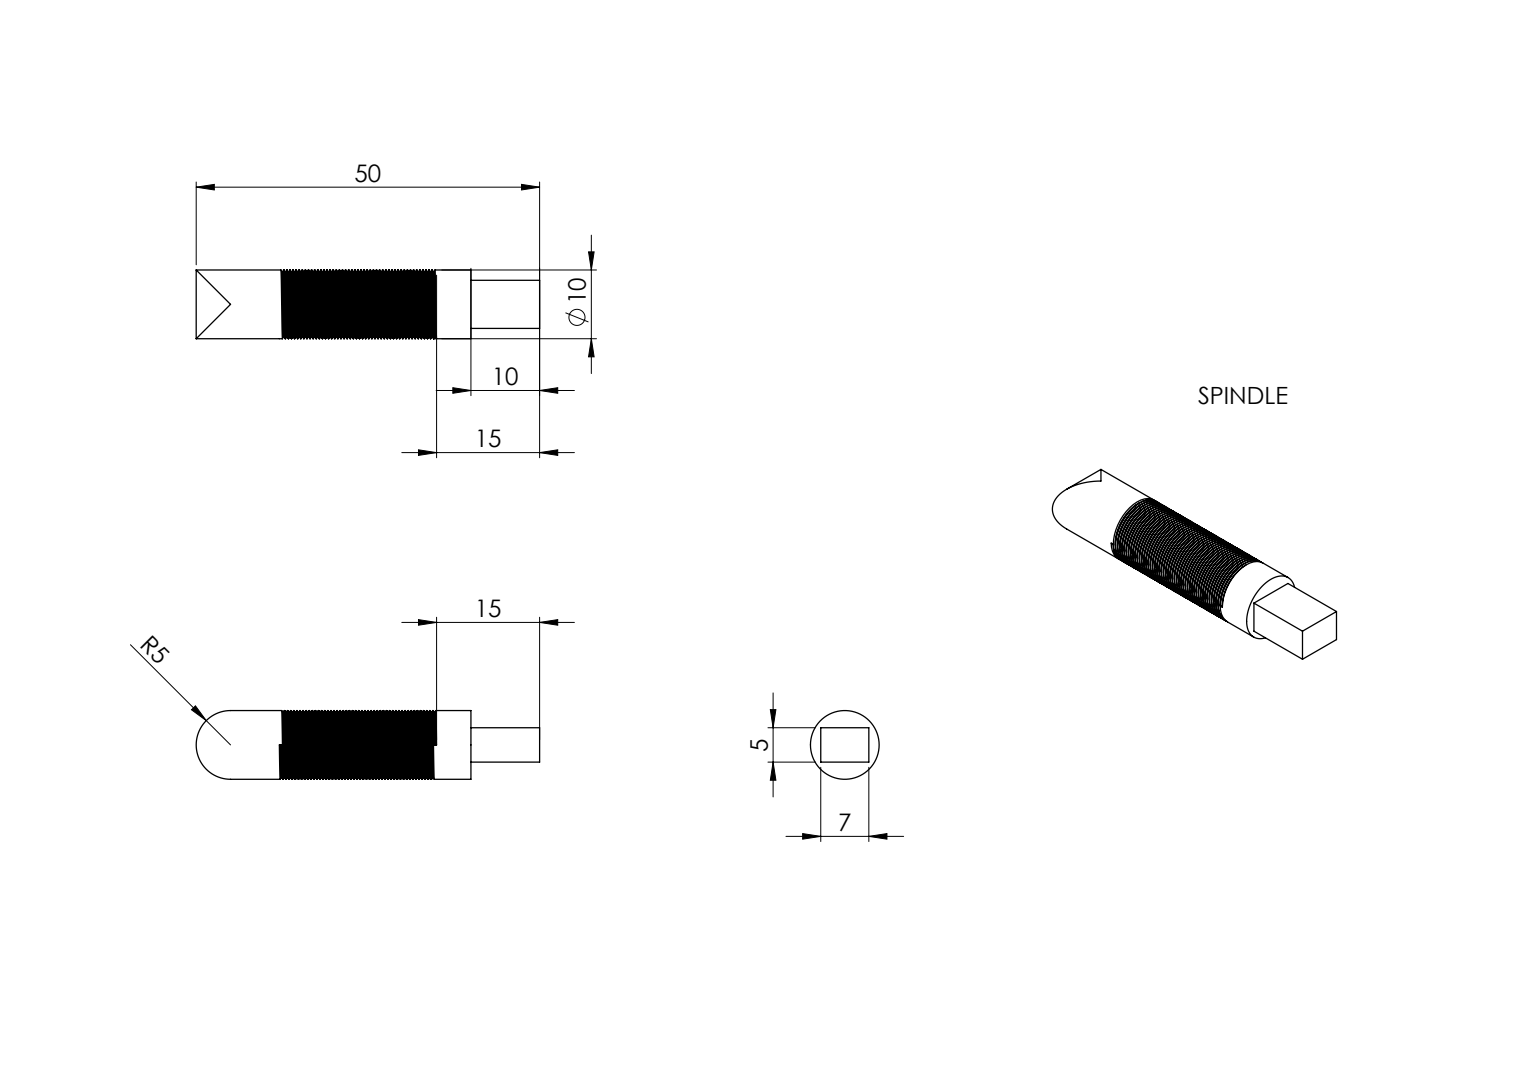
ISO-10303-21;
HEADER;
FILE_DESCRIPTION (('STEP AP214'),
    '1' );
FILE_NAME ('spindle.step',
    '2026-10-26T05:42:23',
    ( '' ),
    ( '' ),
    'SwSTEP 2.0',
    'SolidWorks 2026',
    '' );
FILE_SCHEMA (( 'AUTOMOTIVE_DESIGN' ));
ENDSEC;

DATA;
#7=CARTESIAN_POINT ( 'NONE',  ( 45.00000000000000000, 0.000000000000000000, 0.000000000000000000 ) ) ;
#9=CARTESIAN_POINT ( 'NONE',  ( 19.58437500061451786, -2.746126346562642428, -4.756430356249999214 ) ) ;
#12=CARTESIAN_POINT ( 'NONE',  ( 15.13125000122903252, 4.330127018922191873, 2.499999999999999556 ) ) ;
#27=CARTESIAN_POINT ( 'NONE',  ( 7.396875000614516082, -4.119189519843965641, -2.378215178125001383 ) ) ;
#49=CARTESIAN_POINT ( 'NONE',  ( 13.88437500061451679, 5.824947211148865298E-16, -4.756430356249998326 ) ) ;
#74=EDGE_CURVE ( 'NONE', #45106, #54880, #1431, .T. ) ;
#80=CARTESIAN_POINT ( 'NONE',  ( 19.88437500061451857, 4.119189519843966529, 2.378215178124999607 ) ) ;
#85=CARTESIAN_POINT ( 'NONE',  ( 19.46249999999999858, 2.886751345948129099, -4.999999999999998224 ) ) ;
#89=CARTESIAN_POINT ( 'NONE',  ( 24.45937500061451786, -5.492252693125287522, -1.008910452111647106E-15 ) ) ;
#95=CARTESIAN_POINT ( 'NONE',  ( 27.64687500061451431, -4.119189519843965641, -2.378215178125001383 ) ) ;
#97=CARTESIAN_POINT ( 'NONE',  ( 11.07187500061451679, 5.824947211148865298E-16, -4.756430356249998326 ) ) ;
#104=( BOUNDED_CURVE ( )  B_SPLINE_CURVE ( 2, ( #27084, #21157, #20050, #59212, #14521, #42242, #3825 ),
 .UNSPECIFIED., .F., .F. ) 
 B_SPLINE_CURVE_WITH_KNOTS ( ( 3, 2, 2, 3 ),
 ( 0.5700000000000000622, 0.5733333333333334725, 0.5766666666666667718, 0.5800000000000000711 ),
 .UNSPECIFIED. ) 
 CURVE ( )  GEOMETRIC_REPRESENTATION_ITEM ( )  RATIONAL_B_SPLINE_CURVE ( ( 0.9999999999999955591, 0.8660254037844431485, 1.000000000000000000, 0.8660254037844387076, 1.000000000000000000, 0.8660254037844342667, 1.000000000000004441 ) ) 
 REPRESENTATION_ITEM ( '' )  );
#108=CARTESIAN_POINT ( 'NONE',  ( 18.67500000000000071, 4.330127018922191873, 2.499999999999999556 ) ) ;
#123=ORIENTED_EDGE ( 'NONE', *, *, #29254, .F. ) ;
#133=CARTESIAN_POINT ( 'NONE',  ( 22.35937500061451644, -4.119189519843965641, -2.378215178125001383 ) ) ;
#139=ORIENTED_EDGE ( 'NONE', *, *, #5292, .F. ) ;
#151=CARTESIAN_POINT ( 'NONE',  ( 17.30625000122903145, 4.330127018922192761, -2.499999999999997780 ) ) ;
#163=EDGE_CURVE ( 'NONE', #39643, #7983, #64627, .T. ) ;
#168=CARTESIAN_POINT ( 'NONE',  ( 26.67187500061451644, 2.746126346562643317, 4.756430356249998326 ) ) ;
#173=CARTESIAN_POINT ( 'NONE',  ( 26.25000000000000000, 4.330127018922192761, -2.499999999999997780 ) ) ;
#181=CARTESIAN_POINT ( 'NONE',  ( 11.11875000122903323, 2.886751345948126879, 4.999999999999999112 ) ) ;
#182=CARTESIAN_POINT ( 'NONE',  ( 13.19999999999999929, 4.330127018922192761, -2.499999999999997780 ) ) ;
#185=CARTESIAN_POINT ( 'NONE',  ( 21.27187500061451431, -4.119189519843968306, 2.378215178124996054 ) ) ;
#192=CARTESIAN_POINT ( 'NONE',  ( 10.74375000122903323, -2.886751345948130876, 4.999999999999996447 ) ) ;
#196=CARTESIAN_POINT ( 'NONE',  ( 13.05937500061451573, 2.746126346562643317, 4.756430356249998326 ) ) ;
#203=LINE ( 'NONE', #67793, #8872 ) ;
#217=CARTESIAN_POINT ( 'NONE',  ( 13.57500000000000107, 6.123233995736764310E-16, -4.999999999999998224 ) ) ;
#219=CARTESIAN_POINT ( 'NONE',  ( 29.29687500061451644, 0.000000000000000000, 4.756430356249998326 ) ) ;
#220=CARTESIAN_POINT ( 'NONE',  ( 12.38437500061451857, -4.119189519843968306, 2.378215178124996054 ) ) ;
#237=CARTESIAN_POINT ( 'NONE',  ( 23.26875000122903003, 2.886751345948126879, 4.999999999999999112 ) ) ;
#282=CARTESIAN_POINT ( 'NONE',  ( 17.89687500061451431, 4.119189519843966529, -2.378215178124998275 ) ) ;
#297=CARTESIAN_POINT ( 'NONE',  ( 18.22499999999999787, 4.330127018922191873, 2.499999999999999556 ) ) ;
#298=CARTESIAN_POINT ( 'NONE',  ( 19.05937500061451928, 0.000000000000000000, 4.756430356249998326 ) ) ;
#308=EDGE_LOOP ( 'NONE', ( #45837, #56679, #50706, #57678 ) ) ;
#339=AXIS2_PLACEMENT_3D ( 'NONE', #22340, #45247, #39713 ) ;
#342=CARTESIAN_POINT ( 'NONE',  ( 9.946875000614516793, 5.492252693125287522, 3.363034840372157021E-16 ) ) ;
#360=CARTESIAN_POINT ( 'NONE',  ( 18.38437500061451502, 5.492252693125287522, 3.363034840372157021E-16 ) ) ;
#363=CARTESIAN_POINT ( 'NONE',  ( 26.67187500061451289, -4.119189519843968306, 2.378215178124996054 ) ) ;
#371=FACE_OUTER_BOUND ( 'NONE', #14066, .T. ) ;
#377=CARTESIAN_POINT ( 'NONE',  ( 7.696875000614517681, 0.000000000000000000, 4.756430356249998326 ) ) ;
#384=CARTESIAN_POINT ( 'NONE',  ( 24.84375000122903288, -2.886751345948153968, -4.999999999999952038 ) ) ;
#386=CARTESIAN_POINT ( 'NONE',  ( 11.38125000122903252, 6.123233995736764310E-16, -4.999999999999998224 ) ) ;
#399=CARTESIAN_POINT ( 'NONE',  ( 15.08437500061451786, -4.119189519843968306, 2.378215178124996054 ) ) ;
#430=CARTESIAN_POINT ( 'NONE',  ( 17.37187500061451573, -5.492252693125287522, -1.008910452111647106E-15 ) ) ;
#432=CARTESIAN_POINT ( 'NONE',  ( 14.53125000122903288, 6.123233995736764310E-16, -4.999999999999998224 ) ) ;
#437=CARTESIAN_POINT ( 'NONE',  ( 18.67500000000000071, 4.330127018922191873, 2.499999999999999556 ) ) ;
#441=CARTESIAN_POINT ( 'NONE',  ( 26.14687500061451431, 0.000000000000000000, 4.756430356249998326 ) ) ;
#442=CARTESIAN_POINT ( 'NONE',  ( 18.39375000122902648, -2.886751345948074920, 5.000000000000092371 ) ) ;
#449=CARTESIAN_POINT ( 'NONE',  ( 25.02187500061451431, 5.824947211148865298E-16, -4.756430356249998326 ) ) ;
#451=CARTESIAN_POINT ( 'NONE',  ( 11.10937500061451644, 2.746126346562645981, -4.756430356249997438 ) ) ;
#454=ORIENTED_EDGE ( 'NONE', *, *, #66600, .F. ) ;
#456=CARTESIAN_POINT ( 'NONE',  ( 45.00000000000000000, 6.123233995736764310E-16, -4.999999999999998224 ) ) ;
#457=CARTESIAN_POINT ( 'NONE',  ( 17.00625000122903074, 0.000000000000000000, 4.999999999999998224 ) ) ;
#461=CYLINDRICAL_SURFACE ( 'NONE', #51393, 4.999999999999998224 ) ;
#465=CARTESIAN_POINT ( 'NONE',  ( 13.69687500061451679, -4.119189519843965641, -2.378215178125001383 ) ) ;
#475=CARTESIAN_POINT ( 'NONE',  ( 18.86249999999999716, -5.773502691896255534, -1.060575238724906372E-15 ) ) ;
#485=CARTESIAN_POINT ( 'NONE',  ( 21.53437500061451715, 5.824947211148865298E-16, -4.756430356249998326 ) ) ;
#489=( BOUNDED_CURVE ( )  B_SPLINE_CURVE ( 2, ( #20921, #14646, #9118, #48647, #21286, #33107, #71172 ),
 .UNSPECIFIED., .F., .F. ) 
 B_SPLINE_CURVE_WITH_KNOTS ( ( 3, 2, 2, 3 ),
 ( 0.3500000000000000888, 0.3533333333333333881, 0.3566666666666667429, 0.3599999999999999867 ),
 .UNSPECIFIED. ) 
 CURVE ( )  GEOMETRIC_REPRESENTATION_ITEM ( )  RATIONAL_B_SPLINE_CURVE ( ( 0.9999999999999955591, 0.8660254037844431485, 1.000000000000000000, 0.8660254037844387076, 1.000000000000000000, 0.8660254037844387076, 1.000000000000000000 ) ) 
 REPRESENTATION_ITEM ( '' )  );
#507=CARTESIAN_POINT ( 'NONE',  ( 16.66875000122903216, -5.773502691896255534, -1.060575238724906372E-15 ) ) ;
#509=CARTESIAN_POINT ( 'NONE',  ( 29.67656250092177217, 0.000000000000000000, 4.878215178124998275 ) ) ;
#523=CARTESIAN_POINT ( 'NONE',  ( 25.32187500061451857, 2.746126346562643317, 4.756430356249998326 ) ) ;
#528=CARTESIAN_POINT ( 'NONE',  ( 26.17500000000000071, 6.123233995736764310E-16, -4.999999999999998224 ) ) ;
#538=CARTESIAN_POINT ( 'NONE',  ( 9.431250001229033231, -4.330127018922194537, 2.499999999999995559 ) ) ;
#542=CARTESIAN_POINT ( 'NONE',  ( 18.87187500061451573, 4.119189519843966529, 2.378215178124999607 ) ) ;
#555=CARTESIAN_POINT ( 'NONE',  ( 13.13437500061451679, -2.746126346562646425, 4.756430356249996549 ) ) ;
#579=CARTESIAN_POINT ( 'NONE',  ( 28.88437500061451502, 4.119189519843966529, 2.378215178124999607 ) ) ;
#583=CARTESIAN_POINT ( 'NONE',  ( 11.67187500061451821, 2.746126346562645981, -4.756430356249997438 ) ) ;
#593=( BOUNDED_CURVE ( )  B_SPLINE_CURVE ( 2, ( #12661, #29655, #35196, #35914, #62904, #56997, #24104 ),
 .UNSPECIFIED., .F., .F. ) 
 B_SPLINE_CURVE_WITH_KNOTS ( ( 3, 2, 2, 3 ),
 ( 0.8600000000000002087, 0.8633333333333333970, 0.8666666666666668073, 0.8699999999999999956 ),
 .UNSPECIFIED. ) 
 CURVE ( )  GEOMETRIC_REPRESENTATION_ITEM ( )  RATIONAL_B_SPLINE_CURVE ( ( 0.9999999999999911182, 0.8660254037844475894, 1.000000000000000000, 0.8660254037844387076, 1.000000000000000000, 0.8660254037844387076, 1.000000000000000000 ) ) 
 REPRESENTATION_ITEM ( '' )  );
#600=CARTESIAN_POINT ( 'NONE',  ( 22.36875000122903145, 2.886751345948126879, 4.999999999999999112 ) ) ;
#607=CARTESIAN_POINT ( 'NONE',  ( 25.55625000122903501, 0.000000000000000000, 4.999999999999998224 ) ) ;
#647=CARTESIAN_POINT ( 'NONE',  ( 18.12187500061451928, -4.119189519843968306, 2.378215178124996054 ) ) ;
#662=CARTESIAN_POINT ( 'NONE',  ( 22.12500000000000000, 6.123233995736764310E-16, -4.999999999999998224 ) ) ;
#663=CARTESIAN_POINT ( 'NONE',  ( 20.85937500061451644, 0.000000000000000000, 4.756430356249998326 ) ) ;
#675=VERTEX_POINT ( 'NONE', #2077 ) ;
#706=AXIS2_PLACEMENT_3D ( 'NONE', #6791, #31874, #14139 ) ;
#707=CARTESIAN_POINT ( 'NONE',  ( 9.834375000614517859, 5.824947211148865298E-16, -4.756430356249998326 ) ) ;
#729=CARTESIAN_POINT ( 'NONE',  ( 18.23437500061451644, -2.746126346562642428, -4.756430356249999214 ) ) ;
#732=CARTESIAN_POINT ( 'NONE',  ( 24.98437500061451289, -2.746126346562642428, -4.756430356249999214 ) ) ;
#736=CARTESIAN_POINT ( 'NONE',  ( 28.72500000000000142, -4.330127018922194537, 2.499999999999995559 ) ) ;
#746=CARTESIAN_POINT ( 'NONE',  ( 26.14687500061451431, 5.492252693125287522, 3.363034840372157021E-16 ) ) ;
#765=CARTESIAN_POINT ( 'NONE',  ( 15.19687500061451679, -2.746126346562641984, -4.756430356249999214 ) ) ;
#780=ORIENTED_EDGE ( 'NONE', *, *, #27131, .T. ) ;
#797=CARTESIAN_POINT ( 'NONE',  ( 17.29687500061451999, -2.746126346562646425, 4.756430356249996549 ) ) ;
#805=CARTESIAN_POINT ( 'NONE',  ( 16.35000000000000142, 4.330127018922192761, -2.499999999999997780 ) ) ;
#809=CARTESIAN_POINT ( 'NONE',  ( 26.52187500061451431, 4.119189519843966529, 2.378215178124999607 ) ) ;
#816=CARTESIAN_POINT ( 'NONE',  ( 23.85937500061451644, 2.746126346562643317, 4.756430356249998326 ) ) ;
#818=CARTESIAN_POINT ( 'NONE',  ( 10.32187500061451679, 4.119189519843966529, 2.378215178124999607 ) ) ;
#821=ORIENTED_EDGE ( 'NONE', *, *, #39594, .T. ) ;
#823=CARTESIAN_POINT ( 'NONE',  ( 16.72500000000000142, 6.123233995736764310E-16, -4.999999999999998224 ) ) ;
#827=CARTESIAN_POINT ( 'NONE',  ( 29.55000000000000071, 0.000000000000000000, 4.999999999999998224 ) ) ;
#829=VERTEX_POINT ( 'NONE', #12152 ) ;
#831=CARTESIAN_POINT ( 'NONE',  ( 11.82187500061451502, -4.119189519843968306, 2.378215178124996054 ) ) ;
#851=VECTOR ( 'NONE', #69149, 1000.000000000000000 ) ;
#853=CARTESIAN_POINT ( 'NONE',  ( 21.38437500061451502, -4.119189519843968306, 2.378215178124996054 ) ) ;
#865=CARTESIAN_POINT ( 'NONE',  ( 15.05625000122903323, 4.330127018922192761, -2.499999999999997780 ) ) ;
#873=CARTESIAN_POINT ( 'NONE',  ( 16.59375000122903288, -2.886751345948129988, 4.999999999999997335 ) ) ;
#889=CARTESIAN_POINT ( 'NONE',  ( 24.60937500061451644, -4.119189519843965641, -2.378215178125001383 ) ) ;
#893=EDGE_CURVE ( 'NONE', #53197, #52280, #67237, .T. ) ;
#895=CARTESIAN_POINT ( 'NONE',  ( 23.96249999999999858, 2.886751345948129099, -4.999999999999998224 ) ) ;
#902=CARTESIAN_POINT ( 'NONE',  ( 22.96875000122903288, -5.773502691896255534, -1.060575238724906372E-15 ) ) ;
#904=CARTESIAN_POINT ( 'NONE',  ( 9.993750001229033231, -2.886751345948125991, -5.000000000000000000 ) ) ;
#905=CARTESIAN_POINT ( 'NONE',  ( 9.037499999999997868, -2.886751345948181946, -4.999999999999904077 ) ) ;
#908=CARTESIAN_POINT ( 'NONE',  ( 19.39687500061451786, 0.000000000000000000, 4.756430356249998326 ) ) ;
#911=ORIENTED_EDGE ( 'NONE', *, *, #71191, .F. ) ;
#912=CARTESIAN_POINT ( 'NONE',  ( 27.52500000000000213, 6.123233995736764310E-16, -4.999999999999998224 ) ) ;
#919=CARTESIAN_POINT ( 'NONE',  ( 10.20937500061451608, 2.746126346562645981, -4.756430356249997438 ) ) ;
#922=( BOUNDED_CURVE ( )  B_SPLINE_CURVE ( 2, ( #607, #7219, #22752, #18276, #6498, #23113, #45303 ),
 .UNSPECIFIED., .F., .F. ) 
 B_SPLINE_CURVE_WITH_KNOTS ( ( 3, 2, 2, 3 ),
 ( 0.1799999999999999378, 0.1833333333333333204, 0.1866666666666667029, 0.1900000000000000855 ),
 .UNSPECIFIED. ) 
 CURVE ( )  GEOMETRIC_REPRESENTATION_ITEM ( )  RATIONAL_B_SPLINE_CURVE ( ( 1.000000000000002220, 0.8660254037844364872, 1.000000000000000000, 0.8660254037844387076, 1.000000000000000000, 0.8660254037844353769, 1.000000000000003331 ) ) 
 REPRESENTATION_ITEM ( '' )  );
#938=ADVANCED_FACE ( 'NONE', ( #56138 ), #34679, .T. ) ;
#942=CARTESIAN_POINT ( 'NONE',  ( 28.54687500061451644, -2.746126346562646425, 4.756430356249996549 ) ) ;
#945=CARTESIAN_POINT ( 'NONE',  ( 27.64687500061451431, -4.119189519843965641, -2.378215178125001383 ) ) ;
#946=CARTESIAN_POINT ( 'NONE',  ( 12.45937500061451786, -4.119189519843965641, -2.378215178125001383 ) ) ;
#961=CARTESIAN_POINT ( 'NONE',  ( 22.51875000122903003, -5.773502691896255534, -1.060575238724906372E-15 ) ) ;
#987=FACE_OUTER_BOUND ( 'NONE', #13837, .T. ) ;
#996=CARTESIAN_POINT ( 'NONE',  ( 19.14375000122903003, 5.773502691896255534, 3.535250795749688401E-16 ) ) ;
#1007=ORIENTED_EDGE ( 'NONE', *, *, #23321, .F. ) ;
#1010=CARTESIAN_POINT ( 'NONE',  ( 19.80937500061451217, 2.746126346562643317, 4.756430356249998326 ) ) ;
#1012=( BOUNDED_CURVE ( )  B_SPLINE_CURVE ( 2, ( #8240, #47399, #2701, #60291, #65115, #64749, #48503 ),
 .UNSPECIFIED., .F., .F. ) 
 B_SPLINE_CURVE_WITH_KNOTS ( ( 3, 2, 2, 3 ),
 ( 0.4799999999999999267, 0.4833333333333333370, 0.4866666666666667473, 0.4900000000000001021 ),
 .UNSPECIFIED. ) 
 CURVE ( )  GEOMETRIC_REPRESENTATION_ITEM ( )  RATIONAL_B_SPLINE_CURVE ( ( 1.000000000000002220, 0.8660254037844364872, 1.000000000000000000, 0.8660254037844387076, 1.000000000000000000, 0.8660254037844342667, 1.000000000000004441 ) ) 
 REPRESENTATION_ITEM ( '' )  );
#1027=CARTESIAN_POINT ( 'NONE',  ( 22.19999999999999574, 4.330127018922192761, -2.499999999999997780 ) ) ;
#1028=CARTESIAN_POINT ( 'NONE',  ( 20.40937500061451715, 0.000000000000000000, 4.756430356249998326 ) ) ;
#1045=CARTESIAN_POINT ( 'NONE',  ( 29.60625000122903216, 0.000000000000000000, 4.999999999999998224 ) ) ;
#1049=CARTESIAN_POINT ( 'NONE',  ( 8.521875000614517859, 2.746126346562645981, -4.756430356249997438 ) ) ;
#1055=EDGE_CURVE ( 'NONE', #42390, #54979, #24487, .T. ) ;
#1067=EDGE_CURVE ( 'NONE', #56470, #45665, #34410, .T. ) ;
#1074=CARTESIAN_POINT ( 'NONE',  ( 8.709375000614517859, 0.000000000000000000, 4.756430356249998326 ) ) ;
#1083=CARTESIAN_POINT ( 'NONE',  ( 23.98125000122903216, 6.123233995736764310E-16, -4.999999999999998224 ) ) ;
#1094=CARTESIAN_POINT ( 'NONE',  ( 16.77187500061451431, -4.119189519843968306, 2.378215178124996054 ) ) ;
#1097=CARTESIAN_POINT ( 'NONE',  ( 27.27187500061451786, 5.824947211148865298E-16, -4.756430356249998326 ) ) ;
#1101=DIRECTION ( 'NONE',  ( -1.000000000000000000, -0.000000000000000000, -0.000000000000000000 ) ) ;
#1104=CARTESIAN_POINT ( 'NONE',  ( 28.25625000122903074, 0.000000000000000000, 4.999999999999998224 ) ) ;
#1105=CARTESIAN_POINT ( 'NONE',  ( 45.00000000000000000, 0.000000000000000000, 0.000000000000000000 ) ) ;
#1111=CARTESIAN_POINT ( 'NONE',  ( 27.60937500061451644, 0.000000000000000000, 4.756430356249998326 ) ) ;
#1128=CARTESIAN_POINT ( 'NONE',  ( 15.42187500061451821, 2.746126346562643317, 4.756430356249998326 ) ) ;
#1145=EDGE_CURVE ( 'NONE', #65176, #58120, #30504, .T. ) ;
#1155=EDGE_LOOP ( 'NONE', ( #2010, #4569, #25849, #38019 ) ) ;
#1159=CARTESIAN_POINT ( 'NONE',  ( 17.48437500061451999, 5.824947211148865298E-16, -4.756430356249998326 ) ) ;
#1165=CARTESIAN_POINT ( 'NONE',  ( 17.02499999999999858, -4.330127018922194537, 2.499999999999995559 ) ) ;
#1168=DIRECTION ( 'NONE',  ( -1.000000000000000000, -0.000000000000000000, -0.000000000000000000 ) ) ;
#1169=CARTESIAN_POINT ( 'NONE',  ( 24.08437500061451786, -2.746126346562641984, -4.756430356249999214 ) ) ;
#1172=DIRECTION ( 'NONE',  ( 0.000000000000000000, -0.000000000000000000, -1.000000000000000000 ) ) ;
#1176=CARTESIAN_POINT ( 'NONE',  ( 25.77187500061451431, -4.119189519843968306, 2.378215178124996054 ) ) ;
#1178=CARTESIAN_POINT ( 'NONE',  ( 11.40937500061451537, -5.492252693125287522, -1.008910452111647106E-15 ) ) ;
#1186=CARTESIAN_POINT ( 'NONE',  ( 19.31250000000000000, -5.773502691896255534, -1.060575238724906372E-15 ) ) ;
#1187=FACE_OUTER_BOUND ( 'NONE', #70804, .T. ) ;
#1188=ORIENTED_EDGE ( 'NONE', *, *, #50906, .T. ) ;
#1190=CARTESIAN_POINT ( 'NONE',  ( 10.88437500061451679, -2.746126346562646425, 4.756430356249996549 ) ) ;
#1203=ORIENTED_EDGE ( 'NONE', *, *, #11547, .T. ) ;
#1211=CARTESIAN_POINT ( 'NONE',  ( 22.62187500061451573, 2.746126346562643317, 4.756430356249998326 ) ) ;
#1228=CARTESIAN_POINT ( 'NONE',  ( 28.61250000000000071, 2.886751345948148195, 4.999999999999962697 ) ) ;
#1231=CARTESIAN_POINT ( 'NONE',  ( 17.41875000122903216, 2.886751345948126879, 4.999999999999999112 ) ) ;
#1248=CARTESIAN_POINT ( 'NONE',  ( 23.48437500061451644, 4.119189519843966529, 2.378215178124999607 ) ) ;
#1254=CARTESIAN_POINT ( 'NONE',  ( 25.08749999999999858, -2.886751345948129988, 4.999999999999997335 ) ) ;
#1258=CARTESIAN_POINT ( 'NONE',  ( 24.41250000000000142, 2.886751345948142866, -4.999999999999973355 ) ) ;
#1262=CARTESIAN_POINT ( 'NONE',  ( 8.493750001229033231, -2.886751345948129988, 4.999999999999997335 ) ) ;
#1265=CARTESIAN_POINT ( 'NONE',  ( 17.74687500061451928, -4.119189519843965641, -2.378215178125001383 ) ) ;
#1274=CARTESIAN_POINT ( 'NONE',  ( 16.55625000122903145, 0.000000000000000000, 4.999999999999998224 ) ) ;
#1275=CARTESIAN_POINT ( 'NONE',  ( 11.03437500061451360, -2.746126346562642428, -4.756430356249999214 ) ) ;
#1288=CARTESIAN_POINT ( 'NONE',  ( 9.637499999999999289, 5.773502691896255534, 3.535250795749688894E-16 ) ) ;
#1297=CARTESIAN_POINT ( 'NONE',  ( 29.55937500061451573, -4.119189519843965641, -2.378215178125001383 ) ) ;
#1299=CARTESIAN_POINT ( 'NONE',  ( 28.65937500061451715, 2.746126346562645981, -4.756430356249997438 ) ) ;
#1300=CARTESIAN_POINT ( 'NONE',  ( 13.69687500061451679, -2.746126346562646425, 4.756430356249996549 ) ) ;
#1308=DIRECTION ( 'NONE',  ( -1.000000000000000000, -0.000000000000000000, -0.000000000000000000 ) ) ;
#1317=CARTESIAN_POINT ( 'NONE',  ( 22.93125000122903145, -4.330127018922194537, 2.499999999999995559 ) ) ;
#1342=DIRECTION ( 'NONE',  ( 0.000000000000000000, 0.000000000000000000, -1.000000000000000000 ) ) ;
#1343=ADVANCED_FACE ( 'NONE', ( #50096 ), #44567, .T. ) ;
#1345=ADVANCED_FACE ( 'NONE', ( #26702 ), #38510, .T. ) ;
#1353=CARTESIAN_POINT ( 'NONE',  ( 19.10625000122903216, 4.330127018922192761, -2.499999999999997780 ) ) ;
#1361=CARTESIAN_POINT ( 'NONE',  ( 11.10000000000000142, 0.000000000000000000, 4.999999999999998224 ) ) ;
#1370=CARTESIAN_POINT ( 'NONE',  ( 18.27187500061451431, 5.824947211148865298E-16, -4.756430356249998326 ) ) ;
#1379=ORIENTED_EDGE ( 'NONE', *, *, #49066, .T. ) ;
#1386=( GEOMETRIC_REPRESENTATION_CONTEXT ( 3 ) GLOBAL_UNCERTAINTY_ASSIGNED_CONTEXT ( ( #63913 ) ) GLOBAL_UNIT_ASSIGNED_CONTEXT ( ( #46737, #57797, #30097 ) ) REPRESENTATION_CONTEXT ( 'NONE', 'WORKASPACE' ) );
#1387=CARTESIAN_POINT ( 'NONE',  ( 22.31250000000000000, 2.886751345948154857, 4.999999999999951150 ) ) ;
#1388=CARTESIAN_POINT ( 'NONE',  ( 20.67187500061451289, 2.746126346562645981, -4.756430356249997438 ) ) ;
#1411=DIRECTION ( 'NONE',  ( -1.000000000000000000, -0.000000000000000000, -0.000000000000000000 ) ) ;
#1431=( BOUNDED_CURVE ( )  B_SPLINE_CURVE ( 2, ( #52853, #2977, #53211, #8514, #2607, #25129, #47670 ),
 .UNSPECIFIED., .F., .T. ) 
 B_SPLINE_CURVE_WITH_KNOTS ( ( 3, 2, 2, 3 ),
 ( 0.6300000000000001155, 0.6333333333333334147, 0.6366666666666668251, 0.6400000000000001243 ),
 .UNSPECIFIED. ) 
 CURVE ( )  GEOMETRIC_REPRESENTATION_ITEM ( )  RATIONAL_B_SPLINE_CURVE ( ( 0.9999999999999955591, 0.8660254037844431485, 1.000000000000000000, 0.8660254037844387076, 1.000000000000000000, 0.8660254037844342667, 1.000000000000004441 ) ) 
 REPRESENTATION_ITEM ( '' )  );
#1434=CARTESIAN_POINT ( 'NONE',  ( 8.934375000614517504, 5.824947211148865298E-16, -4.756430356249998326 ) ) ;
#1440=EDGE_CURVE ( 'NONE', #59687, #30573, #41969, .T. ) ;
#1455=CARTESIAN_POINT ( 'NONE',  ( 17.85937500061451644, 2.746126346562645981, -4.756430356249997438 ) ) ;
#1458=CARTESIAN_POINT ( 'NONE',  ( 26.29687500061451644, -4.119189519843965641, -2.378215178125001383 ) ) ;
#1473=CARTESIAN_POINT ( 'NONE',  ( 27.83437500061451786, 5.824947211148865298E-16, -4.756430356249998326 ) ) ;
#1482=VERTEX_POINT ( 'NONE', #21504 ) ;
#1492=CARTESIAN_POINT ( 'NONE',  ( 14.59687500061452070, -2.746126346562646425, 4.756430356249996549 ) ) ;
#1518=VERTEX_POINT ( 'NONE', #4538 ) ;
#1522=CARTESIAN_POINT ( 'NONE',  ( 15.64687500061451608, -2.746126346562642428, -4.756430356249999214 ) ) ;
#1528=CARTESIAN_POINT ( 'NONE',  ( 18.26249999999999929, 2.886751345948126879, 4.999999999999999112 ) ) ;
#1531=CARTESIAN_POINT ( 'NONE',  ( 45.00000000000000000, 6.123233995736764310E-16, -4.999999999999998224 ) ) ;
#1532=CARTESIAN_POINT ( 'NONE',  ( 24.38437500061451502, -2.746126346562646425, 4.756430356249996549 ) ) ;
#1535=CARTESIAN_POINT ( 'NONE',  ( 45.00000000000000000, 0.000000000000000000, 4.999999999999998224 ) ) ;
#1539=CARTESIAN_POINT ( 'NONE',  ( 25.47187500061451360, 5.824947211148865298E-16, -4.756430356249998326 ) ) ;
#1541=CARTESIAN_POINT ( 'NONE',  ( 10.50937500061451502, -5.492252693125287522, -1.008910452111647106E-15 ) ) ;
#1546=DIRECTION ( 'NONE',  ( 0.000000000000000000, 0.000000000000000000, 1.000000000000000000 ) ) ;
#1550=CARTESIAN_POINT ( 'NONE',  ( 12.28125000122903110, 6.123233995736764310E-16, -4.999999999999998224 ) ) ;
#1553=CARTESIAN_POINT ( 'NONE',  ( 12.19687500061451502, 0.000000000000000000, 4.756430356249998326 ) ) ;
#1565=VERTEX_POINT ( 'NONE', #65849 ) ;
#1573=CARTESIAN_POINT ( 'NONE',  ( 21.83437500061451786, -4.119189519843968306, 2.378215178124996054 ) ) ;
#1580=VERTEX_POINT ( 'NONE', #26328 ) ;
#1590=CARTESIAN_POINT ( 'NONE',  ( 21.41250000000000142, 2.886751345948126879, 4.999999999999998224 ) ) ;
#1607=CARTESIAN_POINT ( 'NONE',  ( 24.30937500061451573, 4.119189519843966529, -2.378215178124998275 ) ) ;
#1611=EDGE_CURVE ( 'NONE', #33907, #61284, #66577, .T. ) ;
#1614=CARTESIAN_POINT ( 'NONE',  ( 25.05000000000000071, 0.000000000000000000, 4.999999999999998224 ) ) ;
#1618=DIRECTION ( 'NONE',  ( 0.000000000000000000, 1.000000000000000000, -8.673617379884037937E-17 ) ) ;
#1624=CARTESIAN_POINT ( 'NONE',  ( 15.29999999999999893, -4.330127018922190985, -2.500000000000001332 ) ) ;
#1626=CARTESIAN_POINT ( 'NONE',  ( 8.381250001229034297, 4.330127018922191873, 2.499999999999999556 ) ) ;
#1629=CARTESIAN_POINT ( 'NONE',  ( 17.48437500061451644, 5.492252693125287522, 3.363034840372157021E-16 ) ) ;
#1636=EDGE_CURVE ( 'NONE', #53798, #61419, #18855, .T. ) ;
#1641=CARTESIAN_POINT ( 'NONE',  ( 9.984375000614516438, -2.746126346562646425, 4.756430356249996549 ) ) ;
#1642=ORIENTED_EDGE ( 'NONE', *, *, #4558, .T. ) ;
#1649=CARTESIAN_POINT ( 'NONE',  ( 28.48125000122902861, 6.123233995736764310E-16, -4.999999999999998224 ) ) ;
#1653=CARTESIAN_POINT ( 'NONE',  ( 10.01250000000000107, 2.886751345948129099, -4.999999999999998224 ) ) ;
#1656=VERTEX_POINT ( 'NONE', #44433 ) ;
#1663=CARTESIAN_POINT ( 'NONE',  ( 26.97187500061451360, 4.119189519843966529, 2.378215178124999607 ) ) ;
#1664=CARTESIAN_POINT ( 'NONE',  ( 13.84687500061451537, -2.746126346562642428, -4.756430356249999214 ) ) ;
#1679=CARTESIAN_POINT ( 'NONE',  ( 23.75625000122903074, 0.000000000000000000, 4.999999999999998224 ) ) ;
#1702=CARTESIAN_POINT ( 'NONE',  ( 25.42500000000000071, 4.330127018922191873, 2.499999999999999556 ) ) ;
#1717=CARTESIAN_POINT ( 'NONE',  ( 45.00000000000000000, 0.000000000000000000, 0.000000000000000000 ) ) ;
#1724=VERTEX_POINT ( 'NONE', #60289 ) ;
#1730=CARTESIAN_POINT ( 'NONE',  ( 19.43437500061451573, -2.746126346562646425, 4.756430356249996549 ) ) ;
#1743=EDGE_CURVE ( 'NONE', #59457, #65810, #46732, .T. ) ;
#1749=CARTESIAN_POINT ( 'NONE',  ( 19.39687500061451786, 5.492252693125287522, 3.363034840372157021E-16 ) ) ;
#1773=CARTESIAN_POINT ( 'NONE',  ( 7.500000000000000000, 0.000000000000000000, 4.999999999999998224 ) ) ;
#1784=VERTEX_POINT ( 'NONE', #29238 ) ;
#1785=VECTOR ( 'NONE', #34589, 1000.000000000000000 ) ;
#1797=CARTESIAN_POINT ( 'NONE',  ( 27.88125000122903074, -4.330127018922194537, 2.499999999999995559 ) ) ;
#1798=CARTESIAN_POINT ( 'NONE',  ( 9.534375000614517148, 4.119189519843966529, 2.378215178124999607 ) ) ;
#1808=DIRECTION ( 'NONE',  ( -1.000000000000000000, -0.000000000000000000, -0.000000000000000000 ) ) ;
#1809=VECTOR ( 'NONE', #70709, 1000.000000000000000 ) ;
#1818=CARTESIAN_POINT ( 'NONE',  ( 14.48437500061451644, -2.746126346562646425, 4.756430356249996549 ) ) ;
#1821=CARTESIAN_POINT ( 'NONE',  ( 25.20937500061451431, 2.746126346562643317, 4.756430356249998326 ) ) ;
#1836=CARTESIAN_POINT ( 'NONE',  ( 27.30937500061451573, -4.119189519843965641, -2.378215178125001383 ) ) ;
#1846=VERTEX_POINT ( 'NONE', #34042 ) ;
#1856=CARTESIAN_POINT ( 'NONE',  ( 11.63437500061451857, 5.824947211148865298E-16, -4.756430356249998326 ) ) ;
#1887=VECTOR ( 'NONE', #21892, 1000.000000000000000 ) ;
#1889=CARTESIAN_POINT ( 'NONE',  ( 17.55937500061451573, 4.119189519843966529, -2.378215178124998275 ) ) ;
#1896=CARTESIAN_POINT ( 'NONE',  ( 16.42500000000000071, 4.330127018922191873, 2.499999999999999556 ) ) ;
#1900=CARTESIAN_POINT ( 'NONE',  ( 22.80937500061451573, 2.746126346562645981, -4.756430356249997438 ) ) ;
#1907=CARTESIAN_POINT ( 'NONE',  ( 24.34687500061451715, 0.000000000000000000, 4.756430356249998326 ) ) ;
#1909=CARTESIAN_POINT ( 'NONE',  ( 8.521875000614517859, 4.119189519843966529, 2.378215178124999607 ) ) ;
#1921=CARTESIAN_POINT ( 'NONE',  ( 12.94687500061451502, 4.119189519843966529, -2.378215178124998275 ) ) ;
#1939=CARTESIAN_POINT ( 'NONE',  ( 19.77187500061451786, 2.746126346562645981, -4.756430356249997438 ) ) ;
#1975=CARTESIAN_POINT ( 'NONE',  ( 23.14687500061451786, -2.746126346562646425, 4.756430356249996549 ) ) ;
#1981=CARTESIAN_POINT ( 'NONE',  ( 25.83749999999999858, 5.773502691896255534, 3.535250795749688894E-16 ) ) ;
#1989=CARTESIAN_POINT ( 'NONE',  ( 9.206250001229033586, 4.330127018922192761, -2.499999999999997780 ) ) ;
#1992=CARTESIAN_POINT ( 'NONE',  ( 17.97187500061451360, 4.119189519843966529, 2.378215178124999607 ) ) ;
#2004=CARTESIAN_POINT ( 'NONE',  ( 9.909375000614517148, 2.746126346562643317, 4.756430356249998326 ) ) ;
#2010=ORIENTED_EDGE ( 'NONE', *, *, #40326, .T. ) ;
#2015=CARTESIAN_POINT ( 'NONE',  ( 27.49687500061451573, 0.000000000000000000, 4.756430356249998326 ) ) ;
#2018=CARTESIAN_POINT ( 'NONE',  ( 8.437500000000000000, -2.886751345948129988, 4.999999999999997335 ) ) ;
#2021=ORIENTED_EDGE ( 'NONE', *, *, #59244, .T. ) ;
#2026=CARTESIAN_POINT ( 'NONE',  ( 28.80937500061451573, 4.119189519843966529, -2.378215178124998275 ) ) ;
#2028=CARTESIAN_POINT ( 'NONE',  ( 28.73437500061451644, 5.492252693125287522, 3.363034840372157021E-16 ) ) ;
#2029=CARTESIAN_POINT ( 'NONE',  ( 9.571875000614518569, 2.746126346562643317, 4.756430356249998326 ) ) ;
#2043=CARTESIAN_POINT ( 'NONE',  ( 22.06875000122903074, -5.773502691896255534, -1.060575238724906372E-15 ) ) ;
#2058=CARTESIAN_POINT ( 'NONE',  ( 29.74687500061451217, 5.492252693125287522, 3.363034840372157021E-16 ) ) ;
#2068=FACE_OUTER_BOUND ( 'NONE', #6092, .T. ) ;
#2077=CARTESIAN_POINT ( 'NONE',  ( 28.25625000122903074, 0.000000000000000000, 4.999999999999998224 ) ) ;
#2080=VERTEX_POINT ( 'NONE', #36056 ) ;
#2084=LINE ( 'NONE', #13876, #33673 ) ;
#2094=CARTESIAN_POINT ( 'NONE',  ( 15.42187500061451466, -4.119189519843968306, 2.378215178124996054 ) ) ;
#2102=CARTESIAN_POINT ( 'NONE',  ( 11.49375000122903145, 5.773502691896255534, 3.535250795749688401E-16 ) ) ;
#2113=CARTESIAN_POINT ( 'NONE',  ( 18.49687500061452283, 5.492252693125287522, 3.363034840372157021E-16 ) ) ;
#2122=EDGE_CURVE ( 'NONE', #31702, #69475, #39613, .T. ) ;
#2144=EDGE_LOOP ( 'NONE', ( #2437, #31615, #54378, #3537 ) ) ;
#2156=CARTESIAN_POINT ( 'NONE',  ( 28.46249999999999858, 2.886751345948129099, -4.999999999999998224 ) ) ;
#2165=CYLINDRICAL_SURFACE ( 'NONE', #11436, 4.999999999999998224 ) ;
#2174=CARTESIAN_POINT ( 'NONE',  ( 16.47187500061451715, 5.824947211148865298E-16, -4.756430356249998326 ) ) ;
#2177=CARTESIAN_POINT ( 'NONE',  ( 23.48437500061451644, -2.746126346562646425, 4.756430356249996549 ) ) ;
#2185=CARTESIAN_POINT ( 'NONE',  ( 18.52499999999999858, 6.123233995736764310E-16, -4.999999999999998224 ) ) ;
#2192=CARTESIAN_POINT ( 'NONE',  ( 27.27187500061451431, -5.492252693125287522, -1.008910452111647106E-15 ) ) ;
#2211=CARTESIAN_POINT ( 'NONE',  ( 13.17187500061451821, 2.746126346562643317, 4.756430356249998326 ) ) ;
#2216=ADVANCED_FACE ( 'NONE', ( #14247 ), #53785, .T. ) ;
#2225=CARTESIAN_POINT ( 'NONE',  ( 21.93750000000000000, -2.886751345948130876, 4.999999999999996447 ) ) ;
#2240=CARTESIAN_POINT ( 'NONE',  ( 13.88437500061451679, 5.824947211148865298E-16, -4.756430356249998326 ) ) ;
#2246=CARTESIAN_POINT ( 'NONE',  ( 18.00000000000000355, -4.330127018922190985, -2.500000000000001332 ) ) ;
#2250=CARTESIAN_POINT ( 'NONE',  ( 23.93437500061451573, -2.746126346562646425, 4.756430356249996549 ) ) ;
#2254=CARTESIAN_POINT ( 'NONE',  ( 26.43750000000000355, -2.886751345948143310, 4.999999999999972466 ) ) ;
#2257=( BOUNDED_CURVE ( )  B_SPLINE_CURVE ( 2, ( #19511, #64956, #8081, #42435, #36883, #59401, #8810 ),
 .UNSPECIFIED., .F., .F. ) 
 B_SPLINE_CURVE_WITH_KNOTS ( ( 3, 2, 2, 3 ),
 ( 0.2600000000000000644, 0.2633333333333333637, 0.2666666666666667185, 0.2700000000000000733 ),
 .UNSPECIFIED. ) 
 CURVE ( )  GEOMETRIC_REPRESENTATION_ITEM ( )  RATIONAL_B_SPLINE_CURVE ( ( 0.9999999999999977796, 0.8660254037844409281, 1.000000000000000000, 0.8660254037844387076, 1.000000000000000000, 0.8660254037844364872, 1.000000000000002220 ) ) 
 REPRESENTATION_ITEM ( '' )  );
#2260=CARTESIAN_POINT ( 'NONE',  ( 23.52187500061451431, -4.119189519843968306, 2.378215178124996054 ) ) ;
#2262=CARTESIAN_POINT ( 'NONE',  ( 8.034375000614515372, 5.492252693125287522, 3.363034840372157021E-16 ) ) ;
#2269=EDGE_LOOP ( 'NONE', ( #54628, #66842, #1379, #38711 ) ) ;
#2271=CARTESIAN_POINT ( 'NONE',  ( 11.37187500061451573, -4.119189519843968306, 2.378215178124996054 ) ) ;
#2291=CARTESIAN_POINT ( 'NONE',  ( 19.50937500061451857, 0.000000000000000000, 4.756430356249998326 ) ) ;
#2325=CARTESIAN_POINT ( 'NONE',  ( 22.50937500061451857, 4.119189519843966529, -2.378215178124998275 ) ) ;
#2330=CARTESIAN_POINT ( 'NONE',  ( 24.07499999999999929, 4.330127018922191873, 2.499999999999999556 ) ) ;
#2335=CARTESIAN_POINT ( 'NONE',  ( 45.00000000000000000, 0.000000000000000000, 4.999999999999998224 ) ) ;
#2341=CARTESIAN_POINT ( 'NONE',  ( 28.62187500061451217, 5.824947211148865298E-16, -4.756430356249998326 ) ) ;
#2343=CARTESIAN_POINT ( 'NONE',  ( 16.17187500061451644, 4.119189519843966529, 2.378215178124999607 ) ) ;
#2355=CARTESIAN_POINT ( 'NONE',  ( 11.40937500061451360, -5.492252693125287522, -1.008910452111647106E-15 ) ) ;
#2366=CARTESIAN_POINT ( 'NONE',  ( 28.28437500061451360, 5.492252693125287522, 3.363034840372157021E-16 ) ) ;
#2369=CARTESIAN_POINT ( 'NONE',  ( 8.062500000000000000, -5.773502691896255534, -1.060575238724906372E-15 ) ) ;
#2377=CARTESIAN_POINT ( 'NONE',  ( 27.90937500061451715, 4.119189519843966529, -2.378215178124998275 ) ) ;
#2379=CARTESIAN_POINT ( 'NONE',  ( 10.54687500061451644, -2.746126346562646425, 4.756430356249996549 ) ) ;
#2394=CARTESIAN_POINT ( 'NONE',  ( 20.38125000122903430, 6.123233995736764310E-16, -4.999999999999998224 ) ) ;
#2417=CARTESIAN_POINT ( 'NONE',  ( 45.00000000000000000, 0.000000000000000000, 0.000000000000000000 ) ) ;
#2421=CARTESIAN_POINT ( 'NONE',  ( 45.00000000000000000, 6.123233995736764310E-16, -4.999999999999998224 ) ) ;
#2426=DIRECTION ( 'NONE',  ( -1.000000000000000000, -0.000000000000000000, -0.000000000000000000 ) ) ;
#2433=CARTESIAN_POINT ( 'NONE',  ( 27.58125000122903359, 6.123233995736764310E-16, -4.999999999999998224 ) ) ;
#2437=ORIENTED_EDGE ( 'NONE', *, *, #32834, .F. ) ;
#2441=CARTESIAN_POINT ( 'NONE',  ( 25.94999999999999929, 0.000000000000000000, 4.999999999999998224 ) ) ;
#2444=CARTESIAN_POINT ( 'NONE',  ( 16.09687500061451715, 4.119189519843966529, -2.378215178124998275 ) ) ;
#2452=CYLINDRICAL_SURFACE ( 'NONE', #69010, 4.999999999999998224 ) ;
#2459=CARTESIAN_POINT ( 'NONE',  ( 9.356250001229033941, 0.000000000000000000, 4.999999999999998224 ) ) ;
#2460=CARTESIAN_POINT ( 'NONE',  ( 14.13750000000000107, 5.773502691896255534, 3.535250795749688401E-16 ) ) ;
#2461=CARTESIAN_POINT ( 'NONE',  ( 45.00000000000000000, 6.123233995736764310E-16, -4.999999999999998224 ) ) ;
#2463=CARTESIAN_POINT ( 'NONE',  ( 27.35625000122903216, 0.000000000000000000, 4.999999999999998224 ) ) ;
#2464=CARTESIAN_POINT ( 'NONE',  ( 17.78437500061451715, -4.119189519843968306, 2.378215178124996054 ) ) ;
#2477=CARTESIAN_POINT ( 'NONE',  ( 13.95000000000000107, -4.330127018922190985, -2.500000000000001332 ) ) ;
#2481=CARTESIAN_POINT ( 'NONE',  ( 27.61875000122903145, 2.886751345948129099, -4.999999999999998224 ) ) ;
#2500=PRODUCT_DEFINITION ( 'UNKNOWN', '', #41496, #8500 ) ;
#2508=CARTESIAN_POINT ( 'NONE',  ( 7.959375000614516971, -4.119189519843965641, -2.378215178125001383 ) ) ;
#2511=AXIS2_PLACEMENT_3D ( 'NONE', #7, #11071, #28074 ) ;
#2515=EDGE_CURVE ( 'NONE', #24010, #53411, #49114, .T. ) ;
#2519=CYLINDRICAL_SURFACE ( 'NONE', #71610, 4.999999999999998224 ) ;
#2530=CARTESIAN_POINT ( 'NONE',  ( 14.10937500061451644, -5.492252693125287522, -1.008910452111647106E-15 ) ) ;
#2533=CARTESIAN_POINT ( 'NONE',  ( 23.93437500061451573, -2.746126346562646425, 4.756430356249996549 ) ) ;
#2541=CARTESIAN_POINT ( 'NONE',  ( 23.43750000000000000, -2.886751345948153968, -4.999999999999952038 ) ) ;
#2542=CARTESIAN_POINT ( 'NONE',  ( 45.00000000000000000, 0.000000000000000000, 0.000000000000000000 ) ) ;
#2549=CARTESIAN_POINT ( 'NONE',  ( 23.74687500061451573, -2.746126346562642428, -4.756430356249999214 ) ) ;
#2567=CARTESIAN_POINT ( 'NONE',  ( 13.09687500061451537, 5.492252693125287522, 3.363034840372157021E-16 ) ) ;
#2596=CARTESIAN_POINT ( 'NONE',  ( 13.80937500061451750, -4.119189519843965641, -2.378215178125001383 ) ) ;
#2602=CARTESIAN_POINT ( 'NONE',  ( 15.56250000000000000, 2.886751345948126879, 4.999999999999999112 ) ) ;
#2606=CARTESIAN_POINT ( 'NONE',  ( 24.30937500061451573, 2.746126346562643317, 4.756430356249998326 ) ) ;
#2607=CARTESIAN_POINT ( 'NONE',  ( 15.67500000000000071, -4.330127018922194537, 2.499999999999995559 ) ) ;
#2615=CARTESIAN_POINT ( 'NONE',  ( 21.42187500061451644, 5.824947211148865298E-16, -4.756430356249998326 ) ) ;
#2617=CARTESIAN_POINT ( 'NONE',  ( 7.734375000614519102, -2.746126346562646425, 4.756430356249996549 ) ) ;
#2625=CARTESIAN_POINT ( 'NONE',  ( 8.756250001229034297, 4.330127018922192761, -2.499999999999997780 ) ) ;
#2628=CARTESIAN_POINT ( 'NONE',  ( 9.834375000614514306, 5.492252693125287522, 3.363034840372157021E-16 ) ) ;
#2631=( BOUNDED_CURVE ( )  B_SPLINE_CURVE ( 3, ( #61263, #54627, #16909, #26558 ),
 .UNSPECIFIED., .F., .F. ) 
 B_SPLINE_CURVE_WITH_KNOTS ( ( 4, 4 ),
 ( 3.141592653589793116, 4.712388980384689674 ),
 .UNSPECIFIED. ) 
 CURVE ( )  GEOMETRIC_REPRESENTATION_ITEM ( )  RATIONAL_B_SPLINE_CURVE ( ( 1.000000000000000000, 0.8047378541243649375, 0.8047378541243649375, 1.000000000000000000 ) ) 
 REPRESENTATION_ITEM ( '' )  );
#2651=EDGE_CURVE ( 'NONE', #53197, #48464, #51910, .T. ) ;
#2653=CARTESIAN_POINT ( 'NONE',  ( 20.18437500061451573, 5.824947211148865298E-16, -4.756430356249998326 ) ) ;
#2687=CARTESIAN_POINT ( 'NONE',  ( 21.94687500061451857, -2.746126346562642428, -4.756430356249999214 ) ) ;
#2690=EDGE_CURVE ( 'NONE', #33907, #58199, #16803, .T. ) ;
#2695=CARTESIAN_POINT ( 'NONE',  ( 23.43750000000000000, -2.886751345948125991, -5.000000000000000000 ) ) ;
#2701=CARTESIAN_POINT ( 'NONE',  ( 18.73125000122903216, 4.330127018922191873, 2.499999999999999556 ) ) ;
#2705=CARTESIAN_POINT ( 'NONE',  ( 28.65937500061451715, 2.746126346562645981, -4.756430356249997438 ) ) ;
#2707=CARTESIAN_POINT ( 'NONE',  ( 15.04687500061451466, -4.119189519843965641, -2.378215178125001383 ) ) ;
#2719=CARTESIAN_POINT ( 'NONE',  ( 7.546875000614516438, 4.119189519843966529, -2.378215178124998275 ) ) ;
#2731=CARTESIAN_POINT ( 'NONE',  ( 29.48437500061451644, -2.746126346562642428, -4.756430356249999214 ) ) ;
#2734=CARTESIAN_POINT ( 'NONE',  ( 9.112500000000000711, 2.886751345948129099, -4.999999999999998224 ) ) ;
#2741=CARTESIAN_POINT ( 'NONE',  ( 26.93437500061451573, 5.824947211148865298E-16, -4.756430356249998326 ) ) ;
#2743=CARTESIAN_POINT ( 'NONE',  ( 9.309375000614517504, -4.119189519843965641, -2.378215178125001383 ) ) ;
#2759=CARTESIAN_POINT ( 'NONE',  ( 20.49375000122903501, 5.773502691896255534, 3.535250795749688894E-16 ) ) ;
#2767=CARTESIAN_POINT ( 'NONE',  ( 7.856250001229033053, 4.330127018922192761, -2.499999999999997780 ) ) ;
#2774=CARTESIAN_POINT ( 'NONE',  ( 27.75937500061451502, -4.119189519843965641, -2.378215178125001383 ) ) ;
#2782=CARTESIAN_POINT ( 'NONE',  ( 24.82499999999999929, 6.123233995736764310E-16, -4.999999999999998224 ) ) ;
#2783=EDGE_CURVE ( 'NONE', #4916, #19922, #26439, .T. ) ;
#2795=CYLINDRICAL_SURFACE ( 'NONE', #7670, 4.999999999999998224 ) ;
#2803=ORIENTED_EDGE ( 'NONE', *, *, #45125, .F. ) ;
#2810=CARTESIAN_POINT ( 'NONE',  ( 16.84687500061451715, -4.119189519843965641, -2.378215178125001383 ) ) ;
#2830=CARTESIAN_POINT ( 'NONE',  ( 18.68437500061451928, -4.119189519843968306, 2.378215178124996054 ) ) ;
#2843=CARTESIAN_POINT ( 'NONE',  ( 45.00000000000000000, 6.123233995736764310E-16, -4.999999999999998224 ) ) ;
#2847=CARTESIAN_POINT ( 'NONE',  ( 27.09375000122903288, -2.886751345948125991, -5.000000000000000000 ) ) ;
#2872=CARTESIAN_POINT ( 'NONE',  ( 45.00000000000000000, 2.500000000000000000, -3.500000000000000000 ) ) ;
#2873=CARTESIAN_POINT ( 'NONE',  ( 28.94999999999999929, 4.330127018922192761, -2.499999999999997780 ) ) ;
#2888=( BOUNDED_CURVE ( )  B_SPLINE_CURVE ( 2, ( #41429, #24059, #40705, #58757, #57676, #7081, #827 ),
 .UNSPECIFIED., .F., .F. ) 
 B_SPLINE_CURVE_WITH_KNOTS ( ( 3, 2, 2, 3 ),
 ( 0.009999999999999979391, 0.01333333333333330643, 0.01666666666666663174, 0.01999999999999995878 ),
 .UNSPECIFIED. ) 
 CURVE ( )  GEOMETRIC_REPRESENTATION_ITEM ( )  RATIONAL_B_SPLINE_CURVE ( ( 1.000000000000000888, 0.8660254037844378194, 1.000000000000000000, 0.8660254037844387076, 1.000000000000000000, 0.8660254037844403729, 0.9999999999999983347 ) ) 
 REPRESENTATION_ITEM ( '' )  );
#2891=CARTESIAN_POINT ( 'NONE',  ( 16.39687500061451431, -4.119189519843965641, -2.378215178125001383 ) ) ;
#2894=CARTESIAN_POINT ( 'NONE',  ( 24.27187500061451431, 4.119189519843966529, 2.378215178124999607 ) ) ;
#2905=CARTESIAN_POINT ( 'NONE',  ( 12.00000000000000000, 0.000000000000000000, 4.999999999999998224 ) ) ;
#2912=CARTESIAN_POINT ( 'NONE',  ( 25.47187500061451715, -5.492252693125287522, -1.008910452111647106E-15 ) ) ;
#2926=AXIS2_PLACEMENT_3D ( 'NONE', #23677, #1168, #63567 ) ;
#2934=CARTESIAN_POINT ( 'NONE',  ( 13.24687500061451750, -2.746126346562646425, 4.756430356249996549 ) ) ;
#2947=ORIENTED_EDGE ( 'NONE', *, *, #20762, .F. ) ;
#2959=ORIENTED_EDGE ( 'NONE', *, *, #70747, .F. ) ;
#2962=CARTESIAN_POINT ( 'NONE',  ( 14.07187500061451679, 2.746126346562643317, 4.756430356249998326 ) ) ;
#2966=VECTOR ( 'NONE', #39359, 1000.000000000000000 ) ;
#2968=AXIS2_PLACEMENT_3D ( 'NONE', #71232, #47603, #37613 ) ;
#2972=CARTESIAN_POINT ( 'NONE',  ( 14.96250000000000036, 2.886751345948129099, -4.999999999999998224 ) ) ;
#2975=CARTESIAN_POINT ( 'NONE',  ( 24.71250000000000213, -5.773502691896255534, -1.060575238724906372E-15 ) ) ;
#2977=CARTESIAN_POINT ( 'NONE',  ( 15.78749999999999432, -2.886751345948181946, -4.999999999999904077 ) ) ;
#2983=CARTESIAN_POINT ( 'NONE',  ( 23.10937500061451644, -5.492252693125287522, -1.008910452111647106E-15 ) ) ;
#2985=CARTESIAN_POINT ( 'NONE',  ( 8.821875000614515017, 5.824947211148865298E-16, -4.756430356249998326 ) ) ;
#2996=CARTESIAN_POINT ( 'NONE',  ( 10.32187500061451679, 4.119189519843966529, 2.378215178124999607 ) ) ;
#3015=CARTESIAN_POINT ( 'NONE',  ( 22.80000000000000071, 0.000000000000000000, 4.999999999999998224 ) ) ;
#3018=CARTESIAN_POINT ( 'NONE',  ( 20.70937500061451786, 4.119189519843966529, -2.378215178124998275 ) ) ;
#3026=CIRCLE ( 'NONE', #4197, 4.999999999999998224 ) ;
#3037=EDGE_CURVE ( 'NONE', #72150, #24785, #8967, .T. ) ;
#3045=DIRECTION ( 'NONE',  ( -1.000000000000000000, -0.000000000000000000, -0.000000000000000000 ) ) ;
#3053=CARTESIAN_POINT ( 'NONE',  ( 21.45937500061451786, -4.119189519843965641, -2.378215178125001383 ) ) ;
#3059=CARTESIAN_POINT ( 'NONE',  ( 22.83749999999999858, -2.886751345948129988, 4.999999999999997335 ) ) ;
#3062=CARTESIAN_POINT ( 'NONE',  ( 25.27499999999999858, 6.123233995736764310E-16, -4.999999999999998224 ) ) ;
#3065=EDGE_CURVE ( 'NONE', #50451, #66756, #62271, .T. ) ;
#3067=CARTESIAN_POINT ( 'NONE',  ( 13.79999999999999893, 0.000000000000000000, 4.999999999999998224 ) ) ;
#3069=( BOUNDED_CURVE ( )  B_SPLINE_CURVE ( 2, ( #24738, #69461, #63541, #68736, #28838, #2225, #62815 ),
 .UNSPECIFIED., .F., .F. ) 
 B_SPLINE_CURVE_WITH_KNOTS ( ( 3, 2, 2, 3 ),
 ( 0.3500000000000000888, 0.3533333333333333881, 0.3566666666666667429, 0.3599999999999999867 ),
 .UNSPECIFIED. ) 
 CURVE ( )  GEOMETRIC_REPRESENTATION_ITEM ( )  RATIONAL_B_SPLINE_CURVE ( ( 0.9999999999999955591, 0.8660254037844431485, 1.000000000000000000, 0.8660254037844387076, 1.000000000000000000, 0.8660254037844387076, 1.000000000000000000 ) ) 
 REPRESENTATION_ITEM ( '' )  );
#3072=CARTESIAN_POINT ( 'NONE',  ( 7.181250001229034119, -4.330127018922194537, 2.499999999999995559 ) ) ;
#3075=CARTESIAN_POINT ( 'NONE',  ( 16.99687500061451573, 4.119189519843966529, -2.378215178124998275 ) ) ;
#3096=CARTESIAN_POINT ( 'NONE',  ( 28.17187500061451289, 5.824947211148865298E-16, -4.756430356249998326 ) ) ;
#3107=CARTESIAN_POINT ( 'NONE',  ( 27.45937500061451786, 4.119189519843966529, -2.378215178124998275 ) ) ;
#3109=CARTESIAN_POINT ( 'NONE',  ( 10.43437500061451750, 4.119189519843966529, 2.378215178124999607 ) ) ;
#3118=CARTESIAN_POINT ( 'NONE',  ( 45.00000000000000000, 0.000000000000000000, 4.999999999999998224 ) ) ;
#3120=AXIS2_PLACEMENT_3D ( 'NONE', #19948, #42501, #14413 ) ;
#3129=CARTESIAN_POINT ( 'NONE',  ( 20.94375000122902719, 5.773502691896255534, 3.535250795749688894E-16 ) ) ;
#3141=( BOUNDED_CURVE ( )  B_SPLINE_CURVE ( 2, ( #30041, #52579, #8978, #48505, #48136, #41856, #69933 ),
 .UNSPECIFIED., .F., .F. ) 
 B_SPLINE_CURVE_WITH_KNOTS ( ( 3, 2, 2, 3 ),
 ( 0.5000000000000001110, 0.5033333333333334103, 0.5066666666666667096, 0.5100000000000000089 ),
 .UNSPECIFIED. ) 
 CURVE ( )  GEOMETRIC_REPRESENTATION_ITEM ( )  RATIONAL_B_SPLINE_CURVE ( ( 0.9999999999999955591, 0.8660254037844431485, 1.000000000000000000, 0.8660254037844387076, 1.000000000000000000, 0.8660254037844387076, 1.000000000000000000 ) ) 
 REPRESENTATION_ITEM ( '' )  );
#3147=CARTESIAN_POINT ( 'NONE',  ( 29.29687500061451644, 5.492252693125287522, 3.363034840372157021E-16 ) ) ;
#3166=CARTESIAN_POINT ( 'NONE',  ( 11.00625000122903252, 4.330127018922192761, -2.499999999999997780 ) ) ;
#3173=EDGE_CURVE ( 'NONE', #69337, #40700, #203, .T. ) ;
#3184=CARTESIAN_POINT ( 'NONE',  ( 16.80937500061451573, -5.492252693125287522, -1.008910452111647106E-15 ) ) ;
#3189=CARTESIAN_POINT ( 'NONE',  ( 22.57499999999999929, 6.123233995736764310E-16, -4.999999999999998224 ) ) ;
#3203=CARTESIAN_POINT ( 'NONE',  ( 18.19687500061451502, -2.746126346562646425, 4.756430356249996549 ) ) ;
#3214=ORIENTED_EDGE ( 'NONE', *, *, #57780, .F. ) ;
#3221=CARTESIAN_POINT ( 'NONE',  ( 27.05625000122903145, -4.330127018922190985, -2.500000000000001332 ) ) ;
#3224=AXIS2_PLACEMENT_3D ( 'NONE', #12254, #46972, #34423 ) ;
#3225=CARTESIAN_POINT ( 'NONE',  ( 0.000000000000000000, 4.999999999999998224, 0.000000000000000000 ) ) ;
#3246=CARTESIAN_POINT ( 'NONE',  ( 17.53125000122903288, -4.330127018922194537, 2.499999999999995559 ) ) ;
#3247=CARTESIAN_POINT ( 'NONE',  ( 7.809375000614519280, 0.000000000000000000, 4.756430356249998326 ) ) ;
#3253=CARTESIAN_POINT ( 'NONE',  ( 27.33750000000000213, -2.886751345948088243, 5.000000000000068390 ) ) ;
#3266=CARTESIAN_POINT ( 'NONE',  ( 16.13437500061451502, 5.492252693125287522, 3.363034840372157021E-16 ) ) ;
#3270=CARTESIAN_POINT ( 'NONE',  ( 23.74687500061451573, 4.119189519843966529, -2.378215178124998275 ) ) ;
#3275=CARTESIAN_POINT ( 'NONE',  ( 15.88125000122903074, 6.123233995736764310E-16, -4.999999999999998224 ) ) ;
#3280=CARTESIAN_POINT ( 'NONE',  ( 14.02499999999999858, 6.123233995736764310E-16, -4.999999999999998224 ) ) ;
#3287=CARTESIAN_POINT ( 'NONE',  ( 24.98437500061451644, -4.119189519843968306, 2.378215178124996054 ) ) ;
#3290=( BOUNDED_CURVE ( )  B_SPLINE_CURVE ( 2, ( #30362, #18528, #52169, #18885, #63244, #46991, #36266 ),
 .UNSPECIFIED., .F., .F. ) 
 B_SPLINE_CURVE_WITH_KNOTS ( ( 3, 2, 2, 3 ),
 ( 0.000000000000000000, 0.003333333333333326608, 0.006666666666666653217, 0.009999999999999979391 ),
 .UNSPECIFIED. ) 
 CURVE ( )  GEOMETRIC_REPRESENTATION_ITEM ( )  RATIONAL_B_SPLINE_CURVE ( ( 1.000000000000000000, 0.8660254037844387076, 1.000000000000000000, 0.8660254037844387076, 1.000000000000000000, 0.8660254037844395958, 0.9999999999999991118 ) ) 
 REPRESENTATION_ITEM ( '' )  );
#3300=ORIENTED_EDGE ( 'NONE', *, *, #46331, .T. ) ;
#3309=CARTESIAN_POINT ( 'NONE',  ( 11.52187500061451608, -5.492252693125287522, -1.008910452111647106E-15 ) ) ;
#3324=VERTEX_POINT ( 'NONE', #20057 ) ;
#3327=CARTESIAN_POINT ( 'NONE',  ( 16.12500000000000000, -4.330127018922194537, 2.499999999999995559 ) ) ;
#3341=CARTESIAN_POINT ( 'NONE',  ( 14.44687500061451679, 5.492252693125287522, 3.363034840372157021E-16 ) ) ;
#3350=CARTESIAN_POINT ( 'NONE',  ( 14.43750000000000000, -2.886751345948125991, -5.000000000000000000 ) ) ;
#3358=CARTESIAN_POINT ( 'NONE',  ( 19.96875000122903288, 2.886751345948073588, -5.000000000000094147 ) ) ;
#3363=CARTESIAN_POINT ( 'NONE',  ( 21.90937500061451715, 2.746126346562645981, -4.756430356249997438 ) ) ;
#3365=CARTESIAN_POINT ( 'NONE',  ( 9.196875000614515017, -4.119189519843965641, -2.378215178125001383 ) ) ;
#3376=CARTESIAN_POINT ( 'NONE',  ( 8.821875000614515017, 5.824947211148865298E-16, -4.756430356249998326 ) ) ;
#3382=DIRECTION ( 'NONE',  ( -1.000000000000000000, -0.000000000000000000, -0.000000000000000000 ) ) ;
#3385=( BOUNDED_CURVE ( )  B_SPLINE_CURVE ( 2, ( #40780, #51856, #46679, #27975, #57744, #1258, #18578 ),
 .UNSPECIFIED., .F., .F. ) 
 B_SPLINE_CURVE_WITH_KNOTS ( ( 3, 2, 2, 3 ),
 ( 0.2399999999999999634, 0.2433333333333333182, 0.2466666666666666452, 0.2499999999999999722 ),
 .UNSPECIFIED. ) 
 CURVE ( )  GEOMETRIC_REPRESENTATION_ITEM ( )  RATIONAL_B_SPLINE_CURVE ( ( 1.000000000000001110, 0.8660254037844374864, 1.000000000000000000, 0.8660254037844387076, 1.000000000000000000, 0.8660254037844398178, 0.9999999999999988898 ) ) 
 REPRESENTATION_ITEM ( '' )  );
#3387=ORIENTED_EDGE ( 'NONE', *, *, #58181, .F. ) ;
#3399=CARTESIAN_POINT ( 'NONE',  ( 18.57187500061451857, 2.746126346562643317, 4.756430356249998326 ) ) ;
#3406=EDGE_CURVE ( 'NONE', #69693, #30697, #11344, .T. ) ;
#3431=CARTESIAN_POINT ( 'NONE',  ( 20.07187500061451857, -5.492252693125287522, -1.008910452111647106E-15 ) ) ;
#3438=CARTESIAN_POINT ( 'NONE',  ( 22.34999999999999787, 0.000000000000000000, 4.999999999999998224 ) ) ;
#3440=CARTESIAN_POINT ( 'NONE',  ( 9.187500000000001776, 5.773502691896255534, 3.535250795749688401E-16 ) ) ;
#3443=CARTESIAN_POINT ( 'NONE',  ( 12.05625000122903145, 0.000000000000000000, 4.999999999999998224 ) ) ;
#3444=CYLINDRICAL_SURFACE ( 'NONE', #64377, 4.999999999999998224 ) ;
#3449=CARTESIAN_POINT ( 'NONE',  ( 28.69687500061451502, 4.119189519843966529, -2.378215178124998275 ) ) ;
#3451=CARTESIAN_POINT ( 'NONE',  ( 15.30937500061451573, 2.746126346562643317, 4.756430356249998326 ) ) ;
#3454=ORIENTED_EDGE ( 'NONE', *, *, #50099, .T. ) ;
#3461=CARTESIAN_POINT ( 'NONE',  ( 9.121875000614517504, -4.119189519843968306, 2.378215178124996054 ) ) ;
#3466=ORIENTED_EDGE ( 'NONE', *, *, #3037, .T. ) ;
#3472=CARTESIAN_POINT ( 'NONE',  ( 28.24687500061451217, 4.119189519843966529, -2.378215178124998275 ) ) ;
#3476=CARTESIAN_POINT ( 'NONE',  ( 9.225000000000001421, 4.330127018922191873, 2.499999999999999556 ) ) ;
#3480=EDGE_CURVE ( 'NONE', #25370, #59877, #65508, .T. ) ;
#3485=CARTESIAN_POINT ( 'NONE',  ( 26.03437500061451715, 5.824947211148865298E-16, -4.756430356249998326 ) ) ;
#3487=CARTESIAN_POINT ( 'NONE',  ( 10.50937500061451679, 0.000000000000000000, 4.756430356249998326 ) ) ;
#3503=CARTESIAN_POINT ( 'NONE',  ( 20.98125000122903216, 4.330127018922191873, 2.499999999999999556 ) ) ;
#3517=CARTESIAN_POINT ( 'NONE',  ( 27.19687500061451857, -2.746126346562646425, 4.756430356249996549 ) ) ;
#3525=CARTESIAN_POINT ( 'NONE',  ( 22.14375000122903359, -2.886751345948153968, -4.999999999999952038 ) ) ;
#3537=ORIENTED_EDGE ( 'NONE', *, *, #17177, .F. ) ;
#3550=CARTESIAN_POINT ( 'NONE',  ( 11.66249999999999964, -5.773502691896255534, -1.060575238724906372E-15 ) ) ;
#3553=CARTESIAN_POINT ( 'NONE',  ( 16.13437500061451502, 5.492252693125287522, 3.363034840372157021E-16 ) ) ;
#3564=CARTESIAN_POINT ( 'NONE',  ( 16.93125000122903145, 4.330127018922191873, 2.499999999999999556 ) ) ;
#3572=CARTESIAN_POINT ( 'NONE',  ( 17.70937500061451431, 0.000000000000000000, 4.756430356249998326 ) ) ;
#3583=FACE_OUTER_BOUND ( 'NONE', #19784, .T. ) ;
#3590=CARTESIAN_POINT ( 'NONE',  ( 28.36875000122903145, -5.773502691896255534, -1.060575238724906372E-15 ) ) ;
#3592=CARTESIAN_POINT ( 'NONE',  ( 45.00000000000000000, 0.000000000000000000, 4.999999999999998224 ) ) ;
#3601=VERTEX_POINT ( 'NONE', #24880 ) ;
#3614=CARTESIAN_POINT ( 'NONE',  ( 25.05000000000000071, 0.000000000000000000, 4.999999999999998224 ) ) ;
#3615=CARTESIAN_POINT ( 'NONE',  ( 29.62500000000000000, -4.330127018922194537, 2.499999999999995559 ) ) ;
#3620=CARTESIAN_POINT ( 'NONE',  ( 21.67500000000000071, 6.123233995736764310E-16, -4.999999999999998224 ) ) ;
#3633=CARTESIAN_POINT ( 'NONE',  ( 12.00937500061451502, 2.746126346562645981, -4.756430356249997438 ) ) ;
#3637=CARTESIAN_POINT ( 'NONE',  ( 24.68437500061451573, 5.492252693125287522, 3.363034840372157021E-16 ) ) ;
#3647=CARTESIAN_POINT ( 'NONE',  ( 12.86250000000000071, 2.886751345948126879, 4.999999999999999112 ) ) ;
#3654=CARTESIAN_POINT ( 'NONE',  ( 25.62187500061451573, 2.746126346562645981, -4.756430356249997438 ) ) ;
#3675=CARTESIAN_POINT ( 'NONE',  ( 9.046875000614518214, 5.492252693125287522, 3.363034840372157021E-16 ) ) ;
#3702=CARTESIAN_POINT ( 'NONE',  ( 13.17187500061451999, 2.746126346562643317, 4.756430356249998326 ) ) ;
#3706=STYLED_ITEM ( 'NONE', ( #8294 ), #10934 ) ;
#3711=CARTESIAN_POINT ( 'NONE',  ( 15.48749999999999893, 5.773502691896255534, 3.535250795749688894E-16 ) ) ;
#3713=CARTESIAN_POINT ( 'NONE',  ( 21.28125000122903288, 6.123233995736764310E-16, -4.999999999999998224 ) ) ;
#3725=CARTESIAN_POINT ( 'NONE',  ( 23.37187500061451573, 4.119189519843966529, 2.378215178124999607 ) ) ;
#3738=CARTESIAN_POINT ( 'NONE',  ( 10.13437500061451502, -2.746126346562642428, -4.756430356249999214 ) ) ;
#3761=CARTESIAN_POINT ( 'NONE',  ( 16.58437500061451786, 5.824947211148865298E-16, -4.756430356249998326 ) ) ;
#3773=ORIENTED_EDGE ( 'NONE', *, *, #43418, .F. ) ;
#3795=CARTESIAN_POINT ( 'NONE',  ( 22.24687500061451217, -2.746126346562646425, 4.756430356249996549 ) ) ;
#3802=CARTESIAN_POINT ( 'NONE',  ( 22.94999999999999929, -4.330127018922190985, -2.500000000000001332 ) ) ;
#3806=CARTESIAN_POINT ( 'NONE',  ( 18.54375000122903216, -2.886751345948181946, -4.999999999999904077 ) ) ;
#3808=CARTESIAN_POINT ( 'NONE',  ( 28.23749999999999716, -2.886751345948137093, 4.999999999999984901 ) ) ;
#3814=CARTESIAN_POINT ( 'NONE',  ( 29.48437500061451644, -2.746126346562642428, -4.756430356249999214 ) ) ;
#3816=CARTESIAN_POINT ( 'NONE',  ( 16.95937500061451431, 2.746126346562645981, -4.756430356249997438 ) ) ;
#3822=CARTESIAN_POINT ( 'NONE',  ( 26.02499999999999858, -4.330127018922194537, 2.499999999999995559 ) ) ;
#3825=CARTESIAN_POINT ( 'NONE',  ( 16.55625000122903145, 0.000000000000000000, 4.999999999999998224 ) ) ;
#3826=CARTESIAN_POINT ( 'NONE',  ( 8.709375000614516082, -5.492252693125287522, -1.008910452111647106E-15 ) ) ;
#3848=CARTESIAN_POINT ( 'NONE',  ( 26.67187500061451644, 2.746126346562643317, 4.756430356249998326 ) ) ;
#3850=CARTESIAN_POINT ( 'NONE',  ( 7.921875000614517326, -5.492252693125287522, -1.008910452111647106E-15 ) ) ;
#3866=CARTESIAN_POINT ( 'NONE',  ( 17.60625000122903572, -4.330127018922190985, -2.500000000000001332 ) ) ;
#3882=ADVANCED_FACE ( 'NONE', ( #38906 ), #27093, .T. ) ;
#3884=CARTESIAN_POINT ( 'NONE',  ( 28.24687500061451573, -2.746126346562642428, -4.756430356249999214 ) ) ;
#3918=CARTESIAN_POINT ( 'NONE',  ( 11.55000000000000071, 0.000000000000000000, 4.999999999999998224 ) ) ;
#3921=CARTESIAN_POINT ( 'NONE',  ( 13.47187500061451715, 4.119189519843966529, 2.378215178124999607 ) ) ;
#3940=CARTESIAN_POINT ( 'NONE',  ( 15.60937500061451644, -4.119189519843965641, -2.378215178125001383 ) ) ;
#3950=CARTESIAN_POINT ( 'NONE',  ( 13.06875000122903252, -5.773502691896255534, -1.060575238724906372E-15 ) ) ;
#3953=CARTESIAN_POINT ( 'NONE',  ( 24.50625000122903074, 4.330127018922192761, -2.499999999999997780 ) ) ;
#3957=CARTESIAN_POINT ( 'NONE',  ( 29.15625000122903288, 0.000000000000000000, 4.999999999999998224 ) ) ;
#3959=CARTESIAN_POINT ( 'NONE',  ( 26.90625000122902932, 0.000000000000000000, 4.999999999999998224 ) ) ;
#3969=EDGE_LOOP ( 'NONE', ( #38470, #37871, #37135, #21085, #9447, #39565, #454, #49334, #57532, #30105, #69830, #43814, #15641, #22569, #61517, #15338, #6826, #41283, #5734, #50296, #19819, #53002, #52502, #21761, #36258, #29483, #62501, #50659, #31162, #28528, #2803, #23071, #10901, #23829, #14031, #59663, #20232, #21301, #19195, #60039, #44630, #32712, #23652, #32547, #4840, #34362, #911, #52509, #22582, #58085, #33339, #45827, #27225, #48022, #64051, #16436, #17205, #44911, #31975, #29923, #29249, #3387, #7442, #35869, #45244, #40070, #52077, #23066, #67874, #71276, #16373, #61647, #11771, #14855, #44854, #54439, #45179, #33522, #29666, #14102, #18956, #50395, #23163, #18490, #48751, #64611, #55896, #8587, #54471, #58855, #52237, #6386, #37665, #7894, #21537, #71421, #47543, #41892, #71650, #64408, #39084, #40079, #67576 ) ) ;
#3983=CARTESIAN_POINT ( 'NONE',  ( 27.56250000000000000, 2.886751345948129099, -4.999999999999998224 ) ) ;
#4007=CARTESIAN_POINT ( 'NONE',  ( 20.85937500061451644, -5.492252693125287522, -1.008910452111647106E-15 ) ) ;
#4011=CARTESIAN_POINT ( 'NONE',  ( 16.06875000122903074, 2.886751345948126879, 4.999999999999998224 ) ) ;
#4016=CARTESIAN_POINT ( 'NONE',  ( 13.19999999999999929, 4.330127018922192761, -2.499999999999997780 ) ) ;
#4023=CARTESIAN_POINT ( 'NONE',  ( 24.60937500061451644, -4.119189519843965641, -2.378215178125001383 ) ) ;
#4044=CARTESIAN_POINT ( 'NONE',  ( 9.909375000614517148, 4.119189519843966529, -2.378215178124998275 ) ) ;
#4058=CARTESIAN_POINT ( 'NONE',  ( 16.27499999999999858, 6.123233995736764310E-16, -4.999999999999998224 ) ) ;
#4067=ORIENTED_EDGE ( 'NONE', *, *, #24303, .T. ) ;
#4070=CARTESIAN_POINT ( 'NONE',  ( 11.85937500061451644, 0.000000000000000000, 4.756430356249998326 ) ) ;
#4090=CARTESIAN_POINT ( 'NONE',  ( 21.04687500061451644, 4.119189519843966529, -2.378215178124998275 ) ) ;
#4093=CARTESIAN_POINT ( 'NONE',  ( 14.53125000122903288, 6.123233995736764310E-16, -4.999999999999998224 ) ) ;
#4109=CARTESIAN_POINT ( 'NONE',  ( 9.084375000614516082, -2.746126346562646425, 4.756430356249996549 ) ) ;
#4130=CARTESIAN_POINT ( 'NONE',  ( 17.18437500061451573, 4.119189519843966529, 2.378215178124999607 ) ) ;
#4148=LINE ( 'NONE', #53275, #62074 ) ;
#4159=AXIS2_PLACEMENT_3D ( 'NONE', #29800, #57509, #6911 ) ;
#4162=CARTESIAN_POINT ( 'NONE',  ( 20.52187500061451786, -5.492252693125287522, -1.008910452111647106E-15 ) ) ;
#4169=CARTESIAN_POINT ( 'NONE',  ( 23.25000000000000000, 0.000000000000000000, 4.999999999999998224 ) ) ;
#4172=CARTESIAN_POINT ( 'NONE',  ( 18.43125000122903501, -4.330127018922194537, 2.499999999999995559 ) ) ;
#4175=CARTESIAN_POINT ( 'NONE',  ( 24.22500000000000142, -4.330127018922194537, 2.499999999999995559 ) ) ;
#4179=CARTESIAN_POINT ( 'NONE',  ( 26.74687500061451573, -4.119189519843965641, -2.378215178125001383 ) ) ;
#4181=CARTESIAN_POINT ( 'NONE',  ( 13.39687500061451431, 4.119189519843966529, -2.378215178124998275 ) ) ;
#4192=CARTESIAN_POINT ( 'NONE',  ( 8.934375000614515727, 5.492252693125287522, 3.363034840372157021E-16 ) ) ;
#4197=AXIS2_PLACEMENT_3D ( 'NONE', #19143, #47604, #46158 ) ;
#4204=CARTESIAN_POINT ( 'NONE',  ( 16.33125000122903359, 6.123233995736764310E-16, -4.999999999999998224 ) ) ;
#4216=CARTESIAN_POINT ( 'NONE',  ( 23.22187500061451715, -5.492252693125287522, -1.008910452111647106E-15 ) ) ;
#4218=CARTESIAN_POINT ( 'NONE',  ( 8.784375000614518925, -4.119189519843968306, 2.378215178124996054 ) ) ;
#4237=CARTESIAN_POINT ( 'NONE',  ( 18.65625000122902932, 4.330127018922192761, -2.499999999999997780 ) ) ;
#4239=DIRECTION ( 'NONE',  ( 0.000000000000000000, 0.000000000000000000, 1.000000000000000000 ) ) ;
#4240=VERTEX_POINT ( 'NONE', #46616 ) ;
#4254=CARTESIAN_POINT ( 'NONE',  ( 28.99687500061451573, -2.746126346562646425, 4.756430356249996549 ) ) ;
#4259=ADVANCED_FACE ( 'NONE', ( #62155 ), #12265, .T. ) ;
#4263=CARTESIAN_POINT ( 'NONE',  ( 24.97499999999999787, 4.330127018922191873, 2.499999999999999556 ) ) ;
#4273=CARTESIAN_POINT ( 'NONE',  ( 21.23437500061451644, -2.746126346562646425, 4.756430356249996549 ) ) ;
#4282=VERTEX_POINT ( 'NONE', #62869 ) ;
#4290=CARTESIAN_POINT ( 'NONE',  ( 15.23437500061451644, 5.492252693125287522, 3.363034840372157021E-16 ) ) ;
#4292=AXIS2_PLACEMENT_3D ( 'NONE', #32297, #36736, #4239 ) ;
#4309=CARTESIAN_POINT ( 'NONE',  ( 27.13125000122903430, 6.123233995736764310E-16, -4.999999999999998224 ) ) ;
#4310=CARTESIAN_POINT ( 'NONE',  ( 14.82187500061451679, 2.746126346562645981, -4.756430356249997438 ) ) ;
#4329=CARTESIAN_POINT ( 'NONE',  ( 25.44375000122903074, 5.773502691896255534, 3.535250795749688894E-16 ) ) ;
#4339=EDGE_LOOP ( 'NONE', ( #44542, #11640, #13920, #65373 ) ) ;
#4373=ORIENTED_EDGE ( 'NONE', *, *, #58181, .T. ) ;
#4376=CARTESIAN_POINT ( 'NONE',  ( 22.20937500061451786, -5.492252693125287522, -1.008910452111647106E-15 ) ) ;
#4385=CARTESIAN_POINT ( 'NONE',  ( 13.79999999999999893, 0.000000000000000000, 4.999999999999998224 ) ) ;
#4393=CARTESIAN_POINT ( 'NONE',  ( 21.30937500061451573, 0.000000000000000000, 4.756430356249998326 ) ) ;
#4396=CARTESIAN_POINT ( 'NONE',  ( 22.40625000122903288, 0.000000000000000000, 4.999999999999998224 ) ) ;
#4404=ORIENTED_EDGE ( 'NONE', *, *, #51739, .T. ) ;
#4410=LINE ( 'NONE', #50917, #49252 ) ;
#4415=CARTESIAN_POINT ( 'NONE',  ( 9.271875000614519635, -5.492252693125287522, -1.008910452111647106E-15 ) ) ;
#4438=CARTESIAN_POINT ( 'NONE',  ( 11.22187500061451892, 2.746126346562645981, -4.756430356249997438 ) ) ;
#4448=CARTESIAN_POINT ( 'NONE',  ( 16.72500000000000142, 6.123233995736764310E-16, -4.999999999999998224 ) ) ;
#4458=CARTESIAN_POINT ( 'NONE',  ( 19.28437500061451715, 5.492252693125287522, 3.363034840372157021E-16 ) ) ;
#4461=CARTESIAN_POINT ( 'NONE',  ( 13.89375000122903536, -2.886751345948129988, 4.999999999999997335 ) ) ;
#4474=CARTESIAN_POINT ( 'NONE',  ( 29.03437500061451715, -4.119189519843968306, 2.378215178124996054 ) ) ;
#4482=CYLINDRICAL_SURFACE ( 'NONE', #38309, 4.999999999999998224 ) ;
#4497=CARTESIAN_POINT ( 'NONE',  ( 16.88437500061451502, -4.119189519843968306, 2.378215178124996054 ) ) ;
#4528=CARTESIAN_POINT ( 'NONE',  ( 18.90937500061451360, 4.119189519843966529, -2.378215178124998275 ) ) ;
#4530=EDGE_CURVE ( 'NONE', #59687, #19922, #58042, .T. ) ;
#4535=CARTESIAN_POINT ( 'NONE',  ( 20.66250000000000142, -5.773502691896255534, -1.060575238724906372E-15 ) ) ;
#4538=CARTESIAN_POINT ( 'NONE',  ( 17.62500000000000000, 6.123233995736764310E-16, -4.999999999999998224 ) ) ;
#4540=CARTESIAN_POINT ( 'NONE',  ( 17.47499999999999787, -4.330127018922194537, 2.499999999999995559 ) ) ;
#4544=CARTESIAN_POINT ( 'NONE',  ( 27.83437500061451075, 5.492252693125287522, 3.363034840372157021E-16 ) ) ;
#4546=CARTESIAN_POINT ( 'NONE',  ( 12.87187500061451750, 5.824947211148865298E-16, -4.756430356249998326 ) ) ;
#4557=EDGE_LOOP ( 'NONE', ( #30061, #35969, #11210, #14169 ) ) ;
#4558=EDGE_CURVE ( 'NONE', #47688, #38854, #26886, .T. ) ;
#4563=ORIENTED_EDGE ( 'NONE', *, *, #21957, .F. ) ;
#4569=ORIENTED_EDGE ( 'NONE', *, *, #62104, .T. ) ;
#4571=CARTESIAN_POINT ( 'NONE',  ( 29.47499999999999787, 4.330127018922191873, 2.499999999999999556 ) ) ;
#4578=CARTESIAN_POINT ( 'NONE',  ( 24.87187500061451573, 2.746126346562643317, 4.756430356249998326 ) ) ;
#4580=CARTESIAN_POINT ( 'NONE',  ( 8.896875000614517859, -2.746126346562642428, -4.756430356249999214 ) ) ;
#4587=CARTESIAN_POINT ( 'NONE',  ( 27.18750000000000000, 5.773502691896255534, 3.535250795749688401E-16 ) ) ;
#4597=CARTESIAN_POINT ( 'NONE',  ( 19.66875000122903216, 2.886751345948126879, 4.999999999999999112 ) ) ;
#4599=CARTESIAN_POINT ( 'NONE',  ( 13.63125000122903252, 6.123233995736764310E-16, -4.999999999999998224 ) ) ;
#4614=CARTESIAN_POINT ( 'NONE',  ( 25.84687500061451360, -2.746126346562646425, 4.756430356249996549 ) ) ;
#4627=CARTESIAN_POINT ( 'NONE',  ( 27.75000000000000000, 0.000000000000000000, 4.999999999999998224 ) ) ;
#4629=CARTESIAN_POINT ( 'NONE',  ( 11.19375000122903252, -2.886751345948129988, 4.999999999999997335 ) ) ;
#4633=CARTESIAN_POINT ( 'NONE',  ( 20.29687500061451289, 0.000000000000000000, 4.756430356249998326 ) ) ;
#4636=ORIENTED_EDGE ( 'NONE', *, *, #47275, .F. ) ;
#4637=CARTESIAN_POINT ( 'NONE',  ( 45.00000000000000000, 0.000000000000000000, 4.999999999999998224 ) ) ;
#4639=CYLINDRICAL_SURFACE ( 'NONE', #68731, 4.999999999999998224 ) ;
#4652=CARTESIAN_POINT ( 'NONE',  ( 14.22187500061451537, 5.824947211148865298E-16, -4.756430356249998326 ) ) ;
#4663=CARTESIAN_POINT ( 'NONE',  ( 13.18125000122903323, 6.123233995736764310E-16, -4.999999999999998224 ) ) ;
#4667=CARTESIAN_POINT ( 'NONE',  ( 29.22187500061451360, 4.119189519843966529, 2.378215178124999607 ) ) ;
#4668=CARTESIAN_POINT ( 'NONE',  ( 15.30937500061451750, 4.119189519843966529, -2.378215178124998275 ) ) ;
#4685=CARTESIAN_POINT ( 'NONE',  ( 26.34375000122903288, 5.773502691896255534, 3.535250795749688894E-16 ) ) ;
#4697=LINE ( 'NONE', #9864, #23334 ) ;
#4713=CARTESIAN_POINT ( 'NONE',  ( 12.52500000000000213, -4.330127018922194537, 2.499999999999995559 ) ) ;
#4717=CARTESIAN_POINT ( 'NONE',  ( 26.00625000122903074, 0.000000000000000000, 4.999999999999998224 ) ) ;
#4732=CARTESIAN_POINT ( 'NONE',  ( 21.38437500061451502, -2.746126346562642428, -4.756430356249999214 ) ) ;
#4739=CARTESIAN_POINT ( 'NONE',  ( 26.66250000000000142, 2.886751345948129099, -4.999999999999997335 ) ) ;
#4740=ORIENTED_EDGE ( 'NONE', *, *, #71606, .T. ) ;
#4741=CARTESIAN_POINT ( 'NONE',  ( 11.10000000000000142, 0.000000000000000000, 4.999999999999998224 ) ) ;
#4748=CARTESIAN_POINT ( 'NONE',  ( 21.34687500061451715, -2.746126346562646425, 4.756430356249996549 ) ) ;
#4770=CARTESIAN_POINT ( 'NONE',  ( 11.07187500061451679, -5.492252693125287522, -1.008910452111647106E-15 ) ) ;
#4778=VERTEX_POINT ( 'NONE', #31071 ) ;
#4794=CARTESIAN_POINT ( 'NONE',  ( 10.58437500061451964, -4.119189519843968306, 2.378215178124996054 ) ) ;
#4814=CARTESIAN_POINT ( 'NONE',  ( 19.09687500061451360, -4.119189519843965641, -2.378215178125001383 ) ) ;
#4817=CARTESIAN_POINT ( 'NONE',  ( 13.48125000122903394, -4.330127018922194537, 2.499999999999995559 ) ) ;
#4831=CARTESIAN_POINT ( 'NONE',  ( 29.40937500061451715, 0.000000000000000000, 4.756430356249998326 ) ) ;
#4840=ORIENTED_EDGE ( 'NONE', *, *, #1055, .F. ) ;
#4852=CARTESIAN_POINT ( 'NONE',  ( 17.85937500061451999, -4.119189519843965641, -2.378215178125001383 ) ) ;
#4856=ORIENTED_EDGE ( 'NONE', *, *, #35798, .T. ) ;
#4866=ORIENTED_EDGE ( 'NONE', *, *, #14038, .F. ) ;
#4884=CARTESIAN_POINT ( 'NONE',  ( 19.54687500061451644, -2.746126346562646425, 4.756430356249996549 ) ) ;
#4891=CARTESIAN_POINT ( 'NONE',  ( 20.69999999999999929, -4.330127018922190985, -2.500000000000001332 ) ) ;
#4894=CARTESIAN_POINT ( 'NONE',  ( 26.67187500061451289, -4.119189519843968306, 2.378215178124996054 ) ) ;
#4895=CARTESIAN_POINT ( 'NONE',  ( 24.16875000122903216, 2.886751345948112668, 5.000000000000023981 ) ) ;
#4897=CARTESIAN_POINT ( 'NONE',  ( 28.42499999999999716, 6.123233995736764310E-16, -4.999999999999998224 ) ) ;
#4898=CARTESIAN_POINT ( 'NONE',  ( 24.18750000000000355, -2.886751345948102898, 5.000000000000044409 ) ) ;
#4902=CARTESIAN_POINT ( 'NONE',  ( 28.20937500061451075, 2.746126346562645981, -4.756430356249997438 ) ) ;
#4904=CARTESIAN_POINT ( 'NONE',  ( 14.55937500061451573, -5.492252693125287522, -1.008910452111647106E-15 ) ) ;
#4910=CARTESIAN_POINT ( 'NONE',  ( 45.00000000000000000, 0.000000000000000000, 0.000000000000000000 ) ) ;
#4914=DIRECTION ( 'NONE',  ( 0.000000000000000000, 0.000000000000000000, 1.000000000000000000 ) ) ;
#4915=FACE_BOUND ( 'NONE', #44003, .T. ) ;
#4916=VERTEX_POINT ( 'NONE', #43999 ) ;
#4921=ORIENTED_EDGE ( 'NONE', *, *, #55404, .T. ) ;
#4931=CARTESIAN_POINT ( 'NONE',  ( 25.66875000122903216, -5.773502691896255534, -1.060575238724906372E-15 ) ) ;
#4939=CARTESIAN_POINT ( 'NONE',  ( 24.83437500061451431, 4.119189519843966529, 2.378215178124999607 ) ) ;
#4941=CARTESIAN_POINT ( 'NONE',  ( 8.634375000614518569, 4.119189519843966529, 2.378215178124999607 ) ) ;
#4946=ORIENTED_EDGE ( 'NONE', *, *, #24217, .F. ) ;
#4958=CARTESIAN_POINT ( 'NONE',  ( 19.33125000122903359, -4.330127018922194537, 2.499999999999995559 ) ) ;
#4960=CARTESIAN_POINT ( 'NONE',  ( 29.60625000122903216, 0.000000000000000000, 4.999999999999998224 ) ) ;
#4967=DIRECTION ( 'NONE',  ( 0.000000000000000000, 0.000000000000000000, 1.000000000000000000 ) ) ;
#4973=CARTESIAN_POINT ( 'NONE',  ( 25.58437500061451431, 5.824947211148865298E-16, -4.756430356249998326 ) ) ;
#4988=CARTESIAN_POINT ( 'NONE',  ( 12.80625000122903323, 4.330127018922192761, -2.499999999999997780 ) ) ;
#4990=CARTESIAN_POINT ( 'NONE',  ( 34.99999999999999289, 0.000000000000000000, 0.000000000000000000 ) ) ;
#4992=CARTESIAN_POINT ( 'NONE',  ( 21.49687500061451573, 4.119189519843966529, -2.378215178124998275 ) ) ;
#4995=VERTEX_POINT ( 'NONE', #71335 ) ;
#4998=CARTESIAN_POINT ( 'NONE',  ( 45.00000000000000000, 0.000000000000000000, 0.000000000000000000 ) ) ;
#5003=CARTESIAN_POINT ( 'NONE',  ( 13.62187500061451750, -4.119189519843968306, 2.378215178124996054 ) ) ;
#5012=CARTESIAN_POINT ( 'NONE',  ( 14.70937500061451431, 2.746126346562645981, -4.756430356249997438 ) ) ;
#5026=CARTESIAN_POINT ( 'NONE',  ( 14.70937500061451786, -4.119189519843965641, -2.378215178125001383 ) ) ;
#5029=( BOUNDED_CURVE ( )  B_SPLINE_CURVE ( 2, ( #64835, #20119, #59278, #43777, #15317, #71852, #66304 ),
 .UNSPECIFIED., .F., .F. ) 
 B_SPLINE_CURVE_WITH_KNOTS ( ( 3, 2, 2, 3 ),
 ( 0.9799999999999999822, 0.9833333333333333925, 0.9866666666666668029, 0.9900000000000002132 ),
 .UNSPECIFIED. ) 
 CURVE ( )  GEOMETRIC_REPRESENTATION_ITEM ( )  RATIONAL_B_SPLINE_CURVE ( ( 1.000000000000000000, 0.8660254037844387076, 1.000000000000000000, 0.8660254037844387076, 1.000000000000000000, 0.8660254037844298258, 1.000000000000008882 ) ) 
 REPRESENTATION_ITEM ( '' )  );
#5033=CARTESIAN_POINT ( 'NONE',  ( 10.61250000000000071, 2.886751345948238789, 4.999999999999807265 ) ) ;
#5036=AXIS2_PLACEMENT_3D ( 'NONE', #55619, #21994, #32722 ) ;
#5046=CARTESIAN_POINT ( 'NONE',  ( 26.15625000122903288, -4.330127018922190985, -2.500000000000001332 ) ) ;
#5062=ADVANCED_FACE ( 'NONE', ( #15901 ), #72426, .T. ) ;
#5067=EDGE_CURVE ( 'NONE', #33154, #22800, #15171, .T. ) ;
#5085=DIRECTION ( 'NONE',  ( -1.000000000000000000, -0.000000000000000000, -0.000000000000000000 ) ) ;
#5090=ORIENTED_EDGE ( 'NONE', *, *, #66497, .F. ) ;
#5093=CARTESIAN_POINT ( 'NONE',  ( 22.02187500061451431, 4.119189519843966529, 2.378215178124999607 ) ) ;
#5102=CARTESIAN_POINT ( 'NONE',  ( 11.40000000000000036, 4.330127018922192761, -2.499999999999997780 ) ) ;
#5110=CARTESIAN_POINT ( 'NONE',  ( 22.43437500061451573, 5.824947211148865298E-16, -4.756430356249998326 ) ) ;
#5132=CARTESIAN_POINT ( 'NONE',  ( 9.084375000614517859, 4.119189519843966529, 2.378215178124999607 ) ) ;
#5151=EDGE_CURVE ( 'NONE', #21883, #44291, #71709, .T. ) ;
#5154=CARTESIAN_POINT ( 'NONE',  ( 12.38437500061451857, -4.119189519843968306, 2.378215178124996054 ) ) ;
#5164=CARTESIAN_POINT ( 'NONE',  ( 45.00000000000000000, 6.123233995736764310E-16, -4.999999999999998224 ) ) ;
#5165=CARTESIAN_POINT ( 'NONE',  ( 45.00000000000000000, 0.000000000000000000, 0.000000000000000000 ) ) ;
#5169=DIRECTION ( 'NONE',  ( -1.000000000000000000, -0.000000000000000000, -0.000000000000000000 ) ) ;
#5172=LINE ( 'NONE', #34318, #31635 ) ;
#5174=CARTESIAN_POINT ( 'NONE',  ( 20.63437500061451502, 5.492252693125287522, 3.363034840372157021E-16 ) ) ;
#5177=CARTESIAN_POINT ( 'NONE',  ( 13.33125000122903359, 4.330127018922191873, 2.499999999999999556 ) ) ;
#5191=CARTESIAN_POINT ( 'NONE',  ( 29.48437500061451644, -4.119189519843968306, 2.378215178124996054 ) ) ;
#5210=CARTESIAN_POINT ( 'NONE',  ( 16.32187500061451502, 2.746126346562643317, 4.756430356249998326 ) ) ;
#5214=ORIENTED_EDGE ( 'NONE', *, *, #71351, .F. ) ;
#5224=EDGE_LOOP ( 'NONE', ( #29968, #17834, #57777, #70360 ) ) ;
#5244=CARTESIAN_POINT ( 'NONE',  ( 18.75937500061451857, -4.119189519843965641, -2.378215178125001383 ) ) ;
#5245=CARTESIAN_POINT ( 'NONE',  ( 14.60625000122903216, 4.330127018922192761, -2.499999999999997780 ) ) ;
#5249=CARTESIAN_POINT ( 'NONE',  ( 19.53749999999999432, 5.773502691896255534, 3.535250795749688894E-16 ) ) ;
#5252=CARTESIAN_POINT ( 'NONE',  ( 20.60625000122902861, 0.000000000000000000, 4.999999999999998224 ) ) ;
#5253=CARTESIAN_POINT ( 'NONE',  ( 25.54687500061451644, 4.119189519843966529, -2.378215178124998275 ) ) ;
#5254=CARTESIAN_POINT ( 'NONE',  ( 24.05625000122903145, 4.330127018922192761, -2.499999999999997780 ) ) ;
#5259=CARTESIAN_POINT ( 'NONE',  ( 27.87187500061451217, 4.119189519843966529, 2.378215178124999607 ) ) ;
#5261=CARTESIAN_POINT ( 'NONE',  ( 13.09687500061451715, 0.000000000000000000, 4.756430356249998326 ) ) ;
#5271=CARTESIAN_POINT ( 'NONE',  ( 45.00000000000000000, 6.123233995736764310E-16, -4.999999999999998224 ) ) ;
#5278=EDGE_CURVE ( 'NONE', #59530, #39431, #54709, .T. ) ;
#5285=CARTESIAN_POINT ( 'NONE',  ( 16.21875000122903643, -5.773502691896255534, -1.060575238724906372E-15 ) ) ;
#5292=EDGE_CURVE ( 'NONE', #59817, #30697, #28451, .T. ) ;
#5297=CARTESIAN_POINT ( 'NONE',  ( 24.79687500061452354, 5.492252693125287522, 3.363034840372157021E-16 ) ) ;
#5302=EDGE_CURVE ( 'NONE', #61284, #68160, #23261, .T. ) ;
#5319=CARTESIAN_POINT ( 'NONE',  ( 17.64375000122903003, -2.886751345948125991, -5.000000000000000000 ) ) ;
#5336=CARTESIAN_POINT ( 'NONE',  ( 24.98437500061451644, -4.119189519843968306, 2.378215178124996054 ) ) ;
#5342=CARTESIAN_POINT ( 'NONE',  ( 26.36249999999999716, 2.886751345948126879, 4.999999999999999112 ) ) ;
#5350=CARTESIAN_POINT ( 'NONE',  ( 10.89375000122903003, -2.886751345948125991, -5.000000000000000000 ) ) ;
#5354=CARTESIAN_POINT ( 'NONE',  ( 21.79687500061451644, -4.119189519843965641, -2.378215178125001383 ) ) ;
#5365=CARTESIAN_POINT ( 'NONE',  ( 12.45937500061451608, 2.746126346562645981, -4.756430356249997438 ) ) ;
#5386=CARTESIAN_POINT ( 'NONE',  ( 17.06250000000000000, -5.773502691896255534, -1.060575238724906372E-15 ) ) ;
#5389=CARTESIAN_POINT ( 'NONE',  ( 15.34687500061451537, 5.492252693125287522, 3.363034840372157021E-16 ) ) ;
#5393=EDGE_CURVE ( 'NONE', #50344, #27832, #69810, .T. ) ;
#5396=CARTESIAN_POINT ( 'NONE',  ( 10.57500000000000107, 4.330127018922191873, 2.499999999999999556 ) ) ;
#5408=CARTESIAN_POINT ( 'NONE',  ( 27.01875000122903359, -5.773502691896255534, -1.060575238724906372E-15 ) ) ;
#5412=DIRECTION ( 'NONE',  ( 0.000000000000000000, 0.000000000000000000, 1.000000000000000000 ) ) ;
#5421=CARTESIAN_POINT ( 'NONE',  ( 23.94375000122903074, -2.886751345948112224, -5.000000000000023981 ) ) ;
#5450=( BOUNDED_CURVE ( )  B_SPLINE_CURVE ( 2, ( #58196, #41588, #30138, #36039, #57483, #46410, #58559 ),
 .UNSPECIFIED., .F., .F. ) 
 B_SPLINE_CURVE_WITH_KNOTS ( ( 3, 2, 2, 3 ),
 ( 0.4500000000000000111, 0.4533333333333333104, 0.4566666666666666652, 0.4600000000000000200 ),
 .UNSPECIFIED. ) 
 CURVE ( )  GEOMETRIC_REPRESENTATION_ITEM ( )  RATIONAL_B_SPLINE_CURVE ( ( 1.000000000000000000, 0.8660254037844387076, 1.000000000000000000, 0.8660254037844387076, 1.000000000000000000, 0.8660254037844387076, 1.000000000000000000 ) ) 
 REPRESENTATION_ITEM ( '' )  );
#5455=CARTESIAN_POINT ( 'NONE',  ( 21.34687500061451715, -4.119189519843965641, -2.378215178125001383 ) ) ;
#5466=CARTESIAN_POINT ( 'NONE',  ( 10.91250000000000320, 2.886751345948129099, -4.999999999999998224 ) ) ;
#5474=CARTESIAN_POINT ( 'NONE',  ( 22.50937500061451857, 4.119189519843966529, -2.378215178124998275 ) ) ;
#5485=EDGE_LOOP ( 'NONE', ( #32259, #24814, #18681, #14610, #45131, #14448, #50932 ) ) ;
#5496=CARTESIAN_POINT ( 'NONE',  ( 8.259375000614518569, 0.000000000000000000, 4.756430356249998326 ) ) ;
#5505=ORIENTED_EDGE ( 'NONE', *, *, #48083, .F. ) ;
#5516=ORIENTED_EDGE ( 'NONE', *, *, #41396, .T. ) ;
#5519=CARTESIAN_POINT ( 'NONE',  ( 12.64687500061451608, 5.492252693125287522, 3.363034840372157021E-16 ) ) ;
#5528=CARTESIAN_POINT ( 'NONE',  ( 12.18749999999999645, -2.886751345948181946, -4.999999999999904077 ) ) ;
#5529=VECTOR ( 'NONE', #60915, 1000.000000000000000 ) ;
#5530=CARTESIAN_POINT ( 'NONE',  ( 12.58125000122903359, -4.330127018922194537, 2.499999999999995559 ) ) ;
#5532=DIRECTION ( 'NONE',  ( -1.000000000000000000, -0.000000000000000000, -0.000000000000000000 ) ) ;
#5534=CARTESIAN_POINT ( 'NONE',  ( 19.42499999999999716, 6.123233995736764310E-16, -4.999999999999998224 ) ) ;
#5539=CARTESIAN_POINT ( 'NONE',  ( 20.55937500061451217, 2.746126346562645981, -4.756430356249997438 ) ) ;
#5542=CARTESIAN_POINT ( 'NONE',  ( 14.90625000122903110, -4.330127018922190985, -2.500000000000001332 ) ) ;
#5554=EDGE_CURVE ( 'NONE', #8225, #63037, #22891, .T. ) ;
#5557=CARTESIAN_POINT ( 'NONE',  ( 7.546875000614516438, 4.119189519843966529, -2.378215178124998275 ) ) ;
#5579=CARTESIAN_POINT ( 'NONE',  ( 15.53437500061451715, -4.119189519843968306, 2.378215178124996054 ) ) ;
#5594=ORIENTED_EDGE ( 'NONE', *, *, #48575, .T. ) ;
#5602=AXIS2_PLACEMENT_3D ( 'NONE', #51225, #24581, #69659 ) ;
#5612=CARTESIAN_POINT ( 'NONE',  ( 17.78437500061451715, -4.119189519843968306, 2.378215178124996054 ) ) ;
#5613=DIRECTION ( 'NONE',  ( 0.000000000000000000, -1.000000000000000000, 8.673617379884035472E-17 ) ) ;
#5618=CARTESIAN_POINT ( 'NONE',  ( 20.85000000000000142, 4.330127018922192761, -2.499999999999997780 ) ) ;
#5622=CARTESIAN_POINT ( 'NONE',  ( 24.49687500061451573, -4.119189519843965641, -2.378215178125001383 ) ) ;
#5629=CARTESIAN_POINT ( 'NONE',  ( 26.10937500061451644, 2.746126346562643317, 4.756430356249998326 ) ) ;
#5631=CARTESIAN_POINT ( 'NONE',  ( 12.49687500061451573, 4.119189519843966529, -2.378215178124998275 ) ) ;
#5636=CARTESIAN_POINT ( 'NONE',  ( 16.57499999999999929, -4.330127018922194537, 2.499999999999995559 ) ) ;
#5639=VECTOR ( 'NONE', #24621, 1000.000000000000000 ) ;
#5648=ADVANCED_FACE ( 'NONE', ( #22181 ), #34709, .T. ) ;
#5665=CARTESIAN_POINT ( 'NONE',  ( 23.82187500061451502, 2.746126346562645981, -4.756430356249997438 ) ) ;
#5676=CARTESIAN_POINT ( 'NONE',  ( 15.09375000122903110, 5.773502691896255534, 3.535250795749688401E-16 ) ) ;
#5683=CARTESIAN_POINT ( 'NONE',  ( 17.34375000122903288, 5.773502691896255534, 3.535250795749688894E-16 ) ) ;
#5697=CARTESIAN_POINT ( 'NONE',  ( 26.93437500061451573, 5.824947211148865298E-16, -4.756430356249998326 ) ) ;
#5703=CARTESIAN_POINT ( 'NONE',  ( 27.15000000000000213, 4.330127018922192761, -2.499999999999997780 ) ) ;
#5711=CARTESIAN_POINT ( 'NONE',  ( 12.24375000122903323, -2.886751345948125991, -5.000000000000000000 ) ) ;
#5715=CARTESIAN_POINT ( 'NONE',  ( 21.60937500061451644, 2.746126346562643317, 4.756430356249998326 ) ) ;
#5723=CARTESIAN_POINT ( 'NONE',  ( 10.85625000122903216, -4.330127018922190985, -2.500000000000001332 ) ) ;
#5727=CARTESIAN_POINT ( 'NONE',  ( 13.50937500061451679, 2.746126346562643317, 4.756430356249998326 ) ) ;
#5734=ORIENTED_EDGE ( 'NONE', *, *, #39155, .F. ) ;
#5735=CARTESIAN_POINT ( 'NONE',  ( 19.08749999999999858, 5.773502691896255534, 3.535250795749688401E-16 ) ) ;
#5751=CARTESIAN_POINT ( 'NONE',  ( 29.40937500061451360, -5.492252693125287522, -1.008910452111647106E-15 ) ) ;
#5752=CARTESIAN_POINT ( 'NONE',  ( 13.05937500061451750, 4.119189519843966529, -2.378215178124998275 ) ) ;
#5761=CARTESIAN_POINT ( 'NONE',  ( 19.93125000122903145, 6.123233995736764310E-16, -4.999999999999998224 ) ) ;
#5771=CARTESIAN_POINT ( 'NONE',  ( 26.11875000122902790, -5.773502691896255534, -1.060575238724906372E-15 ) ) ;
#5776=CARTESIAN_POINT ( 'NONE',  ( -2.928932188134523606, -4.999999999999997335, 2.928932188134523606 ) ) ;
#5795=EDGE_CURVE ( 'NONE', #24462, #11954, #63319, .T. ) ;
#5814=CARTESIAN_POINT ( 'NONE',  ( 18.08437500061451075, -2.746126346562646425, 4.756430356249996549 ) ) ;
#5822=CARTESIAN_POINT ( 'NONE',  ( 26.81250000000000000, 2.886751345948126879, 4.999999999999998224 ) ) ;
#5830=CARTESIAN_POINT ( 'NONE',  ( 23.59687500061451715, -2.746126346562646425, 4.756430356249996549 ) ) ;
#5847=CARTESIAN_POINT ( 'NONE',  ( 45.00000000000000000, 0.000000000000000000, 4.999999999999998224 ) ) ;
#5848=EDGE_CURVE ( 'NONE', #48096, #14158, #58125, .T. ) ;
#5865=CYLINDRICAL_SURFACE ( 'NONE', #55222, 4.999999999999998224 ) ;
#5869=EDGE_CURVE ( 'NONE', #10555, #8125, #41127, .T. ) ;
#5874=CARTESIAN_POINT ( 'NONE',  ( 10.13437500061451679, -4.119189519843968306, 2.378215178124996054 ) ) ;
#5881=( BOUNDED_CURVE ( )  B_SPLINE_CURVE ( 2, ( #34955, #51596, #63745, #996, #1353, #13134, #7967 ),
 .UNSPECIFIED., .F., .F. ) 
 B_SPLINE_CURVE_WITH_KNOTS ( ( 3, 2, 2, 3 ),
 ( 0.4600000000000000200, 0.4633333333333333748, 0.4666666666666667851, 0.4700000000000001399 ),
 .UNSPECIFIED. ) 
 CURVE ( )  GEOMETRIC_REPRESENTATION_ITEM ( )  RATIONAL_B_SPLINE_CURVE ( ( 1.000000000000000000, 0.8660254037844387076, 1.000000000000000000, 0.8660254037844387076, 1.000000000000000000, 0.8660254037844320463, 1.000000000000006661 ) ) 
 REPRESENTATION_ITEM ( '' )  );
#5890=CARTESIAN_POINT ( 'NONE',  ( 19.65000000000000213, 0.000000000000000000, 4.999999999999998224 ) ) ;
#5894=CARTESIAN_POINT ( 'NONE',  ( 17.93437500061451573, 5.492252693125287522, 3.363034840372157021E-16 ) ) ;
#5897=CARTESIAN_POINT ( 'NONE',  ( 25.88437500061451857, -2.746126346562642428, -4.756430356249999214 ) ) ;
#5905=CYLINDRICAL_SURFACE ( 'NONE', #14771, 4.999999999999998224 ) ;
#5911=CARTESIAN_POINT ( 'NONE',  ( 28.92187500061451644, 2.746126346562643317, 4.756430356249998326 ) ) ;
#5932=CARTESIAN_POINT ( 'NONE',  ( 13.65937500061451715, 0.000000000000000000, 4.756430356249998326 ) ) ;
#5940=( BOUNDED_CURVE ( )  B_SPLINE_CURVE ( 2, ( #71584, #14683, #9156, #9523, #14325, #26145, #48322 ),
 .UNSPECIFIED., .F., .F. ) 
 B_SPLINE_CURVE_WITH_KNOTS ( ( 3, 2, 2, 3 ),
 ( 0.9000000000000000222, 0.9033333333333333215, 0.9066666666666666208, 0.9100000000000000311 ),
 .UNSPECIFIED. ) 
 CURVE ( )  GEOMETRIC_REPRESENTATION_ITEM ( )  RATIONAL_B_SPLINE_CURVE ( ( 1.000000000000000000, 0.8660254037844387076, 1.000000000000000000, 0.8660254037844387076, 1.000000000000000000, 0.8660254037844387076, 1.000000000000000000 ) ) 
 REPRESENTATION_ITEM ( '' )  );
#5952=EDGE_CURVE ( 'NONE', #19210, #33154, #20825, .T. ) ;
#5961=VERTEX_POINT ( 'NONE', #47527 ) ;
#5964=CARTESIAN_POINT ( 'NONE',  ( 19.35937500061451644, 4.119189519843966529, -2.378215178124998275 ) ) ;
#5965=DIRECTION ( 'NONE',  ( 0.000000000000000000, 0.000000000000000000, 1.000000000000000000 ) ) ;
#5972=CARTESIAN_POINT ( 'NONE',  ( 18.75000000000000000, 0.000000000000000000, 4.999999999999998224 ) ) ;
#5977=CARTESIAN_POINT ( 'NONE',  ( 25.95937500061451431, 2.746126346562645981, -4.756430356249997438 ) ) ;
#5984=CARTESIAN_POINT ( 'NONE',  ( 24.04687500061451289, -4.119189519843965641, -2.378215178125001383 ) ) ;
#5986=CARTESIAN_POINT ( 'NONE',  ( 11.48437500061451644, -2.746126346562641984, -4.756430356249999214 ) ) ;
#5989=EDGE_LOOP ( 'NONE', ( #26647, #40947, #41103, #17915 ) ) ;
#5991=CARTESIAN_POINT ( 'NONE',  ( 45.00000000000000000, 0.000000000000000000, 0.000000000000000000 ) ) ;
#5997=EDGE_LOOP ( 'NONE', ( #61702, #13702, #39988, #34006 ) ) ;
#6019=CARTESIAN_POINT ( 'NONE',  ( 22.77187500061451786, -5.492252693125287522, -1.008910452111647106E-15 ) ) ;
#6032=CARTESIAN_POINT ( 'NONE',  ( 45.00000000000000000, 0.000000000000000000, 4.999999999999998224 ) ) ;
#6039=CARTESIAN_POINT ( 'NONE',  ( 17.26875000122903003, 2.886751345948129099, -4.999999999999998224 ) ) ;
#6054=CARTESIAN_POINT ( 'NONE',  ( 26.63437500061451857, 4.119189519843966529, 2.378215178124999607 ) ) ;
#6061=CARTESIAN_POINT ( 'NONE',  ( 27.63749999999999929, 5.773502691896255534, 3.535250795749688894E-16 ) ) ;
#6068=CARTESIAN_POINT ( 'NONE',  ( 15.33750000000000036, -2.886751345948126435, -5.000000000000000000 ) ) ;
#6070=CARTESIAN_POINT ( 'NONE',  ( 12.20625000122903181, -4.330127018922190985, -2.500000000000001332 ) ) ;
#6072=DIRECTION ( 'NONE',  ( -1.000000000000000000, 0.000000000000000000, 0.000000000000000000 ) ) ;
#6074=CARTESIAN_POINT ( 'NONE',  ( 19.47187500061451360, -4.119189519843968306, 2.378215178124996054 ) ) ;
#6077=VERTEX_POINT ( 'NONE', #4663 ) ;
#6085=CARTESIAN_POINT ( 'NONE',  ( 13.54687500061451466, 0.000000000000000000, 4.756430356249998326 ) ) ;
#6086=VERTEX_POINT ( 'NONE', #44917 ) ;
#6092=EDGE_LOOP ( 'NONE', ( #10688, #72175, #13296, #49439 ) ) ;
#6106=CARTESIAN_POINT ( 'NONE',  ( 29.78437500061451715, 4.119189519843966529, 2.378215178124999607 ) ) ;
#6110=CARTESIAN_POINT ( 'NONE',  ( 12.68437500061451573, 4.119189519843966529, 2.378215178124999607 ) ) ;
#6120=CARTESIAN_POINT ( 'NONE',  ( 11.64375000122903003, -2.886751345948130876, 4.999999999999996447 ) ) ;
#6126=FACE_OUTER_BOUND ( 'NONE', #35513, .T. ) ;
#6127=CARTESIAN_POINT ( 'NONE',  ( 23.38125000122903074, -4.330127018922194537, 2.499999999999995559 ) ) ;
#6130=EDGE_LOOP ( 'NONE', ( #29125, #59504, #27177, #71562 ) ) ;
#6133=CARTESIAN_POINT ( 'NONE',  ( 7.429687500307258219, 0.000000000000000000, 4.878215178124998275 ) ) ;
#6147=( BOUNDED_CURVE ( )  B_SPLINE_CURVE ( 2, ( #63118, #62757, #52042, #23951, #11433, #67951, #46501 ),
 .UNSPECIFIED., .F., .F. ) 
 B_SPLINE_CURVE_WITH_KNOTS ( ( 3, 2, 2, 3 ),
 ( 0.9000000000000000222, 0.9033333333333333215, 0.9066666666666666208, 0.9100000000000000311 ),
 .UNSPECIFIED. ) 
 CURVE ( )  GEOMETRIC_REPRESENTATION_ITEM ( )  RATIONAL_B_SPLINE_CURVE ( ( 1.000000000000000000, 0.8660254037844387076, 1.000000000000000000, 0.8660254037844387076, 1.000000000000000000, 0.8660254037844387076, 1.000000000000000000 ) ) 
 REPRESENTATION_ITEM ( '' )  );
#6175=CARTESIAN_POINT ( 'NONE',  ( 18.72187500061451360, 5.824947211148865298E-16, -4.756430356249998326 ) ) ;
#6177=( BOUNDED_CURVE ( )  B_SPLINE_CURVE ( 2, ( #57360, #18552, #63627, #13017, #35555, #69906, #68828 ),
 .UNSPECIFIED., .F., .F. ) 
 B_SPLINE_CURVE_WITH_KNOTS ( ( 3, 2, 2, 3 ),
 ( 0.9100000000000000311, 0.9133333333333333304, 0.9166666666666667407, 0.9200000000000001510 ),
 .UNSPECIFIED. ) 
 CURVE ( )  GEOMETRIC_REPRESENTATION_ITEM ( )  RATIONAL_B_SPLINE_CURVE ( ( 1.000000000000000000, 0.8660254037844387076, 1.000000000000000000, 0.8660254037844387076, 1.000000000000000000, 0.8660254037844342667, 1.000000000000004441 ) ) 
 REPRESENTATION_ITEM ( '' )  );
#6191=DIRECTION ( 'NONE',  ( -1.000000000000000000, -0.000000000000000000, -0.000000000000000000 ) ) ;
#6192=CARTESIAN_POINT ( 'NONE',  ( 19.80937500061451573, 4.119189519843966529, -2.378215178124998275 ) ) ;
#6195=CARTESIAN_POINT ( 'NONE',  ( 12.90000000000000213, 0.000000000000000000, 4.999999999999998224 ) ) ;
#6237=CARTESIAN_POINT ( 'NONE',  ( 8.896875000614517859, -2.746126346562642428, -4.756430356249999214 ) ) ;
#6249=CARTESIAN_POINT ( 'NONE',  ( 12.61875000122903145, -5.773502691896255534, -1.060575238724906372E-15 ) ) ;
#6258=CARTESIAN_POINT ( 'NONE',  ( 17.40937500061451360, 2.746126346562645981, -4.756430356249997438 ) ) ;
#6261=CARTESIAN_POINT ( 'NONE',  ( 25.62187500061451573, 4.119189519843966529, 2.378215178124999607 ) ) ;
#6275=CARTESIAN_POINT ( 'NONE',  ( 26.63437500061451857, 4.119189519843966529, 2.378215178124999607 ) ) ;
#6295=CARTESIAN_POINT ( 'NONE',  ( 15.12187500061451928, -5.492252693125287522, -1.008910452111647106E-15 ) ) ;
#6326=CARTESIAN_POINT ( 'NONE',  ( 15.98437500061451821, -4.119189519843968306, 2.378215178124996054 ) ) ;
#6332=CARTESIAN_POINT ( 'NONE',  ( 16.50000000000000000, 0.000000000000000000, 4.999999999999998224 ) ) ;
#6336=CARTESIAN_POINT ( 'NONE',  ( 25.47187500061451360, 5.824947211148865298E-16, -4.756430356249998326 ) ) ;
#6344=CARTESIAN_POINT ( 'NONE',  ( 24.15937500061451360, 2.746126346562645981, -4.756430356249997438 ) ) ;
#6346=CARTESIAN_POINT ( 'NONE',  ( 10.54687500061451644, -4.119189519843965641, -2.378215178125001383 ) ) ;
#6354=CYLINDRICAL_SURFACE ( 'NONE', #40790, 4.999999999999998224 ) ;
#6355=CARTESIAN_POINT ( 'NONE',  ( 12.39375000122903536, 5.773502691896255534, 3.535250795749688401E-16 ) ) ;
#6356=ORIENTED_EDGE ( 'NONE', *, *, #28164, .T. ) ;
#6358=CARTESIAN_POINT ( 'NONE',  ( 12.04687500061451821, 4.119189519843966529, -2.378215178124998275 ) ) ;
#6379=CARTESIAN_POINT ( 'NONE',  ( 21.60937500061451644, 4.119189519843966529, -2.378215178124998275 ) ) ;
#6386=ORIENTED_EDGE ( 'NONE', *, *, #26754, .F. ) ;
#6393=CARTESIAN_POINT ( 'NONE',  ( 15.01875000122903359, 2.886751345948129099, -4.999999999999997335 ) ) ;
#6402=CARTESIAN_POINT ( 'NONE',  ( 16.74375000122903145, -2.886751345948125991, -5.000000000000000000 ) ) ;
#6414=EDGE_LOOP ( 'NONE', ( #3300, #61462, #38867, #64999, #62594, #72737, #7843, #19691, #68962, #58407, #32626, #67710, #9221, #27099, #63406, #53640, #63613, #8265, #15789, #15095, #65507, #60274, #10624, #8152, #18946, #3454, #69164, #43392, #47718, #1642, #54428, #4921, #17809, #22288, #6900, #36173, #4404, #15217, #33575, #10677, #73049, #57962, #71011, #25947, #51980, #20052, #3466, #30887, #32828, #54016, #30141, #10444, #55127, #60390, #43428, #68594, #1188, #40212, #35685, #70668, #35167, #65057, #20897, #9079, #63554, #11506, #28171, #12208, #66597, #31842, #21523, #11483, #12619, #36475, #41655, #66185, #70034, #18719, #24752, #26722, #51956, #54731, #10545, #44019, #37149, #45369, #45886, #53781, #57412, #71498, #28480, #19780, #5594, #49346, #69361, #49358, #25795, #23696, #821, #12108, #57282, #6356, #6932 ) ) ;
#6418=CARTESIAN_POINT ( 'NONE',  ( 24.57187500061451502, -5.492252693125287522, -1.008910452111647106E-15 ) ) ;
#6423=CARTESIAN_POINT ( 'NONE',  ( 26.58750000000000213, -2.886751345948125991, -5.000000000000000000 ) ) ;
#6431=CARTESIAN_POINT ( 'NONE',  ( 8.868750001229033231, 2.886751345948126879, 4.999999999999999112 ) ) ;
#6435=CARTESIAN_POINT ( 'NONE',  ( 19.24687500061451573, 4.119189519843966529, -2.378215178124998275 ) ) ;
#6447=CARTESIAN_POINT ( 'NONE',  ( 10.35937500061451644, 2.746126346562643317, 4.756430356249998326 ) ) ;
#6463=VERTEX_POINT ( 'NONE', #12365 ) ;
#6469=CARTESIAN_POINT ( 'NONE',  ( 28.13437500061451502, -4.119189519843968306, 2.378215178124996054 ) ) ;
#6472=CARTESIAN_POINT ( 'NONE',  ( 27.94687500061451502, 0.000000000000000000, 4.756430356249998326 ) ) ;
#6473=CARTESIAN_POINT ( 'NONE',  ( 13.24687500061451750, -2.746126346562646425, 4.756430356249996549 ) ) ;
#6481=EDGE_CURVE ( 'NONE', #53529, #40722, #40677, .T. ) ;
#6489=CARTESIAN_POINT ( 'NONE',  ( 45.00000000000000000, 6.123233995736764310E-16, -4.999999999999998224 ) ) ;
#6490=CARTESIAN_POINT ( 'NONE',  ( 23.79375000122903216, -2.886751345948129988, 4.999999999999997335 ) ) ;
#6493=ORIENTED_EDGE ( 'NONE', *, *, #62104, .F. ) ;
#6498=CARTESIAN_POINT ( 'NONE',  ( 25.40625000122903288, 4.330127018922192761, -2.499999999999997780 ) ) ;
#6507=CARTESIAN_POINT ( 'NONE',  ( 29.59687500061451715, -2.746126346562642428, -4.756430356249999214 ) ) ;
#6527=CARTESIAN_POINT ( 'NONE',  ( 17.92500000000000071, -4.330127018922194537, 2.499999999999995559 ) ) ;
#6538=ORIENTED_EDGE ( 'NONE', *, *, #14507, .F. ) ;
#6541=CARTESIAN_POINT ( 'NONE',  ( 20.03437500061451715, -2.746126346562642428, -4.756430356249999214 ) ) ;
#6554=VECTOR ( 'NONE', #68710, 1000.000000000000000 ) ;
#6560=CARTESIAN_POINT ( 'NONE',  ( 18.83437500061451431, 5.824947211148865298E-16, -4.756430356249998326 ) ) ;
#6568=AXIS2_PLACEMENT_3D ( 'NONE', #2542, #46885, #63855 ) ;
#6572=EDGE_LOOP ( 'NONE', ( #66325, #19695, #30020, #7543 ) ) ;
#6582=( BOUNDED_CURVE ( )  B_SPLINE_CURVE ( 2, ( #57205, #63483, #57572, #56493, #22506, #50955, #35403 ),
 .UNSPECIFIED., .F., .F. ) 
 B_SPLINE_CURVE_WITH_KNOTS ( ( 3, 2, 2, 3 ),
 ( 0.2300000000000000100, 0.2333333333333333370, 0.2366666666666666363, 0.2399999999999999634 ),
 .UNSPECIFIED. ) 
 CURVE ( )  GEOMETRIC_REPRESENTATION_ITEM ( )  RATIONAL_B_SPLINE_CURVE ( ( 1.000000000000000000, 0.8660254037844387076, 1.000000000000000000, 0.8660254037844387076, 1.000000000000000000, 0.8660254037844398178, 0.9999999999999988898 ) ) 
 REPRESENTATION_ITEM ( '' )  );
#6584=FACE_OUTER_BOUND ( 'NONE', #47893, .T. ) ;
#6608=CARTESIAN_POINT ( 'NONE',  ( 9.234375000614518214, -4.119189519843968306, 2.378215178124996054 ) ) ;
#6629=CARTESIAN_POINT ( 'NONE',  ( 17.22187500061451360, -4.119189519843968306, 2.378215178124996054 ) ) ;
#6632=CARTESIAN_POINT ( 'NONE',  ( 26.74687500061451573, -4.119189519843965641, -2.378215178125001383 ) ) ;
#6640=CARTESIAN_POINT ( 'NONE',  ( 28.06875000122903074, 2.886751345948129099, -4.999999999999997335 ) ) ;
#6641=CARTESIAN_POINT ( 'NONE',  ( 45.00000000000000000, 0.000000000000000000, 0.000000000000000000 ) ) ;
#6647=CARTESIAN_POINT ( 'NONE',  ( 28.24687500061451573, -2.746126346562642428, -4.756430356249999214 ) ) ;
#6652=CARTESIAN_POINT ( 'NONE',  ( 45.00000000000000000, 0.000000000000000000, 4.999999999999998224 ) ) ;
#6665=CARTESIAN_POINT ( 'NONE',  ( 14.78437500061451715, 5.824947211148865298E-16, -4.756430356249998326 ) ) ;
#6678=ORIENTED_EDGE ( 'NONE', *, *, #40891, .T. ) ;
#6693=VECTOR ( 'NONE', #67358, 1000.000000000000000 ) ;
#6694=CARTESIAN_POINT ( 'NONE',  ( 16.50937500061451502, -4.119189519843965641, -2.378215178125001383 ) ) ;
#6700=CARTESIAN_POINT ( 'NONE',  ( 17.81250000000000355, 2.886751345948126879, 4.999999999999999112 ) ) ;
#6704=CARTESIAN_POINT ( 'NONE',  ( 24.23437500061451289, 5.492252693125287522, 3.363034840372157021E-16 ) ) ;
#6708=ADVANCED_FACE ( 'NONE', ( #6584 ), #68642, .T. ) ;
#6711=CARTESIAN_POINT ( 'NONE',  ( 25.05937500061451573, 2.746126346562645981, -4.756430356249997438 ) ) ;
#6713=CARTESIAN_POINT ( 'NONE',  ( 12.23437500061451821, -2.746126346562646425, 4.756430356249996549 ) ) ;
#6718=CARTESIAN_POINT ( 'NONE',  ( 16.64999999999999858, -4.330127018922190985, -2.500000000000001332 ) ) ;
#6722=CARTESIAN_POINT ( 'NONE',  ( 15.93750000000000000, 5.773502691896255534, 3.535250795749688401E-16 ) ) ;
#6725=CARTESIAN_POINT ( 'NONE',  ( 12.57187500061451502, 4.119189519843966529, 2.378215178124999607 ) ) ;
#6742=CARTESIAN_POINT ( 'NONE',  ( 11.47499999999999964, 4.330127018922191873, 2.499999999999999556 ) ) ;
#6745=CARTESIAN_POINT ( 'NONE',  ( 21.90937500061451715, -4.119189519843965641, -2.378215178125001383 ) ) ;
#6764=CARTESIAN_POINT ( 'NONE',  ( 17.11875000122903145, -5.773502691896255534, -1.060575238724906372E-15 ) ) ;
#6771=ADVANCED_FACE ( 'NONE', ( #25009 ), #8756, .T. ) ;
#6775=CARTESIAN_POINT ( 'NONE',  ( 13.35000000000000142, 0.000000000000000000, 4.999999999999998224 ) ) ;
#6782=CARTESIAN_POINT ( 'NONE',  ( 23.10937500061451644, 0.000000000000000000, 4.756430356249998326 ) ) ;
#6787=CARTESIAN_POINT ( 'NONE',  ( 24.71250000000000213, -5.773502691896255534, -1.060575238724906372E-15 ) ) ;
#6791=CARTESIAN_POINT ( 'NONE',  ( 45.00000000000000000, 0.000000000000000000, 0.000000000000000000 ) ) ;
#6796=CARTESIAN_POINT ( 'NONE',  ( 9.018750001229033586, -5.773502691896255534, -1.060575238724906372E-15 ) ) ;
#6799=CARTESIAN_POINT ( 'NONE',  ( 18.83437500061451786, 5.492252693125287522, 3.363034840372157021E-16 ) ) ;
#6810=CARTESIAN_POINT ( 'NONE',  ( 11.25937500061451679, 2.746126346562643317, 4.756430356249998326 ) ) ;
#6817=CARTESIAN_POINT ( 'NONE',  ( 13.61250000000000071, 2.886751345948129099, -4.999999999999997335 ) ) ;
#6823=CARTESIAN_POINT ( 'NONE',  ( 10.05000000000000071, 4.330127018922192761, -2.499999999999997780 ) ) ;
#6826=ORIENTED_EDGE ( 'NONE', *, *, #48303, .F. ) ;
#6832=CARTESIAN_POINT ( 'NONE',  ( 28.95937500061451431, 0.000000000000000000, 4.756430356249998326 ) ) ;
#6834=CARTESIAN_POINT ( 'NONE',  ( 28.17187500061451289, 5.824947211148865298E-16, -4.756430356249998326 ) ) ;
#6835=CARTESIAN_POINT ( 'NONE',  ( 13.65937500061451715, 0.000000000000000000, 4.756430356249998326 ) ) ;
#6842=CARTESIAN_POINT ( 'NONE',  ( 45.00000000000000000, 6.123233995736764310E-16, -4.999999999999998224 ) ) ;
#6851=DIRECTION ( 'NONE',  ( -1.000000000000000000, -0.000000000000000000, -0.000000000000000000 ) ) ;
#6852=CARTESIAN_POINT ( 'NONE',  ( 23.11875000122903145, 2.886751345948129099, -4.999999999999998224 ) ) ;
#6854=DIRECTION ( 'NONE',  ( -1.000000000000000000, -0.000000000000000000, -0.000000000000000000 ) ) ;
#6855=ORIENTED_EDGE ( 'NONE', *, *, #59537, .F. ) ;
#6858=AXIS2_PLACEMENT_3D ( 'NONE', #13773, #36314, #58829 ) ;
#6887=CARTESIAN_POINT ( 'NONE',  ( 7.912499999999999645, 2.886751345948126879, 4.999999999999998224 ) ) ;
#6897=ORIENTED_EDGE ( 'NONE', *, *, #42828, .T. ) ;
#6900=ORIENTED_EDGE ( 'NONE', *, *, #54265, .T. ) ;
#6903=CARTESIAN_POINT ( 'NONE',  ( 18.30937500061451573, 2.746126346562645981, -4.756430356249997438 ) ) ;
#6911=DIRECTION ( 'NONE',  ( 0.000000000000000000, 0.000000000000000000, 1.000000000000000000 ) ) ;
#6912=VERTEX_POINT ( 'NONE', #64903 ) ;
#6919=LINE ( 'NONE', #29449, #18576 ) ;
#6920=CARTESIAN_POINT ( 'NONE',  ( 19.99687500061451573, -2.746126346562646425, 4.756430356249996549 ) ) ;
#6932=ORIENTED_EDGE ( 'NONE', *, *, #6481, .F. ) ;
#6942=CARTESIAN_POINT ( 'NONE',  ( 8.671875000614518214, 2.746126346562643317, 4.756430356249998326 ) ) ;
#6963=CARTESIAN_POINT ( 'NONE',  ( 27.91875000122902861, -5.773502691896255534, -1.060575238724906372E-15 ) ) ;
#6964=CARTESIAN_POINT ( 'NONE',  ( 8.296875000614516438, -2.746126346562646425, 4.756430356249996549 ) ) ;
#6965=CARTESIAN_POINT ( 'NONE',  ( 45.00000000000000000, 6.123233995736764310E-16, -4.999999999999998224 ) ) ;
#6974=CARTESIAN_POINT ( 'NONE',  ( 15.58125000122903181, 4.330127018922191873, 2.499999999999999556 ) ) ;
#6985=CARTESIAN_POINT ( 'NONE',  ( 18.08437500061451075, -2.746126346562646425, 4.756430356249996549 ) ) ;
#6988=CARTESIAN_POINT ( 'NONE',  ( 26.82187500061451502, 5.824947211148865298E-16, -4.756430356249998326 ) ) ;
#6995=CARTESIAN_POINT ( 'NONE',  ( 21.73125000122903216, 6.123233995736764310E-16, -4.999999999999998224 ) ) ;
#7002=CARTESIAN_POINT ( 'NONE',  ( 27.49687500061451217, 5.492252693125287522, 3.363034840372157021E-16 ) ) ;
#7005=CARTESIAN_POINT ( 'NONE',  ( 45.00000000000000000, 0.000000000000000000, 4.999999999999998224 ) ) ;
#7006=( BOUNDED_CURVE ( )  B_SPLINE_CURVE ( 2, ( #19775, #70761, #70399, #41240, #20136, #53777, #42326 ),
 .UNSPECIFIED., .F., .F. ) 
 B_SPLINE_CURVE_WITH_KNOTS ( ( 3, 2, 2, 3 ),
 ( 0.07999999999999998779, 0.08333333333333331483, 0.08666666666666664187, 0.08999999999999996891 ),
 .UNSPECIFIED. ) 
 CURVE ( )  GEOMETRIC_REPRESENTATION_ITEM ( )  RATIONAL_B_SPLINE_CURVE ( ( 1.000000000000000666, 0.8660254037844381525, 1.000000000000000000, 0.8660254037844387076, 1.000000000000000000, 0.8660254037844398178, 0.9999999999999988898 ) ) 
 REPRESENTATION_ITEM ( '' )  );
#7020=CARTESIAN_POINT ( 'NONE',  ( 14.18437500061451750, -4.119189519843968306, 2.378215178124996054 ) ) ;
#7045=EDGE_CURVE ( 'NONE', #27917, #71509, #35924, .T. ) ;
#7053=CARTESIAN_POINT ( 'NONE',  ( 15.72187500061451892, 2.746126346562645981, -4.756430356249997438 ) ) ;
#7060=CARTESIAN_POINT ( 'NONE',  ( 17.13749999999999929, -2.886751345948125991, -5.000000000000000000 ) ) ;
#7064=CARTESIAN_POINT ( 'NONE',  ( 23.70937500061451786, 2.746126346562645981, -4.756430356249997438 ) ) ;
#7071=CARTESIAN_POINT ( 'NONE',  ( 25.88437500061451857, -2.746126346562642428, -4.756430356249999214 ) ) ;
#7073=CARTESIAN_POINT ( 'NONE',  ( 11.59687500061451537, 4.119189519843966529, -2.378215178124998275 ) ) ;
#7081=CARTESIAN_POINT ( 'NONE',  ( 29.58749999999999858, -2.886751345948150860, 4.999999999999960920 ) ) ;
#7082=CARTESIAN_POINT ( 'NONE',  ( 15.97499999999999964, 4.330127018922191873, 2.499999999999999556 ) ) ;
#7085=CARTESIAN_POINT ( 'NONE',  ( 10.80937500061451573, 2.746126346562643317, 4.756430356249998326 ) ) ;
#7102=CARTESIAN_POINT ( 'NONE',  ( 12.09375000122903288, -2.886751345948074920, 5.000000000000092371 ) ) ;
#7104=CARTESIAN_POINT ( 'NONE',  ( 23.10937500061451644, 0.000000000000000000, 4.756430356249998326 ) ) ;
#7121=DIRECTION ( 'NONE',  ( -1.000000000000000000, -0.000000000000000000, -0.000000000000000000 ) ) ;
#7133=EDGE_CURVE ( 'NONE', #65361, #57985, #69722, .T. ) ;
#7140=CARTESIAN_POINT ( 'NONE',  ( 23.97187500061451360, 2.746126346562643317, 4.756430356249998326 ) ) ;
#7143=CARTESIAN_POINT ( 'NONE',  ( 29.28749999999999787, -2.886751345948096237, -5.000000000000050626 ) ) ;
#7145=CARTESIAN_POINT ( 'NONE',  ( 24.37500000000000000, 6.123233995736764310E-16, -4.999999999999998224 ) ) ;
#7155=CARTESIAN_POINT ( 'NONE',  ( 9.056250001229033231, -4.330127018922190985, -2.500000000000001332 ) ) ;
#7159=CARTESIAN_POINT ( 'NONE',  ( 19.20937500061451786, 2.746126346562645981, -4.756430356249997438 ) ) ;
#7171=CARTESIAN_POINT ( 'NONE',  ( 9.871875000614517504, 4.119189519843966529, 2.378215178124999607 ) ) ;
#7178=CARTESIAN_POINT ( 'NONE',  ( 19.79999999999999716, -4.330127018922190985, -2.500000000000001332 ) ) ;
#7180=CARTESIAN_POINT ( 'NONE',  ( 9.018750001229033586, -5.773502691896255534, -1.060575238724906372E-15 ) ) ;
#7184=CARTESIAN_POINT ( 'NONE',  ( 10.68750000000000000, -2.886751345948129988, 4.999999999999997335 ) ) ;
#7192=CARTESIAN_POINT ( 'NONE',  ( 28.50937500061451502, 0.000000000000000000, 4.756430356249998326 ) ) ;
#7194=CARTESIAN_POINT ( 'NONE',  ( 28.47187500061451715, -4.119189519843968306, 2.378215178124996054 ) ) ;
#7195=CARTESIAN_POINT ( 'NONE',  ( 12.15937500061451892, 4.119189519843966529, -2.378215178124998275 ) ) ;
#7201=CARTESIAN_POINT ( 'NONE',  ( 45.00000000000000000, 0.000000000000000000, 0.000000000000000000 ) ) ;
#7211=CARTESIAN_POINT ( 'NONE',  ( 22.63125000122903430, 6.123233995736764310E-16, -4.999999999999998224 ) ) ;
#7214=ORIENTED_EDGE ( 'NONE', *, *, #17788, .F. ) ;
#7219=CARTESIAN_POINT ( 'NONE',  ( 25.51875000122903003, 2.886751345948098901, 5.000000000000047073 ) ) ;
#7248=ORIENTED_EDGE ( 'NONE', *, *, #48306, .F. ) ;
#7254=CARTESIAN_POINT ( 'NONE',  ( 27.65625000122902932, 4.330127018922192761, -2.499999999999997780 ) ) ;
#7257=EDGE_LOOP ( 'NONE', ( #67652, #45941, #46966, #14399 ) ) ;
#7263=CARTESIAN_POINT ( 'NONE',  ( 17.93437500061451573, 5.492252693125287522, 3.363034840372157021E-16 ) ) ;
#7279=AXIS2_PLACEMENT_3D ( 'NONE', #70807, #42374, #18721 ) ;
#7281=CARTESIAN_POINT ( 'NONE',  ( 45.00000000000000000, 0.000000000000000000, 0.000000000000000000 ) ) ;
#7282=CARTESIAN_POINT ( 'NONE',  ( 19.35937500061451644, 4.119189519843966529, -2.378215178124998275 ) ) ;
#7303=CARTESIAN_POINT ( 'NONE',  ( 22.66875000122903216, 2.886751345948129099, -4.999999999999997335 ) ) ;
#7323=CARTESIAN_POINT ( 'NONE',  ( 17.68125000122903501, 6.123233995736764310E-16, -4.999999999999998224 ) ) ;
#7324=CARTESIAN_POINT ( 'NONE',  ( 9.346875000614517148, -2.746126346562642428, -4.756430356249999214 ) ) ;
#7344=CARTESIAN_POINT ( 'NONE',  ( 17.70937500061451786, -5.492252693125287522, -1.008910452111647106E-15 ) ) ;
#7347=CARTESIAN_POINT ( 'NONE',  ( 25.47187500061451360, 5.824947211148865298E-16, -4.756430356249998326 ) ) ;
#7362=CARTESIAN_POINT ( 'NONE',  ( 26.93437500061451573, 5.824947211148865298E-16, -4.756430356249998326 ) ) ;
#7379=CARTESIAN_POINT ( 'NONE',  ( 12.19687500061451857, 5.492252693125287522, 3.363034840372157021E-16 ) ) ;
#7394=LINE ( 'NONE', #41025, #64475 ) ;
#7411=CARTESIAN_POINT ( 'NONE',  ( 16.43437500061451573, -4.119189519843968306, 2.378215178124996054 ) ) ;
#7417=CARTESIAN_POINT ( 'NONE',  ( 16.53750000000000142, -2.886751345948129988, 4.999999999999997335 ) ) ;
#7421=CARTESIAN_POINT ( 'NONE',  ( 23.85937500061451644, 2.746126346562643317, 4.756430356249998326 ) ) ;
#7430=CARTESIAN_POINT ( 'NONE',  ( 24.64687500061451431, 4.119189519843966529, -2.378215178124998275 ) ) ;
#7432=CARTESIAN_POINT ( 'NONE',  ( 8.746875000614515727, -4.119189519843965641, -2.378215178125001383 ) ) ;
#7435=ORIENTED_EDGE ( 'NONE', *, *, #5292, .T. ) ;
#7440=DIRECTION ( 'NONE',  ( -1.000000000000000000, -0.000000000000000000, -0.000000000000000000 ) ) ;
#7442=ORIENTED_EDGE ( 'NONE', *, *, #48670, .F. ) ;
#7444=CARTESIAN_POINT ( 'NONE',  ( 12.53437500061451537, 5.492252693125287522, 3.363034840372157021E-16 ) ) ;
#7451=CARTESIAN_POINT ( 'NONE',  ( 23.66250000000000142, 2.886751345948126879, 4.999999999999998224 ) ) ;
#7459=EDGE_CURVE ( 'NONE', #42612, #59877, #43498, .T. ) ;
#7461=CARTESIAN_POINT ( 'NONE',  ( 12.24375000122902968, -2.886751345948181946, -4.999999999999904077 ) ) ;
#7463=CARTESIAN_POINT ( 'NONE',  ( 22.43437500061451573, 5.824947211148865298E-16, -4.756430356249998326 ) ) ;
#7470=ORIENTED_EDGE ( 'NONE', *, *, #8067, .F. ) ;
#7497=CARTESIAN_POINT ( 'NONE',  ( 24.34687500061451715, 5.492252693125287522, 3.363034840372157021E-16 ) ) ;
#7502=CARTESIAN_POINT ( 'NONE',  ( 24.18750000000000355, -2.886751345948129988, 4.999999999999997335 ) ) ;
#7505=CARTESIAN_POINT ( 'NONE',  ( 12.91875000122903394, 2.886751345948126879, 4.999999999999998224 ) ) ;
#7510=EDGE_CURVE ( 'NONE', #57706, #52280, #50603, .T. ) ;
#7512=CARTESIAN_POINT ( 'NONE',  ( 10.51875000122903536, 2.886751345948129099, -4.999999999999998224 ) ) ;
#7513=CARTESIAN_POINT ( 'NONE',  ( 8.887499999999995737, -2.886751345948019409, 5.000000000000189182 ) ) ;
#7515=CARTESIAN_POINT ( 'NONE',  ( 17.37187500061451573, 5.824947211148865298E-16, -4.756430356249998326 ) ) ;
#7518=ORIENTED_EDGE ( 'NONE', *, *, #5067, .T. ) ;
#7527=CARTESIAN_POINT ( 'NONE',  ( 9.459375000614519635, 2.746126346562643317, 4.756430356249998326 ) ) ;
#7533=ORIENTED_EDGE ( 'NONE', *, *, #8440, .T. ) ;
#7537=CARTESIAN_POINT ( 'NONE',  ( 27.68437500061451573, -2.746126346562642428, -4.756430356249999214 ) ) ;
#7540=CARTESIAN_POINT ( 'NONE',  ( 8.812500000000000000, 2.886751345948126879, 4.999999999999999112 ) ) ;
#7543=ORIENTED_EDGE ( 'NONE', *, *, #17037, .F. ) ;
#7548=CARTESIAN_POINT ( 'NONE',  ( 29.52187500061451431, -5.492252693125287522, -1.008910452111647106E-15 ) ) ;
#7550=CARTESIAN_POINT ( 'NONE',  ( 27.42187500061451289, 4.119189519843966529, 2.378215178124999607 ) ) ;
#7551=CARTESIAN_POINT ( 'NONE',  ( 9.946875000614516793, 5.492252693125287522, 3.363034840372157021E-16 ) ) ;
#7566=CARTESIAN_POINT ( 'NONE',  ( 23.49375000122903145, -2.886751345948125991, -5.000000000000000000 ) ) ;
#7591=CARTESIAN_POINT ( 'NONE',  ( 45.00000000000000000, 0.000000000000000000, 0.000000000000000000 ) ) ;
#7613=ADVANCED_FACE ( 'NONE', ( #29295 ), #35191, .T. ) ;
#7618=CARTESIAN_POINT ( 'NONE',  ( 15.53437500061451360, -2.746126346562642428, -4.756430356249999214 ) ) ;
#7635=CARTESIAN_POINT ( 'NONE',  ( 8.381250001229034297, 4.330127018922191873, 2.499999999999999556 ) ) ;
#7637=DIRECTION ( 'NONE',  ( 0.000000000000000000, 0.000000000000000000, 1.000000000000000000 ) ) ;
#7638=CARTESIAN_POINT ( 'NONE',  ( 17.97187500061451715, 2.746126346562645981, -4.756430356249997438 ) ) ;
#7648=CYLINDRICAL_SURFACE ( 'NONE', #66672, 4.999999999999998224 ) ;
#7658=AXIS2_PLACEMENT_3D ( 'NONE', #10070, #15960, #55499 ) ;
#7670=AXIS2_PLACEMENT_3D ( 'NONE', #1717, #24229, #53774 ) ;
#7684=CARTESIAN_POINT ( 'NONE',  ( 29.88749999999999929, 5.773502691896255534, 3.535250795749688894E-16 ) ) ;
#7689=CYLINDRICAL_SURFACE ( 'NONE', #53791, 4.999999999999998224 ) ;
#7692=DIRECTION ( 'NONE',  ( 0.000000000000000000, 0.000000000000000000, 1.000000000000000000 ) ) ;
#7703=VECTOR ( 'NONE', #36777, 1000.000000000000000 ) ;
#7704=CARTESIAN_POINT ( 'NONE',  ( 15.15937500061451537, 2.746126346562645981, -4.756430356249997438 ) ) ;
#7708=CARTESIAN_POINT ( 'NONE',  ( 24.49687500061451573, -4.119189519843965641, -2.378215178125001383 ) ) ;
#7716=CARTESIAN_POINT ( 'NONE',  ( 28.18125000122903145, 4.330127018922191873, 2.499999999999999556 ) ) ;
#7724=CARTESIAN_POINT ( 'NONE',  ( 27.79687500061451999, -2.746126346562642428, -4.756430356249999214 ) ) ;
#7733=EDGE_LOOP ( 'NONE', ( #39629, #49268, #24959, #39725 ) ) ;
#7742=CARTESIAN_POINT ( 'NONE',  ( 12.94687500061451857, -2.746126346562641984, -4.756430356249999214 ) ) ;
#7753=VECTOR ( 'NONE', #20551, 1000.000000000000000 ) ;
#7776=CARTESIAN_POINT ( 'NONE',  ( 13.50937500061451679, 4.119189519843966529, -2.378215178124998275 ) ) ;
#7781=CARTESIAN_POINT ( 'NONE',  ( 17.39999999999999858, 0.000000000000000000, 4.999999999999998224 ) ) ;
#7785=CARTESIAN_POINT ( 'NONE',  ( 22.95937500061451786, 2.746126346562643317, 4.756430356249998326 ) ) ;
#7793=CARTESIAN_POINT ( 'NONE',  ( 21.60937500061451644, 2.746126346562643317, 4.756430356249998326 ) ) ;
#7795=CARTESIAN_POINT ( 'NONE',  ( 8.221875000614515372, -4.119189519843968306, 2.378215178124996054 ) ) ;
#7805=PLANE ( 'NONE',  #3224 ) ;
#7808=CARTESIAN_POINT ( 'NONE',  ( 12.38437500061451502, -2.746126346562642428, -4.756430356249999214 ) ) ;
#7816=CARTESIAN_POINT ( 'NONE',  ( 45.00000000000000000, 6.123233995736764310E-16, -4.999999999999998224 ) ) ;
#7820=VERTEX_POINT ( 'NONE', #49814 ) ;
#7829=CARTESIAN_POINT ( 'NONE',  ( 18.42187500061451999, 2.746126346562645981, -4.756430356249997438 ) ) ;
#7843=ORIENTED_EDGE ( 'NONE', *, *, #17293, .T. ) ;
#7859=ORIENTED_EDGE ( 'NONE', *, *, #39854, .T. ) ;
#7863=CARTESIAN_POINT ( 'NONE',  ( 22.88437500061451857, 5.824947211148865298E-16, -4.756430356249998326 ) ) ;
#7869=CARTESIAN_POINT ( 'NONE',  ( 24.78750000000000497, -2.886751345948125991, -5.000000000000000000 ) ) ;
#7872=CARTESIAN_POINT ( 'NONE',  ( 9.975000000000001421, 6.123233995736764310E-16, -4.999999999999998224 ) ) ;
#7873=DIRECTION ( 'NONE',  ( -1.000000000000000000, -0.000000000000000000, -0.000000000000000000 ) ) ;
#7874=CARTESIAN_POINT ( 'NONE',  ( 45.00000000000000000, 0.000000000000000000, 0.000000000000000000 ) ) ;
#7880=CARTESIAN_POINT ( 'NONE',  ( 9.506250001229030744, -4.330127018922190985, -2.500000000000001332 ) ) ;
#7882=CARTESIAN_POINT ( 'NONE',  ( 15.83437500061451253, -2.746126346562646425, 4.756430356249996549 ) ) ;
#7893=CARTESIAN_POINT ( 'NONE',  ( 9.609375000614514661, -5.492252693125287522, -1.008910452111647106E-15 ) ) ;
#7894=ORIENTED_EDGE ( 'NONE', *, *, #37794, .F. ) ;
#7903=CARTESIAN_POINT ( 'NONE',  ( 29.22187500061451360, 4.119189519843966529, 2.378215178124999607 ) ) ;
#7906=CARTESIAN_POINT ( 'NONE',  ( 8.137500000000002842, -2.886751345948125991, -5.000000000000000000 ) ) ;
#7915=CARTESIAN_POINT ( 'NONE',  ( 26.29687500061451644, -2.746126346562646425, 4.756430356249996549 ) ) ;
#7917=CARTESIAN_POINT ( 'NONE',  ( 11.48437500061451644, -4.119189519843968306, 2.378215178124996054 ) ) ;
#7932=CARTESIAN_POINT ( 'NONE',  ( 20.56875000122903785, 2.886751345948126879, 4.999999999999999112 ) ) ;
#7935=ORIENTED_EDGE ( 'NONE', *, *, #31576, .T. ) ;
#7958=DIRECTION ( 'NONE',  ( 0.000000000000000000, 0.000000000000000000, 1.000000000000000000 ) ) ;
#7959=EDGE_CURVE ( 'NONE', #65810, #68516, #63056, .T. ) ;
#7967=CARTESIAN_POINT ( 'NONE',  ( 19.03125000122902932, 6.123233995736764310E-16, -4.999999999999998224 ) ) ;
#7968=CARTESIAN_POINT ( 'NONE',  ( 16.33125000122903359, 6.123233995736764310E-16, -4.999999999999998224 ) ) ;
#7983=VERTEX_POINT ( 'NONE', #17264 ) ;
#7987=CARTESIAN_POINT ( 'NONE',  ( 16.77187500061451431, -4.119189519843968306, 2.378215178124996054 ) ) ;
#8003=CARTESIAN_POINT ( 'NONE',  ( 9.768750001229031810, 2.886751345948126879, 4.999999999999998224 ) ) ;
#8004=CYLINDRICAL_SURFACE ( 'NONE', #54001, 4.999999999999998224 ) ;
#8007=CARTESIAN_POINT ( 'NONE',  ( 18.53437500061451715, 4.119189519843966529, 2.378215178124999607 ) ) ;
#8020=CARTESIAN_POINT ( 'NONE',  ( 13.91250000000000142, -5.773502691896255534, -1.060575238724906372E-15 ) ) ;
#8024=CARTESIAN_POINT ( 'NONE',  ( 27.84375000122903288, -2.886751345948129988, 4.999999999999997335 ) ) ;
#8028=DIRECTION ( 'NONE',  ( -1.000000000000000000, -0.000000000000000000, -0.000000000000000000 ) ) ;
#8046=ADVANCED_FACE ( 'NONE', ( #51260 ), #51627, .T. ) ;
#8050=CARTESIAN_POINT ( 'NONE',  ( 17.68125000122903501, 6.123233995736764310E-16, -4.999999999999998224 ) ) ;
#8051=CARTESIAN_POINT ( 'NONE',  ( 29.96250000000000213, 2.886751345948126879, 4.999999999999999112 ) ) ;
#8060=CARTESIAN_POINT ( 'NONE',  ( 15.50625000122903430, 4.330127018922192761, -2.499999999999997780 ) ) ;
#8067=EDGE_CURVE ( 'NONE', #48464, #34596, #6919, .T. ) ;
#8071=CARTESIAN_POINT ( 'NONE',  ( 14.74687500061451573, 4.119189519843966529, -2.378215178124998275 ) ) ;
#8074=CARTESIAN_POINT ( 'NONE',  ( 22.58437500061451786, -2.746126346562646425, 4.756430356249996549 ) ) ;
#8081=CARTESIAN_POINT ( 'NONE',  ( 23.68125000122903145, 4.330127018922191873, 2.499999999999999556 ) ) ;
#8082=EDGE_CURVE ( 'NONE', #67338, #70443, #65705, .T. ) ;
#8090=CARTESIAN_POINT ( 'NONE',  ( 23.93437500061451573, 4.119189519843966529, 2.378215178124999607 ) ) ;
#8110=CARTESIAN_POINT ( 'NONE',  ( 12.45937500061451786, -4.119189519843965641, -2.378215178125001383 ) ) ;
#8125=VERTEX_POINT ( 'NONE', #39092 ) ;
#8141=CARTESIAN_POINT ( 'NONE',  ( 13.92187500061451644, 2.746126346562645981, -4.756430356249997438 ) ) ;
#8147=CARTESIAN_POINT ( 'NONE',  ( 14.88750000000000107, -2.886751345948125991, -5.000000000000000000 ) ) ;
#8150=CARTESIAN_POINT ( 'NONE',  ( 24.67500000000000071, -4.330127018922194537, 2.499999999999995559 ) ) ;
#8151=CARTESIAN_POINT ( 'NONE',  ( 22.99687500061451573, 0.000000000000000000, 4.756430356249998326 ) ) ;
#8152=ORIENTED_EDGE ( 'NONE', *, *, #60122, .T. ) ;
#8154=FACE_OUTER_BOUND ( 'NONE', #69900, .T. ) ;
#8158=CARTESIAN_POINT ( 'NONE',  ( 22.17187500061451644, -4.119189519843968306, 2.378215178124996054 ) ) ;
#8160=CARTESIAN_POINT ( 'NONE',  ( 7.959375000614516971, 2.746126346562645981, -4.756430356249997438 ) ) ;
#8171=CARTESIAN_POINT ( 'NONE',  ( 8.484375000614518214, 5.492252693125287522, 3.363034840372157021E-16 ) ) ;
#8191=CARTESIAN_POINT ( 'NONE',  ( 14.15625000122903288, 4.330127018922192761, -2.499999999999997780 ) ) ;
#8194=CARTESIAN_POINT ( 'NONE',  ( 19.39687500061451786, 5.492252693125287522, 3.363034840372157021E-16 ) ) ;
#8217=ADVANCED_FACE ( 'NONE', ( #40540 ), #33531, .T. ) ;
#8221=FACE_OUTER_BOUND ( 'NONE', #62873, .T. ) ;
#8224=EDGE_CURVE ( 'NONE', #68516, #44765, #15645, .T. ) ;
#8225=VERTEX_POINT ( 'NONE', #58230 ) ;
#8229=CARTESIAN_POINT ( 'NONE',  ( 20.78437500061451715, 4.119189519843966529, 2.378215178124999607 ) ) ;
#8234=CARTESIAN_POINT ( 'NONE',  ( 24.48749999999999716, 5.773502691896255534, 3.535250795749688894E-16 ) ) ;
#8237=DIRECTION ( 'NONE',  ( -1.000000000000000000, -0.000000000000000000, -0.000000000000000000 ) ) ;
#8238=PLANE ( 'NONE',  #60689 ) ;
#8240=CARTESIAN_POINT ( 'NONE',  ( 18.80625000122903501, 0.000000000000000000, 4.999999999999998224 ) ) ;
#8245=CARTESIAN_POINT ( 'NONE',  ( 29.33437500061451431, -2.746126346562646425, 4.756430356249996549 ) ) ;
#8247=CARTESIAN_POINT ( 'NONE',  ( 15.38437500061451679, -2.746126346562646425, 4.756430356249996549 ) ) ;
#8259=CARTESIAN_POINT ( 'NONE',  ( 8.446875000614515017, 4.119189519843966529, -2.378215178124998275 ) ) ;
#8265=ORIENTED_EDGE ( 'NONE', *, *, #163, .T. ) ;
#8266=CARTESIAN_POINT ( 'NONE',  ( 10.27499999999999858, -4.330127018922194537, 2.499999999999995559 ) ) ;
#8270=CARTESIAN_POINT ( 'NONE',  ( 29.40937500061451360, -5.492252693125287522, -1.008910452111647106E-15 ) ) ;
#8273=CARTESIAN_POINT ( 'NONE',  ( 9.337500000000000355, -2.886751345948129988, 4.999999999999997335 ) ) ;
#8280=CARTESIAN_POINT ( 'NONE',  ( 26.48437500061451644, 5.824947211148865298E-16, -4.756430356249998326 ) ) ;
#8282=CARTESIAN_POINT ( 'NONE',  ( 10.09687500061451715, -2.746126346562646425, 4.756430356249996549 ) ) ;
#8290=DIRECTION ( 'NONE',  ( -1.000000000000000000, -0.000000000000000000, -0.000000000000000000 ) ) ;
#8294=PRESENTATION_STYLE_ASSIGNMENT (( #58884 ) ) ;
#8299=CARTESIAN_POINT ( 'NONE',  ( 21.91875000122902861, 2.886751345948126879, 4.999999999999999112 ) ) ;
#8302=VERTEX_POINT ( 'NONE', #18703 ) ;
#8310=EDGE_CURVE ( 'NONE', #50518, #31702, #36444, .T. ) ;
#8315=CARTESIAN_POINT ( 'NONE',  ( 27.90937500061451715, 4.119189519843966529, -2.378215178124998275 ) ) ;
#8339=CARTESIAN_POINT ( 'NONE',  ( 8.625000000000000000, 6.123233995736764310E-16, -4.999999999999998224 ) ) ;
#8349=CARTESIAN_POINT ( 'NONE',  ( 17.25937500061451502, -5.492252693125287522, -1.008910452111647106E-15 ) ) ;
#8358=ORIENTED_EDGE ( 'NONE', *, *, #44624, .F. ) ;
#8364=CARTESIAN_POINT ( 'NONE',  ( 25.89375000122903003, 5.773502691896255534, 3.535250795749688401E-16 ) ) ;
#8365=CARTESIAN_POINT ( 'NONE',  ( 9.581250001229033586, 6.123233995736764310E-16, -4.999999999999998224 ) ) ;
#8369=CARTESIAN_POINT ( 'NONE',  ( 16.54687500061451644, -2.746126346562642428, -4.756430356249999214 ) ) ;
#8382=CARTESIAN_POINT ( 'NONE',  ( 13.98750000000000071, -2.886751345948237457, -4.999999999999807265 ) ) ;
#8387=CARTESIAN_POINT ( 'NONE',  ( 27.73125000122902861, 4.330127018922191873, 2.499999999999999556 ) ) ;
#8410=CARTESIAN_POINT ( 'NONE',  ( 7.584375000614516082, 5.824947211148865298E-16, -4.756430356249998326 ) ) ;
#8416=CARTESIAN_POINT ( 'NONE',  ( 11.88749999999999929, 5.773502691896255534, 3.535250795749688401E-16 ) ) ;
#8427=ADVANCED_FACE ( 'NONE', ( #64142 ), #41623, .T. ) ;
#8428=CARTESIAN_POINT ( 'NONE',  ( 15.49687500061451573, -4.119189519843965641, -2.378215178125001383 ) ) ;
#8431=CARTESIAN_POINT ( 'NONE',  ( 22.65937500061451360, -5.492252693125287522, -1.008910452111647106E-15 ) ) ;
#8440=EDGE_CURVE ( 'NONE', #24521, #8998, #53806, .T. ) ;
#8442=CYLINDRICAL_SURFACE ( 'NONE', #6568, 4.999999999999998224 ) ;
#8449=CARTESIAN_POINT ( 'NONE',  ( 23.89687500061451786, 5.492252693125287522, 3.363034840372157021E-16 ) ) ;
#8461=VERTEX_POINT ( 'NONE', #42357 ) ;
#8470=CARTESIAN_POINT ( 'NONE',  ( 12.23437500061451821, 4.119189519843966529, 2.378215178124999607 ) ) ;
#8483=ORIENTED_EDGE ( 'NONE', *, *, #5952, .T. ) ;
#8487=CARTESIAN_POINT ( 'NONE',  ( 14.83125000122903359, -4.330127018922194537, 2.499999999999995559 ) ) ;
#8491=EDGE_CURVE ( 'NONE', #27766, #65361, #23196, .T. ) ;
#8496=EDGE_LOOP ( 'NONE', ( #61068, #1007, #39447, #48879 ) ) ;
#8500=PRODUCT_DEFINITION_CONTEXT ( 'detailed design', #62028, 'design' ) ;
#8501=CARTESIAN_POINT ( 'NONE',  ( 13.43437500061451750, 5.824947211148865298E-16, -4.756430356249998326 ) ) ;
#8509=CARTESIAN_POINT ( 'NONE',  ( 15.86250000000000249, 2.886751345948129099, -4.999999999999998224 ) ) ;
#8512=CYLINDRICAL_SURFACE ( 'NONE', #25320, 4.999999999999998224 ) ;
#8514=CARTESIAN_POINT ( 'NONE',  ( 15.71250000000000036, -5.773502691896255534, -1.060575238724906372E-15 ) ) ;
#8522=CARTESIAN_POINT ( 'NONE',  ( 23.18437500061451217, -2.746126346562642428, -4.756430356249999214 ) ) ;
#8524=CARTESIAN_POINT ( 'NONE',  ( 8.634375000614515017, -2.746126346562646425, 4.756430356249996549 ) ) ;
#8528=CARTESIAN_POINT ( 'NONE',  ( 9.881250001229032520, -4.330127018922194537, 2.499999999999995559 ) ) ;
#8535=CARTESIAN_POINT ( 'NONE',  ( 8.184375000614515727, -2.746126346562646425, 4.756430356249996549 ) ) ;
#8546=( BOUNDED_CURVE ( )  B_SPLINE_CURVE ( 2, ( #14109, #37747, #48478, #65453, #71746, #65825, #36648 ),
 .UNSPECIFIED., .F., .F. ) 
 B_SPLINE_CURVE_WITH_KNOTS ( ( 3, 2, 2, 3 ),
 ( 0.4000000000000000777, 0.4033333333333333215, 0.4066666666666666763, 0.4099999999999999201 ),
 .UNSPECIFIED. ) 
 CURVE ( )  GEOMETRIC_REPRESENTATION_ITEM ( )  RATIONAL_B_SPLINE_CURVE ( ( 0.9999999999999977796, 0.8660254037844409281, 1.000000000000000000, 0.8660254037844387076, 1.000000000000000000, 0.8660254037844409281, 0.9999999999999977796 ) ) 
 REPRESENTATION_ITEM ( '' )  );
#8548=ORIENTED_EDGE ( 'NONE', *, *, #17032, .T. ) ;
#8559=CARTESIAN_POINT ( 'NONE',  ( 18.68437500061451928, -4.119189519843968306, 2.378215178124996054 ) ) ;
#8587=ORIENTED_EDGE ( 'NONE', *, *, #54635, .F. ) ;
#8591=CARTESIAN_POINT ( 'NONE',  ( 22.02187500061452141, 2.746126346562645981, -4.756430356249997438 ) ) ;
#8598=CARTESIAN_POINT ( 'NONE',  ( 23.36250000000000071, -5.773502691896255534, -1.060575238724906372E-15 ) ) ;
#8601=CARTESIAN_POINT ( 'NONE',  ( 45.00000000000000000, 0.000000000000000000, 4.999999999999998224 ) ) ;
#8602=CARTESIAN_POINT ( 'NONE',  ( 34.99999999999999289, -2.499999999999999556, -3.499999999999999556 ) ) ;
#8608=CARTESIAN_POINT ( 'NONE',  ( 7.518750001229031810, 2.886751345948126879, 4.999999999999999112 ) ) ;
#8610=CARTESIAN_POINT ( 'NONE',  ( 14.82187500061451502, 4.119189519843966529, 2.378215178124999607 ) ) ;
#8620=CARTESIAN_POINT ( 'NONE',  ( 18.75000000000000000, 0.000000000000000000, 4.999999999999998224 ) ) ;
#8621=CARTESIAN_POINT ( 'NONE',  ( 8.521875000614517859, 4.119189519843966529, 2.378215178124999607 ) ) ;
#8630=CARTESIAN_POINT ( 'NONE',  ( 19.81875000122903430, -5.773502691896255534, -1.060575238724906372E-15 ) ) ;
#8632=CARTESIAN_POINT ( 'NONE',  ( 28.39687500061451431, 0.000000000000000000, 4.756430356249998326 ) ) ;
#8636=CARTESIAN_POINT ( 'NONE',  ( 9.375000000000001776, -4.330127018922194537, 2.499999999999995559 ) ) ;
#8643=CARTESIAN_POINT ( 'NONE',  ( 26.97187500061451004, 2.746126346562645981, -4.756430356249997438 ) ) ;
#8645=CARTESIAN_POINT ( 'NONE',  ( 10.24687500061451750, -2.746126346562642428, -4.756430356249999214 ) ) ;
#8663=CARTESIAN_POINT ( 'NONE',  ( 20.19375000122903430, -2.886751345948129988, 4.999999999999997335 ) ) ;
#8678=CARTESIAN_POINT ( 'NONE',  ( 27.57187500061451857, 2.746126346562643317, 4.756430356249998326 ) ) ;
#8691=EDGE_CURVE ( 'NONE', #55926, #41736, #19804, .T. ) ;
#8696=CARTESIAN_POINT ( 'NONE',  ( 16.36875000122903145, 2.886751345948129099, -4.999999999999997335 ) ) ;
#8710=ADVANCED_FACE ( 'NONE', ( #19431 ), #8004, .T. ) ;
#8712=DIRECTION ( 'NONE',  ( -1.000000000000000000, 0.000000000000000000, 0.000000000000000000 ) ) ;
#8715=CARTESIAN_POINT ( 'NONE',  ( 16.43437500061451573, -2.746126346562642428, -4.756430356249999214 ) ) ;
#8728=CARTESIAN_POINT ( 'NONE',  ( 16.35000000000000142, 4.330127018922192761, -2.499999999999997780 ) ) ;
#8729=LINE ( 'NONE', #47528, #64291 ) ;
#8733=CARTESIAN_POINT ( 'NONE',  ( 17.74687500061451928, -2.746126346562646425, 4.756430356249996549 ) ) ;
#8743=( BOUNDED_CURVE ( )  B_SPLINE_CURVE ( 2, ( #53138, #37974, #36878, #9175, #30972, #43164, #47600 ),
 .UNSPECIFIED., .F., .F. ) 
 B_SPLINE_CURVE_WITH_KNOTS ( ( 3, 2, 2, 3 ),
 ( 0.2600000000000000644, 0.2633333333333333637, 0.2666666666666667185, 0.2700000000000000733 ),
 .UNSPECIFIED. ) 
 CURVE ( )  GEOMETRIC_REPRESENTATION_ITEM ( )  RATIONAL_B_SPLINE_CURVE ( ( 0.9999999999999977796, 0.8660254037844409281, 1.000000000000000000, 0.8660254037844387076, 1.000000000000000000, 0.8660254037844364872, 1.000000000000002220 ) ) 
 REPRESENTATION_ITEM ( '' )  );
#8753=CARTESIAN_POINT ( 'NONE',  ( 28.55625000122903145, 4.330127018922192761, -2.499999999999997780 ) ) ;
#8756=CYLINDRICAL_SURFACE ( 'NONE', #72873, 4.999999999999998224 ) ;
#8757=CARTESIAN_POINT ( 'NONE',  ( 8.362500000000002487, 2.886751345948126879, 4.999999999999998224 ) ) ;
#8765=VECTOR ( 'NONE', #61298, 1000.000000000000000 ) ;
#8778=CARTESIAN_POINT ( 'NONE',  ( 28.38749999999999929, -2.886751345948125991, -5.000000000000000000 ) ) ;
#8784=CARTESIAN_POINT ( 'NONE',  ( 11.84999999999999964, 4.330127018922192761, -2.499999999999997780 ) ) ;
#8789=ADVANCED_FACE ( 'NONE', ( #6126 ), #29385, .T. ) ;
#8798=CARTESIAN_POINT ( 'NONE',  ( 14.52187500061451608, -4.119189519843968306, 2.378215178124996054 ) ) ;
#8801=CARTESIAN_POINT ( 'NONE',  ( 23.18437500061451217, -2.746126346562642428, -4.756430356249999214 ) ) ;
#8806=CARTESIAN_POINT ( 'NONE',  ( 15.52500000000000036, 4.330127018922191873, 2.499999999999999556 ) ) ;
#8810=CARTESIAN_POINT ( 'NONE',  ( 23.53125000122902932, 6.123233995736764310E-16, -4.999999999999998224 ) ) ;
#8811=CARTESIAN_POINT ( 'NONE',  ( 13.68750000000000178, 5.773502691896255534, 3.535250795749688894E-16 ) ) ;
#8818=CARTESIAN_POINT ( 'NONE',  ( 25.20937500061451431, 4.119189519843966529, -2.378215178124998275 ) ) ;
#8839=CARTESIAN_POINT ( 'NONE',  ( 13.50937500061451679, 4.119189519843966529, -2.378215178124998275 ) ) ;
#8853=EDGE_LOOP ( 'NONE', ( #41532, #34454, #58473, #17243 ) ) ;
#8865=EDGE_CURVE ( 'NONE', #24022, #6086, #22744, .T. ) ;
#8868=CARTESIAN_POINT ( 'NONE',  ( 14.10937500061451644, 0.000000000000000000, 4.756430356249998326 ) ) ;
#8872=VECTOR ( 'NONE', #17167, 1000.000000000000000 ) ;
#8878=CARTESIAN_POINT ( 'NONE',  ( 14.47499999999999964, 6.123233995736764310E-16, -4.999999999999998224 ) ) ;
#8883=EDGE_CURVE ( 'NONE', #1580, #40669, #39029, .T. ) ;
#8893=CARTESIAN_POINT ( 'NONE',  ( 22.65937500061451360, -5.492252693125287522, -1.008910452111647106E-15 ) ) ;
#8895=CARTESIAN_POINT ( 'NONE',  ( 8.146875000614516082, 0.000000000000000000, 4.756430356249998326 ) ) ;
#8907=CARTESIAN_POINT ( 'NONE',  ( 8.971875000614515372, 4.119189519843966529, 2.378215178124999607 ) ) ;
#8930=CARTESIAN_POINT ( 'NONE',  ( 19.80937500061451573, 4.119189519843966529, -2.378215178124998275 ) ) ;
#8951=( BOUNDED_CURVE ( )  B_SPLINE_CURVE ( 2, ( #38234, #71867, #60764, #65210, #27167, #44162, #59664 ),
 .UNSPECIFIED., .F., .F. ) 
 B_SPLINE_CURVE_WITH_KNOTS ( ( 3, 2, 2, 3 ),
 ( 0.8399999999999999689, 0.8433333333333334902, 0.8466666666666667895, 0.8500000000000001998 ),
 .UNSPECIFIED. ) 
 CURVE ( )  GEOMETRIC_REPRESENTATION_ITEM ( )  RATIONAL_B_SPLINE_CURVE ( ( 1.000000000000000000, 0.8660254037844387076, 1.000000000000000000, 0.8660254037844387076, 1.000000000000000000, 0.8660254037844298258, 1.000000000000008882 ) ) 
 REPRESENTATION_ITEM ( '' )  );
#8962=CARTESIAN_POINT ( 'NONE',  ( 20.18437500061451573, 5.824947211148865298E-16, -4.756430356249998326 ) ) ;
#8967=( BOUNDED_CURVE ( )  B_SPLINE_CURVE ( 2, ( #23792, #41170, #7178, #45981, #51527, #58127, #34519 ),
 .UNSPECIFIED., .F., .F. ) 
 B_SPLINE_CURVE_WITH_KNOTS ( ( 3, 2, 2, 3 ),
 ( 0.4500000000000000111, 0.4533333333333333104, 0.4566666666666666652, 0.4600000000000000200 ),
 .UNSPECIFIED. ) 
 CURVE ( )  GEOMETRIC_REPRESENTATION_ITEM ( )  RATIONAL_B_SPLINE_CURVE ( ( 1.000000000000000000, 0.8660254037844387076, 1.000000000000000000, 0.8660254037844387076, 1.000000000000000000, 0.8660254037844387076, 1.000000000000000000 ) ) 
 REPRESENTATION_ITEM ( '' )  );
#8970=CARTESIAN_POINT ( 'NONE',  ( 21.44999999999999929, 0.000000000000000000, 4.999999999999998224 ) ) ;
#8975=FACE_OUTER_BOUND ( 'NONE', #45703, .T. ) ;
#8978=CARTESIAN_POINT ( 'NONE',  ( 18.28125000122903288, 4.330127018922191873, 2.499999999999999556 ) ) ;
#8980=CARTESIAN_POINT ( 'NONE',  ( 7.106250001229032165, 0.000000000000000000, 4.999999999999998224 ) ) ;
#8983=CARTESIAN_POINT ( 'NONE',  ( 15.49687500061451573, -4.119189519843965641, -2.378215178125001383 ) ) ;
#8989=CARTESIAN_POINT ( 'NONE',  ( 17.08125000122903003, -4.330127018922194537, 2.499999999999995559 ) ) ;
#8993=CARTESIAN_POINT ( 'NONE',  ( 8.071875000614515017, 4.119189519843966529, 2.378215178124999607 ) ) ;
#8998=VERTEX_POINT ( 'NONE', #39762 ) ;
#9004=CARTESIAN_POINT ( 'NONE',  ( 27.64687500061451431, -4.119189519843965641, -2.378215178125001383 ) ) ;
#9017=CARTESIAN_POINT ( 'NONE',  ( 26.07187500061451502, 2.746126346562645981, -4.756430356249997438 ) ) ;
#9019=CARTESIAN_POINT ( 'NONE',  ( 9.384375000614518569, 5.824947211148865298E-16, -4.756430356249998326 ) ) ;
#9036=CARTESIAN_POINT ( 'NONE',  ( 20.11875000122903145, 2.886751345948126879, 4.999999999999999112 ) ) ;
#9051=CARTESIAN_POINT ( 'NONE',  ( 27.42187500061451644, 2.746126346562645981, -4.756430356249997438 ) ) ;
#9079=ORIENTED_EDGE ( 'NONE', *, *, #15629, .T. ) ;
#9083=CARTESIAN_POINT ( 'NONE',  ( 11.73750000000000071, -2.886751345948126435, -5.000000000000000000 ) ) ;
#9086=CARTESIAN_POINT ( 'NONE',  ( 17.67187500061451644, -4.119189519843968306, 2.378215178124996054 ) ) ;
#9094=VERTEX_POINT ( 'NONE', #12574 ) ;
#9097=CARTESIAN_POINT ( 'NONE',  ( 45.00000000000000000, 6.123233995736764310E-16, -4.999999999999998224 ) ) ;
#9101=DIRECTION ( 'NONE',  ( -1.000000000000000000, -0.000000000000000000, -0.000000000000000000 ) ) ;
#9104=LINE ( 'NONE', #32002, #27709 ) ;
#9105=CARTESIAN_POINT ( 'NONE',  ( 18.72187500061451360, -5.492252693125287522, -1.008910452111647106E-15 ) ) ;
#9118=CARTESIAN_POINT ( 'NONE',  ( 21.65625000122903288, -4.330127018922190985, -2.500000000000001332 ) ) ;
#9122=CARTESIAN_POINT ( 'NONE',  ( 29.26875000122903003, -5.773502691896255534, -1.060575238724906372E-15 ) ) ;
#9124=CYLINDRICAL_SURFACE ( 'NONE', #21880, 4.999999999999998224 ) ;
#9134=VERTEX_POINT ( 'NONE', #36198 ) ;
#9148=CARTESIAN_POINT ( 'NONE',  ( 7.696875000614516793, 5.492252693125287522, 3.363034840372157021E-16 ) ) ;
#9156=CARTESIAN_POINT ( 'NONE',  ( 9.281250001229032875, 4.330127018922191873, 2.499999999999999556 ) ) ;
#9157=CARTESIAN_POINT ( 'NONE',  ( 22.34999999999999787, 0.000000000000000000, 4.999999999999998224 ) ) ;
#9164=( BOUNDED_CURVE ( )  B_SPLINE_CURVE ( 2, ( #68854, #6068, #1624, #29683, #18581, #13045, #35584 ),
 .UNSPECIFIED., .F., .F. ) 
 B_SPLINE_CURVE_WITH_KNOTS ( ( 3, 2, 2, 3 ),
 ( 0.6500000000000000222, 0.6533333333333333215, 0.6566666666666666208, 0.6600000000000000311 ),
 .UNSPECIFIED. ) 
 CURVE ( )  GEOMETRIC_REPRESENTATION_ITEM ( )  RATIONAL_B_SPLINE_CURVE ( ( 1.000000000000000000, 0.8660254037844387076, 1.000000000000000000, 0.8660254037844387076, 1.000000000000000000, 0.8660254037844387076, 1.000000000000000000 ) ) 
 REPRESENTATION_ITEM ( '' )  );
#9166=CARTESIAN_POINT ( 'NONE',  ( 16.35937500061451644, -5.492252693125287522, -1.008910452111647106E-15 ) ) ;
#9170=CARTESIAN_POINT ( 'NONE',  ( 23.10937500061451644, -5.492252693125287522, -1.008910452111647106E-15 ) ) ;
#9175=CARTESIAN_POINT ( 'NONE',  ( 24.03750000000000142, 5.773502691896255534, 3.535250795749688401E-16 ) ) ;
#9180=CARTESIAN_POINT ( 'NONE',  ( 13.87500000000000178, -4.330127018922194537, 2.499999999999995559 ) ) ;
#9187=CARTESIAN_POINT ( 'NONE',  ( 25.92187500061451999, -5.492252693125287522, -1.008910452111647106E-15 ) ) ;
#9190=CARTESIAN_POINT ( 'NONE',  ( 15.82499999999999929, 6.123233995736764310E-16, -4.999999999999998224 ) ) ;
#9208=CARTESIAN_POINT ( 'NONE',  ( 8.859375000614518214, -4.119189519843965641, -2.378215178125001383 ) ) ;
#9221=ORIENTED_EDGE ( 'NONE', *, *, #49500, .T. ) ;
#9225=CARTESIAN_POINT ( 'NONE',  ( 14.79375000122903039, -2.886751345948130876, 4.999999999999996447 ) ) ;
#9229=VECTOR ( 'NONE', #24853, 1000.000000000000000 ) ;
#9238=CARTESIAN_POINT ( 'NONE',  ( 13.05937500061451750, 4.119189519843966529, -2.378215178124998275 ) ) ;
#9246=CARTESIAN_POINT ( 'NONE',  ( 16.12500000000000000, -4.330127018922194537, 2.499999999999995559 ) ) ;
#9249=DIRECTION ( 'NONE',  ( -1.000000000000000000, -0.000000000000000000, -0.000000000000000000 ) ) ;
#9256=LINE ( 'NONE', #37685, #36734 ) ;
#9258=CARTESIAN_POINT ( 'NONE',  ( 21.68437500061451573, -2.746126346562646425, 4.756430356249996549 ) ) ;
#9269=CARTESIAN_POINT ( 'NONE',  ( 10.01250000000000107, 2.886751345948129099, -4.999999999999997335 ) ) ;
#9271=CARTESIAN_POINT ( 'NONE',  ( 8.746875000614515727, -4.119189519843965641, -2.378215178125001383 ) ) ;
#9282=EDGE_CURVE ( 'NONE', #8125, #8998, #10487, .T. ) ;
#9295=CARTESIAN_POINT ( 'NONE',  ( 20.14687500061451786, -2.746126346562641984, -4.756430356249999214 ) ) ;
#9328=CARTESIAN_POINT ( 'NONE',  ( 22.17187500061451644, 2.746126346562643317, 4.756430356249998326 ) ) ;
#9332=( BOUNDED_CURVE ( )  B_SPLINE_CURVE ( 2, ( #5890, #55052, #38046, #60571, #32876, #60942, #5534 ),
 .UNSPECIFIED., .F., .F. ) 
 B_SPLINE_CURVE_WITH_KNOTS ( ( 3, 2, 2, 3 ),
 ( 0.4600000000000000200, 0.4633333333333333748, 0.4666666666666667851, 0.4700000000000001399 ),
 .UNSPECIFIED. ) 
 CURVE ( )  GEOMETRIC_REPRESENTATION_ITEM ( )  RATIONAL_B_SPLINE_CURVE ( ( 1.000000000000000000, 0.8660254037844387076, 1.000000000000000000, 0.8660254037844387076, 1.000000000000000000, 0.8660254037844320463, 1.000000000000006661 ) ) 
 REPRESENTATION_ITEM ( '' )  );
#9335=CARTESIAN_POINT ( 'NONE',  ( 21.15000000000000213, -4.330127018922190985, -2.500000000000001332 ) ) ;
#9346=CARTESIAN_POINT ( 'NONE',  ( 7.256250001229033408, -4.330127018922190985, -2.500000000000001332 ) ) ;
#9348=CARTESIAN_POINT ( 'NONE',  ( 15.87187500061451573, -4.119189519843968306, 2.378215178124996054 ) ) ;
#9354=DIRECTION ( 'NONE',  ( -1.000000000000000000, -0.000000000000000000, -0.000000000000000000 ) ) ;
#9358=CARTESIAN_POINT ( 'NONE',  ( 8.784375000614515372, -2.746126346562642428, -4.756430356249999214 ) ) ;
#9367=CARTESIAN_POINT ( 'NONE',  ( 19.78125000122902932, -4.330127018922194537, 2.499999999999995559 ) ) ;
#9374=DIRECTION ( 'NONE',  ( 0.000000000000000000, 0.000000000000000000, 1.000000000000000000 ) ) ;
#9381=CARTESIAN_POINT ( 'NONE',  ( 25.92187500061451644, -5.492252693125287522, -1.008910452111647106E-15 ) ) ;
#9383=CARTESIAN_POINT ( 'NONE',  ( 8.409375000614518925, -4.119189519843965641, -2.378215178125001383 ) ) ;
#9401=CARTESIAN_POINT ( 'NONE',  ( 21.73125000122903216, 6.123233995736764310E-16, -4.999999999999998224 ) ) ;
#9409=CARTESIAN_POINT ( 'NONE',  ( 45.00000000000000000, 0.000000000000000000, 0.000000000000000000 ) ) ;
#9417=CARTESIAN_POINT ( 'NONE',  ( 28.77187500061451431, 2.746126346562645981, -4.756430356249997438 ) ) ;
#9426=EDGE_CURVE ( 'NONE', #61742, #60154, #35485, .T. ) ;
#9430=DIRECTION ( 'NONE',  ( -1.000000000000000000, -0.000000000000000000, -0.000000000000000000 ) ) ;
#9435=CARTESIAN_POINT ( 'NONE',  ( 11.08125000122903181, 4.330127018922191873, 2.499999999999999556 ) ) ;
#9439=EDGE_LOOP ( 'NONE', ( #4636, #28828, #41026, #59962 ) ) ;
#9442=CARTESIAN_POINT ( 'NONE',  ( 10.42500000000000071, 6.123233995736764310E-16, -4.999999999999998224 ) ) ;
#9447=ORIENTED_EDGE ( 'NONE', *, *, #59745, .F. ) ;
#9454=CARTESIAN_POINT ( 'NONE',  ( 15.15937500061451537, 2.746126346562645981, -4.756430356249997438 ) ) ;
#9468=CARTESIAN_POINT ( 'NONE',  ( 25.85625000122903216, 4.330127018922192761, -2.499999999999997780 ) ) ;
#9473=CARTESIAN_POINT ( 'NONE',  ( 16.05937500061451573, -4.119189519843965641, -2.378215178125001383 ) ) ;
#9477=ADVANCED_FACE ( 'NONE', ( #54299 ), #5865, .T. ) ;
#9490=CARTESIAN_POINT ( 'NONE',  ( 29.08125000122903003, 4.330127018922191873, 2.499999999999999556 ) ) ;
#9514=CARTESIAN_POINT ( 'NONE',  ( 26.43750000000000000, -2.886751345948129988, 4.999999999999997335 ) ) ;
#9516=DIRECTION ( 'NONE',  ( -1.000000000000000000, -0.000000000000000000, -0.000000000000000000 ) ) ;
#9523=CARTESIAN_POINT ( 'NONE',  ( 9.243750001229033231, 5.773502691896255534, 3.535250795749688401E-16 ) ) ;
#9536=CARTESIAN_POINT ( 'NONE',  ( 21.04687500061451644, 4.119189519843966529, -2.378215178124998275 ) ) ;
#9540=CARTESIAN_POINT ( 'NONE',  ( 16.10625000122903216, 0.000000000000000000, 4.999999999999998224 ) ) ;
#9545=CARTESIAN_POINT ( 'NONE',  ( 13.12500000000000178, 6.123233995736764310E-16, -4.999999999999998224 ) ) ;
#9552=CARTESIAN_POINT ( 'NONE',  ( 24.00937500061451502, 0.000000000000000000, 4.756430356249998326 ) ) ;
#9555=CARTESIAN_POINT ( 'NONE',  ( 13.33125000122903359, 4.330127018922191873, 2.499999999999999556 ) ) ;
#9574=CARTESIAN_POINT ( 'NONE',  ( 10.95937500061451964, 0.000000000000000000, 4.756430356249998326 ) ) ;
#9586=ORIENTED_EDGE ( 'NONE', *, *, #68789, .F. ) ;
#9598=PRODUCT ( 'spindle', 'spindle', '', ( #20087 ) ) ;
#9601=CARTESIAN_POINT ( 'NONE',  ( 11.93437500061451573, -4.119189519843968306, 2.378215178124996054 ) ) ;
#9607=( BOUNDED_SURFACE ( )  B_SPLINE_SURFACE ( 1, 2, ( 
 ( #36345, #19330, #48531, #24884, #64413, #41885, #58860, #2731, #48162, #8270, #30800, #13072, #18966, #37067, #7903, #70325, #25246, #53703, #47795, #20062, #69605, #58494, #14168, #13424, #35611, #19701, #25992, #53333, #42254, #52609, #13806, #42618, #64777, #70687, #36702, #59224, #8632, #41173, #58131, #2366, #3472, #18608, #3096, #47070, #31161, #30441, #35974, #25625, #52970, #65142, #14533, #59591, #41526, #63682, #64045, #7537, #9004, #31536, #54076, #30070, #2015, #47429, #24526, #69960, #40248, #69416, #1097, #23605, #52054, #17687, #63847, #35058, #63129, #50967, #46150, #12525, #62769, #57585, #6988, #23964, #6632, #29519, #363, #28789, #18771, #12160, #51693, #34688, #28430, #39894, #40608, #45792, #1458, #46512, #68327, #29161, #23241, #56855, #69051, #57219, #18413, #35415, #57940, #5897, #40979, #68690, #22870, #18050, #17335, #24328, #6261, #56504, #63494, #12882, #7347, #51330, #29877, #45428, #67962, #41337, #52413, #1821, #62407, #46877, #11806, #13238, #34323, #732, #59763, #37242, #65680, #35776, #64212, #25053, #58299, #3637, #48700, #42787, #19873, #26161, #7708, #53502, #30606, #47968, #19503, #71223, #2894, #25425, #31337, #70125, #43160, #70496, #20235, #20601, #42426, #2533, #48336, #53134, #30242, #53878, #3270, #64947, #25798, #65308, #14339, #52775, #70861, #2177, #13601, #36873, #24690, #47596, #59391, #14698, #42060, #8801, #36509, #9170, #64583, #30967, #13971, #31705, #47234, #54240, #69767, #19135, #41689, #59029, #36147, #8431, #58666, #8074, #26905, #38336, #27629, #60491, #27266, #10268, #9897, #33513, #32801, #4376, #54602, #44633, #21704, #44261, #5093, #21339, #60865, #71965, #44982, #22074, #55337, #15426, #60127, #66794, #61237, #26530, #56062, #61592, #32070, #50162, #49431, #4732, #5455, #66418, #49799, #72692, #32433, #67162, #20973, #27995, #9536, #43894, #72324, #54970, #16523, #4007, #49070, #50524, #39075, #15796, #16165, #10993, #55699, #15068, #10631, #73052, #22434, #38717, #33161, #37605, #71598, #43526, #66048, #37970, #51610, #23880, #34602, #6541, #61958, #67877, #12795, #56771, #46067, #1010, #29434, #23517, #68965, #45343, #34237, #63040, #62325, #11362, #68602, #1730, #57131, #29075, #28345, #17606, #18322, #17963, #46427, #40524, #40166, #12081, #16884, #33880, #51244, #52328, #67519, #51971, #22790, #12439, #6175, #11721, #57501, #28705, #40895, #62685, #34972, #17249, #24243, #39809, #56425, #6903, #1370, #63409, #39438, #35331, #647, #5814, #57854, #23155, #50882, #7263, #282, #45709, #68243, #29792, #41251, #36427, #9086, #69684, #47883, #42702, #58941, #13512, #59304, #64126, #31623, #42339, #14250, #8349, #64862, #31247, #53419, #63762, #36789, #13151, #24604, #30878, #35693, #36059, #2810, #3184, #7987, #25338, #47512, #53788, #58579, #41974, #30523, #19788, #54157, #8715, #25711, #70772, #48248, #53050, #20148, #19414, #65224, #3553, #2444, #70041, #14614, #19049, #70412, #64495, #41607, #37153, #59678, #58213, #13887, #46792, #24967, #69328, #18687, #7618, #30154, #52688, #2094, #47152, #39990, #60405, #21254, #4290, #71139, #9454, #10184, #15345, #55256, #16081, #37885, #49350, #65965, #26444, #27181, #32346, #38630, #5012, #27546, #48614, #66708, #43807, #65595, #66332, #60043, #68064, #48984, #26075, #33078, #61154, #4652, #71513, #9814, #20512, #43069, #11901, #10549, #60777, #14984, #50078, #31984, #55616, #54884, #26816, #465, #22973, #56954, #37522, #54518, #71881, #3921, #17432, #62503, #45535, #32719, #34426, #20889, #15710, #43443, #38248, #49715, #72243, #21620, #44178, #1921, #40709, #13704, #69152, #63948, #69864, #18511, #18142, #29614, #46246, #6725, #7444, #12621, #69510, #58395, #7808, #28890, #46975, #24063, #45888, #1553, #40341, #47331, #29259, #6358, #13333, #18870, #35515, #51789, #63227, #831, #51429, #64314, #41432, #41076, #23339, #30345, #12257, #35871, #35156, #68786, #52873, #2271, #36247, #68420, #34788, #57680, #17782, #19230, #41784, #24787, #63590, #62862, #57321, #46609, #1190, #12978, #7085, #23698, #58034, #29970, #24426, #52150, #52511, #48437, #43262, #49173, #70962, #25524, #71329, #2996, #43627, #54344, #26263, #20335, #3738, #65783, #65411, #53231, #48800, #25150, #36607, #42888, #2628, #48067, #14801, #15165, #19968, #37344, #59494, #37702, #70593, #53978, #42521, #31806, #21076, #20704, #60223, #9637, #32171, #65047, #54704, #31438, #4109, #66149, #14437, #8907, #26637, #31064, #59867, #3376, #53602, #9271, #71704, #47690, #25897, #15527, #36971, #58761, #8171, #30699, #70226, #19600, #42156, #64683, #14068, #59128, #8535, #16263, #10002, #21437, #22175, #27365, #67263, #28094, #45080, #55439, #33263, #49896, #11091, #377, #33619, #56163, #62064, #5557, #21804, #50622, #10731, #27, #45443, #72421, #61333, #22533 ),
 ( #50980, #44368, #55801, #38818, #32537, #43994, #44728, #66895, #16621, #67616, #5191, #27729, #4831, #38443, #39176, #50267, #16982, #39539, #11458, #60593, #33979, #72792, #4474, #61692, #72058, #5911, #60969, #38069, #56518, #28445, #22885, #10369, #67976, #55074, #27004, #49534, #66516, #15896, #32899, #69430, #23255, #46892, #46164, #6647, #41352, #18787, #47250, #17349, #45805, #29174, #39908, #58313, #30258, #24344, #1473, #7724, #62421, #35073, #12175, #29533, #1111, #52791, #57599, #7002, #12897, #51708, #24706, #52068, #1836, #2192, #23979, #57232, #29891, #34703, #11820, #35430, #57954, #46527, #7362, #63862, #69069, #34337, #52430, #56871, #68341, #18428, #6275, #23618, #40994, #13252, #68704, #63510, #18064, #40625, #35790, #17701, #28803, #51344, #63144, #746, #12539, #40262, #62783, #13617, #32086, #9187, #42077, #70514, #31722, #37259, #69783, #42804, #60143, #3654, #14356, #19890, #26548, #2912, #42443, #64965, #36891, #53896, #26177, #59410, #8818, #64228, #70141, #15084, #59045, #48353, #3287, #54258, #25815, #71240, #47611, #36525, #65326, #64599, #36162, #70878, #4023, #31355, #20252, #30620, #14717, #20620, #59781, #48718, #43178, #65697, #37621, #19150, #58680, #53518, #54617, #41704, #9552, #25068, #8090, #8449, #13986, #53150, #30985, #2549, #19519, #25443, #47986, #5830, #49447, #43543, #61610, #16540, #11011, #71617, #56082, #21354, #60508, #44649, #71981, #9914, #28013, #56440, #15812, #49089, #22091, #66064, #38733, #11377, #43910, #50180, #44999, #61253, #67536, #44279, #38354, #15442, #5474, #55715, #5110, #39093, #55354, #21720, #32816, #20990, #50541, #72339, #66434, #37986, #27644, #67179, #32452, #16899, #22450, #54987, #33532, #60881, #66810, #39454, #27282, #10647, #73069, #10286, #16182, #61975, #49815, #33177, #33896, #4748, #4393, #26922, #72708, #22807, #12097, #12459, #23171, #29811, #45359, #67893, #63782, #40914, #663, #29092, #63427, #68983, #28362, #1388, #18706, #35348, #46084, #51628, #58233, #34618, #1028, #23534, #68620, #34990, #57872, #17982, #40541, #17265, #28720, #46811, #17623, #6920, #57519, #12814, #29450, #52346, #6192, #68260, #23897, #45725, #39827, #51987, #35711, #63057, #46445, #62342, #18340, #1749, #7282, #24262, #69348, #41270, #13171, #50898, #11737, #57148, #298, #34254, #56787, #51261, #40182, #62703, #6560, #70793, #24987, #9105, #2830, #30897, #36079, #37540, #8007, #2113, #20168, #48269, #42722, #30176, #14632, #53069, #19069, #3203, #30542, #41625, #59698, #15003, #47532, #7638, #53809, #24624, #70432, #43087, #2464, #8733, #3572, #19807, #26095, #25358, #70060, #47171, #37172, #14270, #36808, #65243, #13908, #53439, #64515, #52707, #31643, #47903, #19434, #69703, #59323, #25731, #64145, #48633, #54175, #13532, #71158, #65614, #58600, #20530, #41995, #36447, #58961, #8369, #42360, #64882, #31267, #55273, #10200, #15364, #16820, #60424, #54538, #72626, #27564, #22010, #9473, #67096, #32364, #71533, #55633, #9835, #20908, #39012, #67457, #26835, #60062, #33094, #3940, #49733, #22369, #54902, #61171, #55996, #72260, #5389, #4668, #49369, #26463, #16454, #66726, #16097, #50095, #66350, #32736, #43826, #32003, #61527, #27198, #4310, #49002, #38647, #5026, #43460, #27927, #33452, #65984, #44566, #71899, #21637, #50460, #38267, #44195, #10925, #21272, #72987, #37906, #44921, #15728, #60795, #10566, #34173, #40825, #33818, #56362, #1664, #51902, #11658, #40103, #1300, #6835, #39374, #12369, #29723, #46361, #57066, #62616, #69260, #45645, #12013, #34536, #6473, #23454, #68895, #29008, #51545, #5752, #39745, #57786, #28641, #17897, #45999, #23810, #68536, #63342, #17185, #6110, #34904, #56709, #28286, #40457, #46725, #946, #62973, #220, #57431, #12728, #29370, #18252, #35264, #7195, #52261, #61893, #50817, #23088, #24173, #11298, #68179, #22725, #45278, #67811, #62261, #51179, #583, #17541, #13087, #18980, #37081, #7917, #70338, #25262, #53717, #47809, #20075, #69618, #58507, #14181, #13439, #35625, #19715, #26005, #58872, #53345, #52623, #41899, #42631, #42267, #48176, #64790, #64426, #36358, #41187, #58145, #2379, #3487, #18622, #3109, #47084, #36715, #30454, #35989, #8645, #52983, #65155, #13818, #8282, #41541, #48544, #64059, #7551, #31174, #59237, #25638, #63696, #70700, #24897, #30085, #14545, #47442, #2029, #59605, #24540, #69974, #19344, #9019, #30812, #2743, #54089, #31549, #72170, #67007, #60701, #16368, #66258, #60335, #37455, #27475, #4580, #27110, #61079, #4218, #43734, #54812, #27845, #4941, #21182, #71442, #42996, #49643, #44104, #9383, #38923, #44476, #14913, #33006, #9744, #15636, #61442, #49279, #32644, #10477, #65896, #55545, #3850, #10835, #65527, #26746, #55185, #15276, #72532, #59974, #31915, #33371, #50007, #43372, #71812, #21920, #38556, #71071 ) ),
 .UNSPECIFIED., .F., .F., .F. ) 
 B_SPLINE_SURFACE_WITH_KNOTS ( ( 2, 2 ),
 ( 3, 2, 2, 2, 2, 2, 2, 2, 2, 2, 2, 2, 2, 2, 2, 2, 2, 2, 2, 2, 2, 2, 2, 2, 2, 2, 2, 2, 2, 2, 2, 2, 2, 2, 2, 2, 2, 2, 2, 2, 2, 2, 2, 2, 2, 2, 2, 2, 2, 2, 2, 2, 2, 2, 2, 2, 2, 2, 2, 2, 2, 2, 2, 2, 2, 2, 2, 2, 2, 2, 2, 2, 2, 2, 2, 2, 2, 2, 2, 2, 2, 2, 2, 2, 2, 2, 2, 2, 2, 2, 2, 2, 2, 2, 2, 2, 2, 2, 2, 2, 2, 2, 2, 2, 2, 2, 2, 2, 2, 2, 2, 2, 2, 2, 2, 2, 2, 2, 2, 2, 2, 2, 2, 2, 2, 2, 2, 2, 2, 2, 2, 2, 2, 2, 2, 2, 2, 2, 2, 2, 2, 2, 2, 2, 2, 2, 2, 2, 2, 2, 2, 2, 2, 2, 2, 2, 2, 2, 2, 2, 2, 2, 2, 2, 2, 2, 2, 2, 2, 2, 2, 2, 2, 2, 2, 2, 2, 2, 2, 2, 2, 2, 2, 2, 2, 2, 2, 2, 2, 2, 2, 2, 2, 2, 2, 2, 2, 2, 2, 2, 2, 2, 2, 2, 2, 2, 2, 2, 2, 2, 2, 2, 2, 2, 2, 2, 2, 2, 2, 2, 2, 2, 2, 2, 2, 2, 2, 2, 2, 2, 2, 2, 2, 2, 2, 2, 2, 2, 2, 2, 2, 2, 2, 2, 2, 2, 2, 2, 2, 2, 2, 2, 2, 2, 2, 2, 2, 2, 2, 2, 2, 2, 2, 2, 2, 2, 2, 2, 2, 2, 2, 2, 2, 2, 2, 2, 2, 2, 2, 2, 2, 2, 2, 2, 2, 2, 2, 2, 2, 2, 2, 2, 2, 2, 2, 2, 2, 2, 2, 2, 3 ),
 ( 0.000000000000000000, 1.000000000000000000 ),
 ( 0.000000000000000000, 0.003333333333333333547, 0.006666666666666667095, 0.01000000000000000021, 0.01333333333333333419, 0.01666666666666666644, 0.02000000000000000042, 0.02333333333333333440, 0.02666666666666666838, 0.02999999999999999889, 0.03333333333333333287, 0.03666666666666666685, 0.04000000000000000083, 0.04333333333333333481, 0.04666666666666666879, 0.05000000000000000278, 0.05333333333333333676, 0.05666666666666666380, 0.05999999999999999778, 0.06333333333333333870, 0.06666666666666666574, 0.07000000000000000666, 0.07333333333333333370, 0.07666666666666666075, 0.08000000000000000167, 0.08333333333333332871, 0.08666666666666666963, 0.08999999999999999667, 0.09333333333333333759, 0.09666666666666666463, 0.1000000000000000056, 0.1033333333333333326, 0.1066666666666666735, 0.1100000000000000006, 0.1133333333333333276, 0.1166666666666666685, 0.1199999999999999956, 0.1233333333333333365, 0.1266666666666666774, 0.1300000000000000044, 0.1333333333333333315, 0.1366666666666666585, 0.1400000000000000133, 0.1433333333333333404, 0.1466666666666666674, 0.1499999999999999944, 0.1533333333333333215, 0.1566666666666666763, 0.1600000000000000033, 0.1633333333333333304, 0.1666666666666666574, 0.1700000000000000122, 0.1733333333333333393, 0.1766666666666666663, 0.1799999999999999933, 0.1833333333333333204, 0.1866666666666666752, 0.1900000000000000022, 0.1933333333333333293, 0.1966666666666666563, 0.2000000000000000111, 0.2033333333333333381, 0.2066666666666666652, 0.2099999999999999922, 0.2133333333333333470, 0.2166666666666666741, 0.2200000000000000011, 0.2233333333333333282, 0.2266666666666666552, 0.2300000000000000100, 0.2333333333333333370, 0.2366666666666666641, 0.2399999999999999911, 0.2433333333333333459, 0.2466666666666666730, 0.2500000000000000000, 0.2533333333333333548, 0.2566666666666666541, 0.2600000000000000089, 0.2633333333333333082, 0.2666666666666666630, 0.2700000000000000178, 0.2733333333333333171, 0.2766666666666666718, 0.2800000000000000266, 0.2833333333333333259, 0.2866666666666666807, 0.2899999999999999800, 0.2933333333333333348, 0.2966666666666666896, 0.2999999999999999889, 0.3033333333333333437, 0.3066666666666666430, 0.3099999999999999978, 0.3133333333333333526, 0.3166666666666666519, 0.3200000000000000067, 0.3233333333333333059, 0.3266666666666666607, 0.3300000000000000155, 0.3333333333333333148, 0.3366666666666666696, 0.3400000000000000244, 0.3433333333333333237, 0.3466666666666666785, 0.3499999999999999778, 0.3533333333333333326, 0.3566666666666666874, 0.3599999999999999867, 0.3633333333333333415, 0.3666666666666666408, 0.3699999999999999956, 0.3733333333333333504, 0.3766666666666666496, 0.3800000000000000044, 0.3833333333333333592, 0.3866666666666666585, 0.3900000000000000133, 0.3933333333333333126, 0.3966666666666666674, 0.4000000000000000222, 0.4033333333333333215, 0.4066666666666666763, 0.4099999999999999756, 0.4133333333333333304, 0.4166666666666666852, 0.4199999999999999845, 0.4233333333333333393, 0.4266666666666666941, 0.4299999999999999933, 0.4333333333333333481, 0.4366666666666666474, 0.4400000000000000022, 0.4433333333333333570, 0.4466666666666666563, 0.4500000000000000111, 0.4533333333333333104, 0.4566666666666666652, 0.4600000000000000200, 0.4633333333333333193, 0.4666666666666666741, 0.4699999999999999734, 0.4733333333333333282, 0.4766666666666666829, 0.4799999999999999822, 0.4833333333333333370, 0.4866666666666666918, 0.4899999999999999911, 0.4933333333333333459, 0.4966666666666666452, 0.5000000000000000000, 0.5033333333333332993, 0.5066666666666667096, 0.5100000000000000089, 0.5133333333333333082, 0.5166666666666667185, 0.5200000000000000178, 0.5233333333333333171, 0.5266666666666666163, 0.5300000000000000266, 0.5333333333333333259, 0.5366666666666666252, 0.5400000000000000355, 0.5433333333333333348, 0.5466666666666666341, 0.5500000000000000444, 0.5533333333333333437, 0.5566666666666666430, 0.5600000000000000533, 0.5633333333333333526, 0.5666666666666666519, 0.5699999999999999512, 0.5733333333333333615, 0.5766666666666666607, 0.5799999999999999600, 0.5833333333333333703, 0.5866666666666666696, 0.5899999999999999689, 0.5933333333333333792, 0.5966666666666666785, 0.5999999999999999778, 0.6033333333333333881, 0.6066666666666666874, 0.6099999999999999867, 0.6133333333333332860, 0.6166666666666666963, 0.6199999999999999956, 0.6233333333333332948, 0.6266666666666667052, 0.6300000000000000044, 0.6333333333333333037, 0.6366666666666667140, 0.6400000000000000133, 0.6433333333333333126, 0.6466666666666666119, 0.6500000000000000222, 0.6533333333333333215, 0.6566666666666666208, 0.6600000000000000311, 0.6633333333333333304, 0.6666666666666666297, 0.6700000000000000400, 0.6733333333333333393, 0.6766666666666666385, 0.6800000000000000488, 0.6833333333333333481, 0.6866666666666666474, 0.6899999999999999467, 0.6933333333333333570, 0.6966666666666666563, 0.6999999999999999556, 0.7033333333333333659, 0.7066666666666666652, 0.7099999999999999645, 0.7133333333333333748, 0.7166666666666666741, 0.7199999999999999734, 0.7233333333333333837, 0.7266666666666666829, 0.7299999999999999822, 0.7333333333333332815, 0.7366666666666666918, 0.7399999999999999911, 0.7433333333333332904, 0.7466666666666667007, 0.7500000000000000000, 0.7533333333333332993, 0.7566666666666667096, 0.7600000000000000089, 0.7633333333333333082, 0.7666666666666667185, 0.7700000000000000178, 0.7733333333333333171, 0.7766666666666666163, 0.7800000000000000266, 0.7833333333333333259, 0.7866666666666666252, 0.7900000000000000355, 0.7933333333333333348, 0.7966666666666666341, 0.8000000000000000444, 0.8033333333333333437, 0.8066666666666666430, 0.8100000000000000533, 0.8133333333333333526, 0.8166666666666666519, 0.8199999999999999512, 0.8233333333333333615, 0.8266666666666666607, 0.8299999999999999600, 0.8333333333333333703, 0.8366666666666666696, 0.8399999999999999689, 0.8433333333333333792, 0.8466666666666666785, 0.8499999999999999778, 0.8533333333333333881, 0.8566666666666666874, 0.8599999999999999867, 0.8633333333333332860, 0.8666666666666666963, 0.8699999999999999956, 0.8733333333333332948, 0.8766666666666667052, 0.8800000000000000044, 0.8833333333333333037, 0.8866666666666667140, 0.8900000000000000133, 0.8933333333333333126, 0.8966666666666666119, 0.9000000000000000222, 0.9033333333333333215, 0.9066666666666666208, 0.9100000000000000311, 0.9133333333333333304, 0.9166666666666666297, 0.9200000000000000400, 0.9233333333333333393, 0.9266666666666666385, 0.9300000000000000488, 0.9333333333333333481, 0.9366666666666666474, 0.9399999999999999467, 0.9433333333333333570, 0.9466666666666666563, 0.9499999999999999556, 0.9533333333333333659, 0.9566666666666666652, 0.9599999999999999645, 0.9633333333333333748, 0.9666666666666666741, 0.9699999999999999734, 0.9733333333333333837, 0.9766666666666666829, 0.9799999999999999822, 0.9833333333333332815, 0.9866666666666666918, 0.9899999999999999911, 0.9933333333333332904, 0.9966666666666667007, 1.000000000000000000 ),
 .UNSPECIFIED. ) 
 GEOMETRIC_REPRESENTATION_ITEM ( )  RATIONAL_B_SPLINE_SURFACE ( (
 ( 1.000000000000000000, 0.8660254037844387076, 1.000000000000000000, 0.8660254037844387076, 1.000000000000000000, 0.8660254037844387076, 1.000000000000000000, 0.8660254037844387076, 1.000000000000000000, 0.8660254037844387076, 1.000000000000000000, 0.8660254037844387076, 1.000000000000000000, 0.8660254037844387076, 1.000000000000000000, 0.8660254037844387076, 1.000000000000000000, 0.8660254037844387076, 1.000000000000000000, 0.8660254037844387076, 1.000000000000000000, 0.8660254037844387076, 1.000000000000000000, 0.8660254037844387076, 1.000000000000000000, 0.8660254037844387076, 1.000000000000000000, 0.8660254037844387076, 1.000000000000000000, 0.8660254037844387076, 1.000000000000000000, 0.8660254037844387076, 1.000000000000000000, 0.8660254037844387076, 1.000000000000000000, 0.8660254037844387076, 1.000000000000000000, 0.8660254037844387076, 1.000000000000000000, 0.8660254037844387076, 1.000000000000000000, 0.8660254037844387076, 1.000000000000000000, 0.8660254037844387076, 1.000000000000000000, 0.8660254037844387076, 1.000000000000000000, 0.8660254037844387076, 1.000000000000000000, 0.8660254037844387076, 1.000000000000000000, 0.8660254037844387076, 1.000000000000000000, 0.8660254037844387076, 1.000000000000000000, 0.8660254037844387076, 1.000000000000000000, 0.8660254037844387076, 1.000000000000000000, 0.8660254037844387076, 1.000000000000000000, 0.8660254037844387076, 1.000000000000000000, 0.8660254037844387076, 1.000000000000000000, 0.8660254037844387076, 1.000000000000000000, 0.8660254037844387076, 1.000000000000000000, 0.8660254037844387076, 1.000000000000000000, 0.8660254037844387076, 1.000000000000000000, 0.8660254037844387076, 1.000000000000000000, 0.8660254037844387076, 1.000000000000000000, 0.8660254037844387076, 1.000000000000000000, 0.8660254037844387076, 1.000000000000000000, 0.8660254037844387076, 1.000000000000000000, 0.8660254037844387076, 1.000000000000000000, 0.8660254037844387076, 1.000000000000000000, 0.8660254037844387076, 1.000000000000000000, 0.8660254037844387076, 1.000000000000000000, 0.8660254037844387076, 1.000000000000000000, 0.8660254037844387076, 1.000000000000000000, 0.8660254037844387076, 1.000000000000000000, 0.8660254037844387076, 1.000000000000000000, 0.8660254037844387076, 1.000000000000000000, 0.8660254037844387076, 1.000000000000000000, 0.8660254037844387076, 1.000000000000000000, 0.8660254037844387076, 1.000000000000000000, 0.8660254037844387076, 1.000000000000000000, 0.8660254037844387076, 1.000000000000000000, 0.8660254037844387076, 1.000000000000000000, 0.8660254037844387076, 1.000000000000000000, 0.8660254037844387076, 1.000000000000000000, 0.8660254037844387076, 1.000000000000000000, 0.8660254037844387076, 1.000000000000000000, 0.8660254037844387076, 1.000000000000000000, 0.8660254037844387076, 1.000000000000000000, 0.8660254037844387076, 1.000000000000000000, 0.8660254037844387076, 1.000000000000000000, 0.8660254037844387076, 1.000000000000000000, 0.8660254037844387076, 1.000000000000000000, 0.8660254037844387076, 1.000000000000000000, 0.8660254037844387076, 1.000000000000000000, 0.8660254037844387076, 1.000000000000000000, 0.8660254037844387076, 1.000000000000000000, 0.8660254037844387076, 1.000000000000000000, 0.8660254037844387076, 1.000000000000000000, 0.8660254037844387076, 1.000000000000000000, 0.8660254037844387076, 1.000000000000000000, 0.8660254037844387076, 1.000000000000000000, 0.8660254037844387076, 1.000000000000000000, 0.8660254037844387076, 1.000000000000000000, 0.8660254037844387076, 1.000000000000000000, 0.8660254037844387076, 1.000000000000000000, 0.8660254037844387076, 1.000000000000000000, 0.8660254037844387076, 1.000000000000000000, 0.8660254037844387076, 1.000000000000000000, 0.8660254037844387076, 1.000000000000000000, 0.8660254037844387076, 1.000000000000000000, 0.8660254037844387076, 1.000000000000000000, 0.8660254037844387076, 1.000000000000000000, 0.8660254037844387076, 1.000000000000000000, 0.8660254037844387076, 1.000000000000000000, 0.8660254037844387076, 1.000000000000000000, 0.8660254037844387076, 1.000000000000000000, 0.8660254037844387076, 1.000000000000000000, 0.8660254037844387076, 1.000000000000000000, 0.8660254037844387076, 1.000000000000000000, 0.8660254037844387076, 1.000000000000000000, 0.8660254037844387076, 1.000000000000000000, 0.8660254037844387076, 1.000000000000000000, 0.8660254037844387076, 1.000000000000000000, 0.8660254037844387076, 1.000000000000000000, 0.8660254037844387076, 1.000000000000000000, 0.8660254037844387076, 1.000000000000000000, 0.8660254037844387076, 1.000000000000000000, 0.8660254037844387076, 1.000000000000000000, 0.8660254037844387076, 1.000000000000000000, 0.8660254037844387076, 1.000000000000000000, 0.8660254037844387076, 1.000000000000000000, 0.8660254037844387076, 1.000000000000000000, 0.8660254037844387076, 1.000000000000000000, 0.8660254037844387076, 1.000000000000000000, 0.8660254037844387076, 1.000000000000000000, 0.8660254037844387076, 1.000000000000000000, 0.8660254037844387076, 1.000000000000000000, 0.8660254037844387076, 1.000000000000000000, 0.8660254037844387076, 1.000000000000000000, 0.8660254037844387076, 1.000000000000000000, 0.8660254037844387076, 1.000000000000000000, 0.8660254037844387076, 1.000000000000000000, 0.8660254037844387076, 1.000000000000000000, 0.8660254037844387076, 1.000000000000000000, 0.8660254037844387076, 1.000000000000000000, 0.8660254037844387076, 1.000000000000000000, 0.8660254037844387076, 1.000000000000000000, 0.8660254037844387076, 1.000000000000000000, 0.8660254037844387076, 1.000000000000000000, 0.8660254037844387076, 1.000000000000000000, 0.8660254037844387076, 1.000000000000000000, 0.8660254037844387076, 1.000000000000000000, 0.8660254037844387076, 1.000000000000000000, 0.8660254037844387076, 1.000000000000000000, 0.8660254037844387076, 1.000000000000000000, 0.8660254037844387076, 1.000000000000000000, 0.8660254037844387076, 1.000000000000000000, 0.8660254037844387076, 1.000000000000000000, 0.8660254037844387076, 1.000000000000000000, 0.8660254037844387076, 1.000000000000000000, 0.8660254037844387076, 1.000000000000000000, 0.8660254037844387076, 1.000000000000000000, 0.8660254037844387076, 1.000000000000000000, 0.8660254037844387076, 1.000000000000000000, 0.8660254037844387076, 1.000000000000000000, 0.8660254037844387076, 1.000000000000000000, 0.8660254037844387076, 1.000000000000000000, 0.8660254037844387076, 1.000000000000000000, 0.8660254037844387076, 1.000000000000000000, 0.8660254037844387076, 1.000000000000000000, 0.8660254037844387076, 1.000000000000000000, 0.8660254037844387076, 1.000000000000000000, 0.8660254037844387076, 1.000000000000000000, 0.8660254037844387076, 1.000000000000000000, 0.8660254037844387076, 1.000000000000000000, 0.8660254037844387076, 1.000000000000000000, 0.8660254037844387076, 1.000000000000000000, 0.8660254037844387076, 1.000000000000000000, 0.8660254037844387076, 1.000000000000000000, 0.8660254037844387076, 1.000000000000000000, 0.8660254037844387076, 1.000000000000000000, 0.8660254037844387076, 1.000000000000000000, 0.8660254037844387076, 1.000000000000000000, 0.8660254037844387076, 1.000000000000000000, 0.8660254037844387076, 1.000000000000000000, 0.8660254037844387076, 1.000000000000000000, 0.8660254037844387076, 1.000000000000000000, 0.8660254037844387076, 1.000000000000000000, 0.8660254037844387076, 1.000000000000000000, 0.8660254037844387076, 1.000000000000000000, 0.8660254037844387076, 1.000000000000000000, 0.8660254037844387076, 1.000000000000000000, 0.8660254037844387076, 1.000000000000000000, 0.8660254037844387076, 1.000000000000000000, 0.8660254037844387076, 1.000000000000000000, 0.8660254037844387076, 1.000000000000000000, 0.8660254037844387076, 1.000000000000000000, 0.8660254037844387076, 1.000000000000000000, 0.8660254037844387076, 1.000000000000000000, 0.8660254037844387076, 1.000000000000000000, 0.8660254037844387076, 1.000000000000000000, 0.8660254037844387076, 1.000000000000000000, 0.8660254037844387076, 1.000000000000000000, 0.8660254037844387076, 1.000000000000000000, 0.8660254037844387076, 1.000000000000000000, 0.8660254037844387076, 1.000000000000000000, 0.8660254037844387076, 1.000000000000000000, 0.8660254037844387076, 1.000000000000000000, 0.8660254037844387076, 1.000000000000000000, 0.8660254037844387076, 1.000000000000000000, 0.8660254037844387076, 1.000000000000000000, 0.8660254037844387076, 1.000000000000000000, 0.8660254037844387076, 1.000000000000000000, 0.8660254037844387076, 1.000000000000000000, 0.8660254037844387076, 1.000000000000000000, 0.8660254037844387076, 1.000000000000000000, 0.8660254037844387076, 1.000000000000000000, 0.8660254037844387076, 1.000000000000000000, 0.8660254037844387076, 1.000000000000000000, 0.8660254037844387076, 1.000000000000000000, 0.8660254037844387076, 1.000000000000000000, 0.8660254037844387076, 1.000000000000000000, 0.8660254037844387076, 1.000000000000000000, 0.8660254037844387076, 1.000000000000000000, 0.8660254037844387076, 1.000000000000000000, 0.8660254037844387076, 1.000000000000000000, 0.8660254037844387076, 1.000000000000000000, 0.8660254037844387076, 1.000000000000000000, 0.8660254037844387076, 1.000000000000000000, 0.8660254037844387076, 1.000000000000000000, 0.8660254037844387076, 1.000000000000000000, 0.8660254037844387076, 1.000000000000000000, 0.8660254037844387076, 1.000000000000000000, 0.8660254037844387076, 1.000000000000000000, 0.8660254037844387076, 1.000000000000000000, 0.8660254037844387076, 1.000000000000000000, 0.8660254037844387076, 1.000000000000000000, 0.8660254037844387076, 1.000000000000000000, 0.8660254037844387076, 1.000000000000000000, 0.8660254037844387076, 1.000000000000000000, 0.8660254037844387076, 1.000000000000000000, 0.8660254037844387076, 1.000000000000000000, 0.8660254037844387076, 1.000000000000000000, 0.8660254037844387076, 1.000000000000000000, 0.8660254037844387076, 1.000000000000000000, 0.8660254037844387076, 1.000000000000000000, 0.8660254037844387076, 1.000000000000000000, 0.8660254037844387076, 1.000000000000000000, 0.8660254037844387076, 1.000000000000000000, 0.8660254037844387076, 1.000000000000000000, 0.8660254037844387076, 1.000000000000000000, 0.8660254037844387076, 1.000000000000000000, 0.8660254037844387076, 1.000000000000000000, 0.8660254037844387076, 1.000000000000000000, 0.8660254037844387076, 1.000000000000000000, 0.8660254037844387076, 1.000000000000000000, 0.8660254037844387076, 1.000000000000000000, 0.8660254037844387076, 1.000000000000000000, 0.8660254037844387076, 1.000000000000000000, 0.8660254037844387076, 1.000000000000000000, 0.8660254037844387076, 1.000000000000000000, 0.8660254037844387076, 1.000000000000000000, 0.8660254037844387076, 1.000000000000000000, 0.8660254037844387076, 1.000000000000000000, 0.8660254037844387076, 1.000000000000000000, 0.8660254037844387076, 1.000000000000000000, 0.8660254037844387076, 1.000000000000000000, 0.8660254037844387076, 1.000000000000000000, 0.8660254037844387076, 1.000000000000000000, 0.8660254037844387076, 1.000000000000000000, 0.8660254037844387076, 1.000000000000000000, 0.8660254037844387076, 1.000000000000000000, 0.8660254037844387076, 1.000000000000000000, 0.8660254037844387076, 1.000000000000000000, 0.8660254037844387076, 1.000000000000000000, 0.8660254037844387076, 1.000000000000000000, 0.8660254037844387076, 1.000000000000000000, 0.8660254037844387076, 1.000000000000000000, 0.8660254037844387076, 1.000000000000000000, 0.8660254037844387076, 1.000000000000000000, 0.8660254037844387076, 1.000000000000000000, 0.8660254037844387076, 1.000000000000000000, 0.8660254037844387076, 1.000000000000000000, 0.8660254037844387076, 1.000000000000000000, 0.8660254037844387076, 1.000000000000000000, 0.8660254037844387076, 1.000000000000000000, 0.8660254037844387076, 1.000000000000000000, 0.8660254037844387076, 1.000000000000000000, 0.8660254037844387076, 1.000000000000000000, 0.8660254037844387076, 1.000000000000000000, 0.8660254037844387076, 1.000000000000000000, 0.8660254037844387076, 1.000000000000000000, 0.8660254037844387076, 1.000000000000000000, 0.8660254037844387076, 1.000000000000000000, 0.8660254037844387076, 1.000000000000000000, 0.8660254037844387076, 1.000000000000000000, 0.8660254037844387076, 1.000000000000000000, 0.8660254037844387076, 1.000000000000000000, 0.8660254037844387076, 1.000000000000000000, 0.8660254037844387076, 1.000000000000000000, 0.8660254037844387076, 1.000000000000000000, 0.8660254037844387076, 1.000000000000000000, 0.8660254037844387076, 1.000000000000000000, 0.8660254037844387076, 1.000000000000000000, 0.8660254037844387076, 1.000000000000000000, 0.8660254037844387076, 1.000000000000000000, 0.8660254037844387076, 1.000000000000000000, 0.8660254037844387076, 1.000000000000000000, 0.8660254037844387076, 1.000000000000000000, 0.8660254037844387076, 1.000000000000000000, 0.8660254037844387076, 1.000000000000000000, 0.8660254037844387076, 1.000000000000000000, 0.8660254037844387076, 1.000000000000000000, 0.8660254037844387076, 1.000000000000000000, 0.8660254037844387076, 1.000000000000000000, 0.8660254037844387076, 1.000000000000000000, 0.8660254037844387076, 1.000000000000000000, 0.8660254037844387076, 1.000000000000000000, 0.8660254037844387076, 1.000000000000000000, 0.8660254037844387076, 1.000000000000000000, 0.8660254037844387076, 1.000000000000000000, 0.8660254037844387076, 1.000000000000000000, 0.8660254037844387076, 1.000000000000000000, 0.8660254037844387076, 1.000000000000000000, 0.8660254037844387076, 1.000000000000000000, 0.8660254037844387076, 1.000000000000000000),
 ( 1.000000000000000000, 0.8660254037844387076, 1.000000000000000000, 0.8660254037844387076, 1.000000000000000000, 0.8660254037844387076, 1.000000000000000000, 0.8660254037844387076, 1.000000000000000000, 0.8660254037844387076, 1.000000000000000000, 0.8660254037844387076, 1.000000000000000000, 0.8660254037844387076, 1.000000000000000000, 0.8660254037844387076, 1.000000000000000000, 0.8660254037844387076, 1.000000000000000000, 0.8660254037844387076, 1.000000000000000000, 0.8660254037844387076, 1.000000000000000000, 0.8660254037844387076, 1.000000000000000000, 0.8660254037844387076, 1.000000000000000000, 0.8660254037844387076, 1.000000000000000000, 0.8660254037844387076, 1.000000000000000000, 0.8660254037844387076, 1.000000000000000000, 0.8660254037844387076, 1.000000000000000000, 0.8660254037844387076, 1.000000000000000000, 0.8660254037844387076, 1.000000000000000000, 0.8660254037844387076, 1.000000000000000000, 0.8660254037844387076, 1.000000000000000000, 0.8660254037844387076, 1.000000000000000000, 0.8660254037844387076, 1.000000000000000000, 0.8660254037844387076, 1.000000000000000000, 0.8660254037844387076, 1.000000000000000000, 0.8660254037844387076, 1.000000000000000000, 0.8660254037844387076, 1.000000000000000000, 0.8660254037844387076, 1.000000000000000000, 0.8660254037844387076, 1.000000000000000000, 0.8660254037844387076, 1.000000000000000000, 0.8660254037844387076, 1.000000000000000000, 0.8660254037844387076, 1.000000000000000000, 0.8660254037844387076, 1.000000000000000000, 0.8660254037844387076, 1.000000000000000000, 0.8660254037844387076, 1.000000000000000000, 0.8660254037844387076, 1.000000000000000000, 0.8660254037844387076, 1.000000000000000000, 0.8660254037844387076, 1.000000000000000000, 0.8660254037844387076, 1.000000000000000000, 0.8660254037844387076, 1.000000000000000000, 0.8660254037844387076, 1.000000000000000000, 0.8660254037844387076, 1.000000000000000000, 0.8660254037844387076, 1.000000000000000000, 0.8660254037844387076, 1.000000000000000000, 0.8660254037844387076, 1.000000000000000000, 0.8660254037844387076, 1.000000000000000000, 0.8660254037844387076, 1.000000000000000000, 0.8660254037844387076, 1.000000000000000000, 0.8660254037844387076, 1.000000000000000000, 0.8660254037844387076, 1.000000000000000000, 0.8660254037844387076, 1.000000000000000000, 0.8660254037844387076, 1.000000000000000000, 0.8660254037844387076, 1.000000000000000000, 0.8660254037844387076, 1.000000000000000000, 0.8660254037844387076, 1.000000000000000000, 0.8660254037844387076, 1.000000000000000000, 0.8660254037844387076, 1.000000000000000000, 0.8660254037844387076, 1.000000000000000000, 0.8660254037844387076, 1.000000000000000000, 0.8660254037844387076, 1.000000000000000000, 0.8660254037844387076, 1.000000000000000000, 0.8660254037844387076, 1.000000000000000000, 0.8660254037844387076, 1.000000000000000000, 0.8660254037844387076, 1.000000000000000000, 0.8660254037844387076, 1.000000000000000000, 0.8660254037844387076, 1.000000000000000000, 0.8660254037844387076, 1.000000000000000000, 0.8660254037844387076, 1.000000000000000000, 0.8660254037844387076, 1.000000000000000000, 0.8660254037844387076, 1.000000000000000000, 0.8660254037844387076, 1.000000000000000000, 0.8660254037844387076, 1.000000000000000000, 0.8660254037844387076, 1.000000000000000000, 0.8660254037844387076, 1.000000000000000000, 0.8660254037844387076, 1.000000000000000000, 0.8660254037844387076, 1.000000000000000000, 0.8660254037844387076, 1.000000000000000000, 0.8660254037844387076, 1.000000000000000000, 0.8660254037844387076, 1.000000000000000000, 0.8660254037844387076, 1.000000000000000000, 0.8660254037844387076, 1.000000000000000000, 0.8660254037844387076, 1.000000000000000000, 0.8660254037844387076, 1.000000000000000000, 0.8660254037844387076, 1.000000000000000000, 0.8660254037844387076, 1.000000000000000000, 0.8660254037844387076, 1.000000000000000000, 0.8660254037844387076, 1.000000000000000000, 0.8660254037844387076, 1.000000000000000000, 0.8660254037844387076, 1.000000000000000000, 0.8660254037844387076, 1.000000000000000000, 0.8660254037844387076, 1.000000000000000000, 0.8660254037844387076, 1.000000000000000000, 0.8660254037844387076, 1.000000000000000000, 0.8660254037844387076, 1.000000000000000000, 0.8660254037844387076, 1.000000000000000000, 0.8660254037844387076, 1.000000000000000000, 0.8660254037844387076, 1.000000000000000000, 0.8660254037844387076, 1.000000000000000000, 0.8660254037844387076, 1.000000000000000000, 0.8660254037844387076, 1.000000000000000000, 0.8660254037844387076, 1.000000000000000000, 0.8660254037844387076, 1.000000000000000000, 0.8660254037844387076, 1.000000000000000000, 0.8660254037844387076, 1.000000000000000000, 0.8660254037844387076, 1.000000000000000000, 0.8660254037844387076, 1.000000000000000000, 0.8660254037844387076, 1.000000000000000000, 0.8660254037844387076, 1.000000000000000000, 0.8660254037844387076, 1.000000000000000000, 0.8660254037844387076, 1.000000000000000000, 0.8660254037844387076, 1.000000000000000000, 0.8660254037844387076, 1.000000000000000000, 0.8660254037844387076, 1.000000000000000000, 0.8660254037844387076, 1.000000000000000000, 0.8660254037844387076, 1.000000000000000000, 0.8660254037844387076, 1.000000000000000000, 0.8660254037844387076, 1.000000000000000000, 0.8660254037844387076, 1.000000000000000000, 0.8660254037844387076, 1.000000000000000000, 0.8660254037844387076, 1.000000000000000000, 0.8660254037844387076, 1.000000000000000000, 0.8660254037844387076, 1.000000000000000000, 0.8660254037844387076, 1.000000000000000000, 0.8660254037844387076, 1.000000000000000000, 0.8660254037844387076, 1.000000000000000000, 0.8660254037844387076, 1.000000000000000000, 0.8660254037844387076, 1.000000000000000000, 0.8660254037844387076, 1.000000000000000000, 0.8660254037844387076, 1.000000000000000000, 0.8660254037844387076, 1.000000000000000000, 0.8660254037844387076, 1.000000000000000000, 0.8660254037844387076, 1.000000000000000000, 0.8660254037844387076, 1.000000000000000000, 0.8660254037844387076, 1.000000000000000000, 0.8660254037844387076, 1.000000000000000000, 0.8660254037844387076, 1.000000000000000000, 0.8660254037844387076, 1.000000000000000000, 0.8660254037844387076, 1.000000000000000000, 0.8660254037844387076, 1.000000000000000000, 0.8660254037844387076, 1.000000000000000000, 0.8660254037844387076, 1.000000000000000000, 0.8660254037844387076, 1.000000000000000000, 0.8660254037844387076, 1.000000000000000000, 0.8660254037844387076, 1.000000000000000000, 0.8660254037844387076, 1.000000000000000000, 0.8660254037844387076, 1.000000000000000000, 0.8660254037844387076, 1.000000000000000000, 0.8660254037844387076, 1.000000000000000000, 0.8660254037844387076, 1.000000000000000000, 0.8660254037844387076, 1.000000000000000000, 0.8660254037844387076, 1.000000000000000000, 0.8660254037844387076, 1.000000000000000000, 0.8660254037844387076, 1.000000000000000000, 0.8660254037844387076, 1.000000000000000000, 0.8660254037844387076, 1.000000000000000000, 0.8660254037844387076, 1.000000000000000000, 0.8660254037844387076, 1.000000000000000000, 0.8660254037844387076, 1.000000000000000000, 0.8660254037844387076, 1.000000000000000000, 0.8660254037844387076, 1.000000000000000000, 0.8660254037844387076, 1.000000000000000000, 0.8660254037844387076, 1.000000000000000000, 0.8660254037844387076, 1.000000000000000000, 0.8660254037844387076, 1.000000000000000000, 0.8660254037844387076, 1.000000000000000000, 0.8660254037844387076, 1.000000000000000000, 0.8660254037844387076, 1.000000000000000000, 0.8660254037844387076, 1.000000000000000000, 0.8660254037844387076, 1.000000000000000000, 0.8660254037844387076, 1.000000000000000000, 0.8660254037844387076, 1.000000000000000000, 0.8660254037844387076, 1.000000000000000000, 0.8660254037844387076, 1.000000000000000000, 0.8660254037844387076, 1.000000000000000000, 0.8660254037844387076, 1.000000000000000000, 0.8660254037844387076, 1.000000000000000000, 0.8660254037844387076, 1.000000000000000000, 0.8660254037844387076, 1.000000000000000000, 0.8660254037844387076, 1.000000000000000000, 0.8660254037844387076, 1.000000000000000000, 0.8660254037844387076, 1.000000000000000000, 0.8660254037844387076, 1.000000000000000000, 0.8660254037844387076, 1.000000000000000000, 0.8660254037844387076, 1.000000000000000000, 0.8660254037844387076, 1.000000000000000000, 0.8660254037844387076, 1.000000000000000000, 0.8660254037844387076, 1.000000000000000000, 0.8660254037844387076, 1.000000000000000000, 0.8660254037844387076, 1.000000000000000000, 0.8660254037844387076, 1.000000000000000000, 0.8660254037844387076, 1.000000000000000000, 0.8660254037844387076, 1.000000000000000000, 0.8660254037844387076, 1.000000000000000000, 0.8660254037844387076, 1.000000000000000000, 0.8660254037844387076, 1.000000000000000000, 0.8660254037844387076, 1.000000000000000000, 0.8660254037844387076, 1.000000000000000000, 0.8660254037844387076, 1.000000000000000000, 0.8660254037844387076, 1.000000000000000000, 0.8660254037844387076, 1.000000000000000000, 0.8660254037844387076, 1.000000000000000000, 0.8660254037844387076, 1.000000000000000000, 0.8660254037844387076, 1.000000000000000000, 0.8660254037844387076, 1.000000000000000000, 0.8660254037844387076, 1.000000000000000000, 0.8660254037844387076, 1.000000000000000000, 0.8660254037844387076, 1.000000000000000000, 0.8660254037844387076, 1.000000000000000000, 0.8660254037844387076, 1.000000000000000000, 0.8660254037844387076, 1.000000000000000000, 0.8660254037844387076, 1.000000000000000000, 0.8660254037844387076, 1.000000000000000000, 0.8660254037844387076, 1.000000000000000000, 0.8660254037844387076, 1.000000000000000000, 0.8660254037844387076, 1.000000000000000000, 0.8660254037844387076, 1.000000000000000000, 0.8660254037844387076, 1.000000000000000000, 0.8660254037844387076, 1.000000000000000000, 0.8660254037844387076, 1.000000000000000000, 0.8660254037844387076, 1.000000000000000000, 0.8660254037844387076, 1.000000000000000000, 0.8660254037844387076, 1.000000000000000000, 0.8660254037844387076, 1.000000000000000000, 0.8660254037844387076, 1.000000000000000000, 0.8660254037844387076, 1.000000000000000000, 0.8660254037844387076, 1.000000000000000000, 0.8660254037844387076, 1.000000000000000000, 0.8660254037844387076, 1.000000000000000000, 0.8660254037844387076, 1.000000000000000000, 0.8660254037844387076, 1.000000000000000000, 0.8660254037844387076, 1.000000000000000000, 0.8660254037844387076, 1.000000000000000000, 0.8660254037844387076, 1.000000000000000000, 0.8660254037844387076, 1.000000000000000000, 0.8660254037844387076, 1.000000000000000000, 0.8660254037844387076, 1.000000000000000000, 0.8660254037844387076, 1.000000000000000000, 0.8660254037844387076, 1.000000000000000000, 0.8660254037844387076, 1.000000000000000000, 0.8660254037844387076, 1.000000000000000000, 0.8660254037844387076, 1.000000000000000000, 0.8660254037844387076, 1.000000000000000000, 0.8660254037844387076, 1.000000000000000000, 0.8660254037844387076, 1.000000000000000000, 0.8660254037844387076, 1.000000000000000000, 0.8660254037844387076, 1.000000000000000000, 0.8660254037844387076, 1.000000000000000000, 0.8660254037844387076, 1.000000000000000000, 0.8660254037844387076, 1.000000000000000000, 0.8660254037844387076, 1.000000000000000000, 0.8660254037844387076, 1.000000000000000000, 0.8660254037844387076, 1.000000000000000000, 0.8660254037844387076, 1.000000000000000000, 0.8660254037844387076, 1.000000000000000000, 0.8660254037844387076, 1.000000000000000000, 0.8660254037844387076, 1.000000000000000000, 0.8660254037844387076, 1.000000000000000000, 0.8660254037844387076, 1.000000000000000000, 0.8660254037844387076, 1.000000000000000000, 0.8660254037844387076, 1.000000000000000000, 0.8660254037844387076, 1.000000000000000000, 0.8660254037844387076, 1.000000000000000000, 0.8660254037844387076, 1.000000000000000000, 0.8660254037844387076, 1.000000000000000000, 0.8660254037844387076, 1.000000000000000000, 0.8660254037844387076, 1.000000000000000000, 0.8660254037844387076, 1.000000000000000000, 0.8660254037844387076, 1.000000000000000000, 0.8660254037844387076, 1.000000000000000000, 0.8660254037844387076, 1.000000000000000000, 0.8660254037844387076, 1.000000000000000000, 0.8660254037844387076, 1.000000000000000000, 0.8660254037844387076, 1.000000000000000000, 0.8660254037844387076, 1.000000000000000000, 0.8660254037844387076, 1.000000000000000000, 0.8660254037844387076, 1.000000000000000000, 0.8660254037844387076, 1.000000000000000000, 0.8660254037844387076, 1.000000000000000000, 0.8660254037844387076, 1.000000000000000000, 0.8660254037844387076, 1.000000000000000000, 0.8660254037844387076, 1.000000000000000000, 0.8660254037844387076, 1.000000000000000000, 0.8660254037844387076, 1.000000000000000000, 0.8660254037844387076, 1.000000000000000000, 0.8660254037844387076, 1.000000000000000000, 0.8660254037844387076, 1.000000000000000000, 0.8660254037844387076, 1.000000000000000000, 0.8660254037844387076, 1.000000000000000000, 0.8660254037844387076, 1.000000000000000000, 0.8660254037844387076, 1.000000000000000000, 0.8660254037844387076, 1.000000000000000000, 0.8660254037844387076, 1.000000000000000000, 0.8660254037844387076, 1.000000000000000000, 0.8660254037844387076, 1.000000000000000000, 0.8660254037844387076, 1.000000000000000000, 0.8660254037844387076, 1.000000000000000000, 0.8660254037844387076, 1.000000000000000000, 0.8660254037844387076, 1.000000000000000000, 0.8660254037844387076, 1.000000000000000000, 0.8660254037844387076, 1.000000000000000000) ) ) 
 REPRESENTATION_ITEM ( '' )  SURFACE ( )  );
#9623=CARTESIAN_POINT ( 'NONE',  ( 20.18437500061451217, 5.492252693125287522, 3.363034840372157021E-16 ) ) ;
#9626=CARTESIAN_POINT ( 'NONE',  ( 7.321875000614517681, -4.119189519843968306, 2.378215178124996054 ) ) ;
#9637=CARTESIAN_POINT ( 'NONE',  ( 9.271875000614517859, 5.824947211148865298E-16, -4.756430356249998326 ) ) ;
#9644=CARTESIAN_POINT ( 'NONE',  ( 14.62500000000000000, 4.330127018922191873, 2.499999999999999556 ) ) ;
#9660=CARTESIAN_POINT ( 'NONE',  ( 16.17187500061451644, 2.746126346562645981, -4.756430356249997438 ) ) ;
#9691=CARTESIAN_POINT ( 'NONE',  ( 20.82187500061451857, 2.746126346562643317, 4.756430356249998326 ) ) ;
#9697=CARTESIAN_POINT ( 'NONE',  ( 21.97500000000000142, -4.330127018922194537, 2.499999999999995559 ) ) ;
#9699=CARTESIAN_POINT ( 'NONE',  ( 20.77500000000000213, 6.123233995736764310E-16, -4.999999999999998224 ) ) ;
#9700=CARTESIAN_POINT ( 'NONE',  ( 24.01875000122903359, 2.886751345948142866, -4.999999999999973355 ) ) ;
#9707=CARTESIAN_POINT ( 'NONE',  ( 28.88437500061451502, -2.746126346562646425, 4.756430356249996549 ) ) ;
#9709=CARTESIAN_POINT ( 'NONE',  ( 14.10937500061451644, -5.492252693125287522, -1.008910452111647106E-15 ) ) ;
#9715=ADVANCED_FACE ( 'NONE', ( #11042 ), #27315, .T. ) ;
#9720=CARTESIAN_POINT ( 'NONE',  ( 8.146875000614516082, 0.000000000000000000, 4.756430356249998326 ) ) ;
#9735=CARTESIAN_POINT ( 'NONE',  ( 29.55000000000000071, 0.000000000000000000, 4.999999999999998224 ) ) ;
#9742=CARTESIAN_POINT ( 'NONE',  ( 24.00937500061451502, 0.000000000000000000, 4.756430356249998326 ) ) ;
#9744=CARTESIAN_POINT ( 'NONE',  ( 8.221875000614518925, 2.746126346562643317, 4.756430356249998326 ) ) ;
#9753=DIRECTION ( 'NONE',  ( -1.000000000000000000, -0.000000000000000000, -0.000000000000000000 ) ) ;
#9756=SHAPE_DEFINITION_REPRESENTATION ( #20177, #25944 ) ;
#9761=CARTESIAN_POINT ( 'NONE',  ( 18.24375000122903501, 5.773502691896255534, 3.535250795749688894E-16 ) ) ;
#9764=VERTEX_POINT ( 'NONE', #28397 ) ;
#9777=CARTESIAN_POINT ( 'NONE',  ( 28.02187500061451431, 2.746126346562643317, 4.756430356249998326 ) ) ;
#9795=CARTESIAN_POINT ( 'NONE',  ( 20.63437500061451502, 5.492252693125287522, 3.363034840372157021E-16 ) ) ;
#9811=CARTESIAN_POINT ( 'NONE',  ( 19.20000000000000284, 0.000000000000000000, 4.999999999999998224 ) ) ;
#9814=CARTESIAN_POINT ( 'NONE',  ( 14.14687500061451431, -4.119189519843965641, -2.378215178125001383 ) ) ;
#9822=ORIENTED_EDGE ( 'NONE', *, *, #47475, .T. ) ;
#9835=CARTESIAN_POINT ( 'NONE',  ( 15.87187500061451573, 2.746126346562643317, 4.756430356249998326 ) ) ;
#9852=CARTESIAN_POINT ( 'NONE',  ( 24.91875000122902861, 2.886751345948129099, -4.999999999999998224 ) ) ;
#9864=CARTESIAN_POINT ( 'NONE',  ( 45.00000000000000000, 6.123233995736764310E-16, -4.999999999999998224 ) ) ;
#9877=CARTESIAN_POINT ( 'NONE',  ( 26.45625000122903003, 0.000000000000000000, 4.999999999999998224 ) ) ;
#9894=EDGE_LOOP ( 'NONE', ( #48810, #60628, #27456, #29996 ) ) ;
#9897=CARTESIAN_POINT ( 'NONE',  ( 22.32187500061451502, 5.824947211148865298E-16, -4.756430356249998326 ) ) ;
#9907=CARTESIAN_POINT ( 'NONE',  ( 12.30000000000000249, 4.330127018922192761, -2.499999999999997780 ) ) ;
#9914=CARTESIAN_POINT ( 'NONE',  ( 23.14687500061451786, -2.746126346562646425, 4.756430356249996549 ) ) ;
#9932=DIRECTION ( 'NONE',  ( -1.000000000000000000, -0.000000000000000000, -0.000000000000000000 ) ) ;
#9938=CARTESIAN_POINT ( 'NONE',  ( 10.65937500061451715, -4.119189519843965641, -2.378215178125001383 ) ) ;
#9960=ORIENTED_EDGE ( 'NONE', *, *, #16624, .T. ) ;
#9963=CARTESIAN_POINT ( 'NONE',  ( 10.95937500061451964, 0.000000000000000000, 4.756430356249998326 ) ) ;
#9967=EDGE_CURVE ( 'NONE', #18378, #5961, #21389, .T. ) ;
#9984=CARTESIAN_POINT ( 'NONE',  ( 19.47187500061451360, -4.119189519843968306, 2.378215178124996054 ) ) ;
#9985=VECTOR ( 'NONE', #49874, 1000.000000000000000 ) ;
#9988=CARTESIAN_POINT ( 'NONE',  ( 15.01875000122903181, 2.886751345948129099, -4.999999999999998224 ) ) ;
#9990=CARTESIAN_POINT ( 'NONE',  ( 7.284375000614518036, -2.746126346562646425, 4.756430356249996549 ) ) ;
#10002=CARTESIAN_POINT ( 'NONE',  ( 8.109375000614516438, 2.746126346562643317, 4.756430356249998326 ) ) ;
#10023=CARTESIAN_POINT ( 'NONE',  ( 17.78437500061451715, -4.119189519843968306, 2.378215178124996054 ) ) ;
#10039=EDGE_LOOP ( 'NONE', ( #52253, #19611, #5090, #49545 ) ) ;
#10049=AXIS2_PLACEMENT_3D ( 'NONE', #57208, #5532, #50243 ) ;
#10056=ORIENTED_EDGE ( 'NONE', *, *, #56020, .F. ) ;
#10060=CARTESIAN_POINT ( 'NONE',  ( 18.27187500061451431, -5.492252693125287522, -1.008910452111647106E-15 ) ) ;
#10067=CARTESIAN_POINT ( 'NONE',  ( 18.82500000000000284, -4.330127018922194537, 2.499999999999995559 ) ) ;
#10070=CARTESIAN_POINT ( 'NONE',  ( 45.00000000000000000, 0.000000000000000000, 0.000000000000000000 ) ) ;
#10073=CARTESIAN_POINT ( 'NONE',  ( 17.43750000000000000, -2.886751345948130876, 4.999999999999996447 ) ) ;
#10077=CARTESIAN_POINT ( 'NONE',  ( 27.42187500061451289, 4.119189519843966529, 2.378215178124999607 ) ) ;
#10079=CARTESIAN_POINT ( 'NONE',  ( 12.98437500061451289, 5.492252693125287522, 3.363034840372157021E-16 ) ) ;
#10086=CARTESIAN_POINT ( 'NONE',  ( 45.00000000000000000, 0.000000000000000000, 0.000000000000000000 ) ) ;
#10105=CARTESIAN_POINT ( 'NONE',  ( 29.39999999999999858, 4.330127018922192761, -2.499999999999997780 ) ) ;
#10112=CARTESIAN_POINT ( 'NONE',  ( 24.68437500061451573, 5.824947211148865298E-16, -4.756430356249998326 ) ) ;
#10119=ORIENTED_EDGE ( 'NONE', *, *, #50679, .T. ) ;
#10131=CARTESIAN_POINT ( 'NONE',  ( 18.95625000122903003, -4.330127018922190985, -2.500000000000001332 ) ) ;
#10134=ORIENTED_EDGE ( 'NONE', *, *, #48422, .F. ) ;
#10148=CARTESIAN_POINT ( 'NONE',  ( 26.89687500061451431, -2.746126346562642428, -4.756430356249999214 ) ) ;
#10161=DIRECTION ( 'NONE',  ( -1.000000000000000000, -0.000000000000000000, -0.000000000000000000 ) ) ;
#10163=CARTESIAN_POINT ( 'NONE',  ( 11.94375000122903252, 5.773502691896255534, 3.535250795749688894E-16 ) ) ;
#10167=CARTESIAN_POINT ( 'NONE',  ( 21.94687500061451146, 4.119189519843966529, -2.378215178124998275 ) ) ;
#10177=EDGE_LOOP ( 'NONE', ( #58165, #17633, #34372, #40085 ) ) ;
#10183=CARTESIAN_POINT ( 'NONE',  ( 11.02500000000000036, 4.330127018922191873, 2.499999999999999556 ) ) ;
#10184=CARTESIAN_POINT ( 'NONE',  ( 15.12187500061451573, 5.824947211148865298E-16, -4.756430356249998326 ) ) ;
#10200=CARTESIAN_POINT ( 'NONE',  ( 16.35937500061451644, 0.000000000000000000, 4.756430356249998326 ) ) ;
#10220=CARTESIAN_POINT ( 'NONE',  ( 26.83125000122903003, 4.330127018922191873, 2.499999999999999556 ) ) ;
#10232=DIRECTION ( 'NONE',  ( 0.000000000000000000, 0.000000000000000000, 1.000000000000000000 ) ) ;
#10268=CARTESIAN_POINT ( 'NONE',  ( 22.35937500061451644, 2.746126346562645981, -4.756430356249997438 ) ) ;
#10275=CARTESIAN_POINT ( 'NONE',  ( 26.77499999999999858, 4.330127018922191873, 2.499999999999999556 ) ) ;
#10277=CARTESIAN_POINT ( 'NONE',  ( 12.03749999999999964, -2.886751345948129988, 4.999999999999997335 ) ) ;
#10286=CARTESIAN_POINT ( 'NONE',  ( 21.57187500061451502, 2.746126346562645981, -4.756430356249997438 ) ) ;
#10306=CARTESIAN_POINT ( 'NONE',  ( 10.13437500061451679, -4.119189519843968306, 2.378215178124996054 ) ) ;
#10316=VERTEX_POINT ( 'NONE', #12129 ) ;
#10329=CARTESIAN_POINT ( 'NONE',  ( 12.27187500061451786, 2.746126346562643317, 4.756430356249998326 ) ) ;
#10340=CYLINDRICAL_SURFACE ( 'NONE', #3120, 4.999999999999998224 ) ;
#10351=CARTESIAN_POINT ( 'NONE',  ( 20.89687500061451786, -4.119189519843965641, -2.378215178125001383 ) ) ;
#10354=CARTESIAN_POINT ( 'NONE',  ( 13.74375000122903323, 5.773502691896255534, 3.535250795749688894E-16 ) ) ;
#10366=ADVANCED_FACE ( 'NONE', ( #47563 ), #64548, .T. ) ;
#10369=CARTESIAN_POINT ( 'NONE',  ( 28.69687500061451502, -2.746126346562642428, -4.756430356249999214 ) ) ;
#10374=DIRECTION ( 'NONE',  ( 0.000000000000000000, 0.000000000000000000, 1.000000000000000000 ) ) ;
#10390=CARTESIAN_POINT ( 'NONE',  ( 16.99687500061451573, -2.746126346562641984, -4.756430356249999214 ) ) ;
#10417=CARTESIAN_POINT ( 'NONE',  ( 14.36249999999999893, -5.773502691896255534, -1.060575238724906372E-15 ) ) ;
#10422=CARTESIAN_POINT ( 'NONE',  ( 17.93437500061451928, 5.824947211148865298E-16, -4.756430356249998326 ) ) ;
#10429=CARTESIAN_POINT ( 'NONE',  ( 21.03750000000000142, -2.886751345948129988, 4.999999999999997335 ) ) ;
#10432=CARTESIAN_POINT ( 'NONE',  ( 24.09375000122903288, 5.773502691896255534, 3.535250795749688401E-16 ) ) ;
#10435=CARTESIAN_POINT ( 'NONE',  ( 24.29999999999999716, -4.330127018922190985, -2.500000000000001332 ) ) ;
#10439=CARTESIAN_POINT ( 'NONE',  ( 28.13437500061451502, -2.746126346562642428, -4.756430356249999214 ) ) ;
#10441=CARTESIAN_POINT ( 'NONE',  ( 14.59687500061451537, -4.119189519843965641, -2.378215178125001383 ) ) ;
#10444=ORIENTED_EDGE ( 'NONE', *, *, #15050, .T. ) ;
#10451=CARTESIAN_POINT ( 'NONE',  ( 17.98125000122903572, -4.330127018922194537, 2.499999999999995559 ) ) ;
#10452=CARTESIAN_POINT ( 'NONE',  ( 18.71249999999999503, 2.886751345948182834, 4.999999999999902300 ) ) ;
#10453=VERTEX_POINT ( 'NONE', #31302 ) ;
#10475=CARTESIAN_POINT ( 'NONE',  ( 25.47187500061451715, -5.492252693125287522, -1.008910452111647106E-15 ) ) ;
#10477=CARTESIAN_POINT ( 'NONE',  ( 8.034375000614518925, 5.824947211148865298E-16, -4.756430356249998326 ) ) ;
#10487=( BOUNDED_CURVE ( )  B_SPLINE_CURVE ( 2, ( #4058, #60180, #26216, #70551, #3327, #64637, #14023 ),
 .UNSPECIFIED., .F., .F. ) 
 B_SPLINE_CURVE_WITH_KNOTS ( ( 3, 2, 2, 3 ),
 ( 0.6100000000000002087, 0.6133333333333333970, 0.6166666666666668073, 0.6199999999999999956 ),
 .UNSPECIFIED. ) 
 CURVE ( )  GEOMETRIC_REPRESENTATION_ITEM ( )  RATIONAL_B_SPLINE_CURVE ( ( 0.9999999999999911182, 0.8660254037844475894, 1.000000000000000000, 0.8660254037844387076, 1.000000000000000000, 0.8660254037844387076, 1.000000000000000000 ) ) 
 REPRESENTATION_ITEM ( '' )  );
#10496=CARTESIAN_POINT ( 'NONE',  ( 19.59375000122903288, 5.773502691896255534, 3.535250795749688894E-16 ) ) ;
#10510=( BOUNDED_CURVE ( )  B_SPLINE_CURVE ( 2, ( #41321, #36131, #19486, #24673, #29861, #47220, #41674 ),
 .UNSPECIFIED., .F., .F. ) 
 B_SPLINE_CURVE_WITH_KNOTS ( ( 3, 2, 2, 3 ),
 ( 0.02999999999999993991, 0.03333333333333331899, 0.03666666666666669461, 0.04000000000000007022 ),
 .UNSPECIFIED. ) 
 CURVE ( )  GEOMETRIC_REPRESENTATION_ITEM ( )  RATIONAL_B_SPLINE_CURVE ( ( 1.000000000000002442, 0.8660254037844364872, 1.000000000000000000, 0.8660254037844387076, 1.000000000000000000, 0.8660254037844359321, 1.000000000000002887 ) ) 
 REPRESENTATION_ITEM ( '' )  );
#10513=CARTESIAN_POINT ( 'NONE',  ( 26.59687500061451360, 5.492252693125287522, 3.363034840372157021E-16 ) ) ;
#10526=CARTESIAN_POINT ( 'NONE',  ( 11.23125000122903216, -4.330127018922194537, 2.499999999999995559 ) ) ;
#10530=CARTESIAN_POINT ( 'NONE',  ( 19.84687500061451360, 0.000000000000000000, 4.756430356249998326 ) ) ;
#10535=FACE_OUTER_BOUND ( 'NONE', #69101, .T. ) ;
#10540=CARTESIAN_POINT ( 'NONE',  ( 11.97187500061451537, 5.824947211148865298E-16, -4.756430356249998326 ) ) ;
#10545=ORIENTED_EDGE ( 'NONE', *, *, #2122, .T. ) ;
#10549=CARTESIAN_POINT ( 'NONE',  ( 13.99687500061451395, 0.000000000000000000, 4.756430356249998326 ) ) ;
#10555=VERTEX_POINT ( 'NONE', #31673 ) ;
#10562=CARTESIAN_POINT ( 'NONE',  ( 17.13749999999999574, -2.886751345948181946, -4.999999999999904077 ) ) ;
#10566=CARTESIAN_POINT ( 'NONE',  ( 14.03437500061451715, 4.119189519843966529, 2.378215178124999607 ) ) ;
#10574=CARTESIAN_POINT ( 'NONE',  ( 8.025000000000000355, -4.330127018922194537, 2.499999999999995559 ) ) ;
#10577=CARTESIAN_POINT ( 'NONE',  ( 13.14375000122903536, -2.886751345948126435, -5.000000000000000000 ) ) ;
#10585=CARTESIAN_POINT ( 'NONE',  ( 26.56875000122903074, -5.773502691896255534, -1.060575238724906372E-15 ) ) ;
#10597=CARTESIAN_POINT ( 'NONE',  ( 23.90625000122903288, -4.330127018922190985, -2.500000000000001332 ) ) ;
#10609=DIRECTION ( 'NONE',  ( -1.000000000000000000, -0.000000000000000000, -0.000000000000000000 ) ) ;
#10624=ORIENTED_EDGE ( 'NONE', *, *, #44946, .T. ) ;
#10631=CARTESIAN_POINT ( 'NONE',  ( 20.52187500061451786, 5.824947211148865298E-16, -4.756430356249998326 ) ) ;
#10638=DIRECTION ( 'NONE',  ( -0.4999999999999975575, -0.000000000000000000, -0.8660254037844400399 ) ) ;
#10640=CARTESIAN_POINT ( 'NONE',  ( 9.600000000000001421, 4.330127018922192761, -2.499999999999997780 ) ) ;
#10647=CARTESIAN_POINT ( 'NONE',  ( 21.64687500061451786, 5.492252693125287522, 3.363034840372157021E-16 ) ) ;
#10662=CARTESIAN_POINT ( 'NONE',  ( 27.31875000122903430, 2.886751345948098901, 5.000000000000047073 ) ) ;
#10669=CARTESIAN_POINT ( 'NONE',  ( 9.196875000614518569, -2.746126346562646425, 4.756430356249996549 ) ) ;
#10677=ORIENTED_EDGE ( 'NONE', *, *, #7510, .T. ) ;
#10688=ORIENTED_EDGE ( 'NONE', *, *, #16624, .F. ) ;
#10691=CARTESIAN_POINT ( 'NONE',  ( 10.84687500061451892, 5.492252693125287522, 3.363034840372157021E-16 ) ) ;
#10713=CARTESIAN_POINT ( 'NONE',  ( 20.70937500061451786, 2.746126346562643317, 4.756430356249998326 ) ) ;
#10716=CARTESIAN_POINT ( 'NONE',  ( 13.78125000122903288, 4.330127018922191873, 2.499999999999999556 ) ) ;
#10731=CARTESIAN_POINT ( 'NONE',  ( 7.434375000614515727, -2.746126346562642428, -4.756430356249999214 ) ) ;
#10748=CARTESIAN_POINT ( 'NONE',  ( 19.87500000000000000, 6.123233995736764310E-16, -4.999999999999998224 ) ) ;
#10750=EDGE_CURVE ( 'NONE', #67289, #3601, #4697, .T. ) ;
#10752=CARTESIAN_POINT ( 'NONE',  ( 16.43437500061451573, -4.119189519843968306, 2.378215178124996054 ) ) ;
#10783=CARTESIAN_POINT ( 'NONE',  ( 18.87187500061451573, 2.746126346562645981, -4.756430356249997438 ) ) ;
#10788=CARTESIAN_POINT ( 'NONE',  ( 19.38749999999999929, -2.886751345948125991, -5.000000000000000000 ) ) ;
#10791=CARTESIAN_POINT ( 'NONE',  ( 25.13437500061451502, 5.492252693125287522, 3.363034840372157021E-16 ) ) ;
#10792=CARTESIAN_POINT ( 'NONE',  ( 23.98125000122903216, 6.123233995736764310E-16, -4.999999999999998224 ) ) ;
#10795=CARTESIAN_POINT ( 'NONE',  ( 24.37500000000000000, 6.123233995736764310E-16, -4.999999999999998224 ) ) ;
#10796=EDGE_CURVE ( 'NONE', #17653, #48156, #18435, .T. ) ;
#10799=CARTESIAN_POINT ( 'NONE',  ( 26.22187500061451360, -4.119189519843968306, 2.378215178124996054 ) ) ;
#10801=CARTESIAN_POINT ( 'NONE',  ( 12.94687500061451502, 4.119189519843966529, -2.378215178124998275 ) ) ;
#10811=CARTESIAN_POINT ( 'NONE',  ( 18.59999999999999787, 4.330127018922192761, -2.499999999999997780 ) ) ;
#10833=CARTESIAN_POINT ( 'NONE',  ( 23.67187500061451644, -5.492252693125287522, -1.008910452111647106E-15 ) ) ;
#10835=CARTESIAN_POINT ( 'NONE',  ( 7.884375000614517681, -4.119189519843968306, 2.378215178124996054 ) ) ;
#10853=CARTESIAN_POINT ( 'NONE',  ( 19.70625000122903359, 0.000000000000000000, 4.999999999999998224 ) ) ;
#10857=ADVANCED_FACE ( 'NONE', ( #33125 ), #55662, .T. ) ;
#10870=CARTESIAN_POINT ( 'NONE',  ( 25.43437500061451573, -4.119189519843968306, 2.378215178124996054 ) ) ;
#10875=CARTESIAN_POINT ( 'NONE',  ( 26.96249999999999858, -5.773502691896255534, -1.060575238724906372E-15 ) ) ;
#10883=EDGE_CURVE ( 'NONE', #61284, #27013, #33559, .T. ) ;
#10886=CARTESIAN_POINT ( 'NONE',  ( 12.58125000122903359, -4.330127018922194537, 2.499999999999995559 ) ) ;
#10887=CARTESIAN_POINT ( 'NONE',  ( 13.16250000000000142, 2.886751345948129099, -4.999999999999997335 ) ) ;
#10888=DIRECTION ( 'NONE',  ( 0.000000000000000000, 0.000000000000000000, 1.000000000000000000 ) ) ;
#10890=CARTESIAN_POINT ( 'NONE',  ( 21.08437500061451786, 5.492252693125287522, 3.363034840372157021E-16 ) ) ;
#10900=CARTESIAN_POINT ( 'NONE',  ( 12.30937500061451750, -5.492252693125287522, -1.008910452111647106E-15 ) ) ;
#10901=ORIENTED_EDGE ( 'NONE', *, *, #10796, .F. ) ;
#10915=ORIENTED_EDGE ( 'NONE', *, *, #55179, .F. ) ;
#10922=CARTESIAN_POINT ( 'NONE',  ( 17.17500000000000071, 6.123233995736764310E-16, -4.999999999999998224 ) ) ;
#10924=CARTESIAN_POINT ( 'NONE',  ( 29.74687500061451573, 0.000000000000000000, 4.756430356249998326 ) ) ;
#10925=CARTESIAN_POINT ( 'NONE',  ( 14.29687500061451821, -2.746126346562642428, -4.756430356249999214 ) ) ;
#10933=CARTESIAN_POINT ( 'NONE',  ( 7.987500000000000711, -2.886751345948130876, 4.999999999999996447 ) ) ;
#10934=ADVANCED_BREP_SHAPE_REPRESENTATION ( '', ( #45331, #23765 ), #1386 ) ;
#10946=CARTESIAN_POINT ( 'NONE',  ( 25.36875000122903501, 2.886751345948129099, -4.999999999999998224 ) ) ;
#10948=CARTESIAN_POINT ( 'NONE',  ( 9.806250001229033231, 0.000000000000000000, 4.999999999999998224 ) ) ;
#10958=CARTESIAN_POINT ( 'NONE',  ( 23.86875000122903501, -5.773502691896255534, -1.060575238724906372E-15 ) ) ;
#10969=DIRECTION ( 'NONE',  ( 0.000000000000000000, 0.000000000000000000, 1.000000000000000000 ) ) ;
#10973=EDGE_CURVE ( 'NONE', #42476, #59817, #63740, .T. ) ;
#10986=ORIENTED_EDGE ( 'NONE', *, *, #5278, .F. ) ;
#10993=CARTESIAN_POINT ( 'NONE',  ( 20.63437500061451502, 5.492252693125287522, 3.363034840372157021E-16 ) ) ;
#11004=CARTESIAN_POINT ( 'NONE',  ( 11.17500000000000071, -4.330127018922194537, 2.499999999999995559 ) ) ;
#11011=CARTESIAN_POINT ( 'NONE',  ( 23.40937500061451715, 4.119189519843966529, -2.378215178124998275 ) ) ;
#11042=FACE_OUTER_BOUND ( 'NONE', #71756, .T. ) ;
#11051=CARTESIAN_POINT ( 'NONE',  ( 17.17500000000000071, 6.123233995736764310E-16, -4.999999999999998224 ) ) ;
#11052=CARTESIAN_POINT ( 'NONE',  ( 11.63437500061451857, 5.824947211148865298E-16, -4.756430356249998326 ) ) ;
#11057=( BOUNDED_CURVE ( )  B_SPLINE_CURVE ( 2, ( #61575, #67504, #56048, #50867, #32786, #45694, #4717 ),
 .UNSPECIFIED., .F., .F. ) 
 B_SPLINE_CURVE_WITH_KNOTS ( ( 3, 2, 2, 3 ),
 ( 0.1499999999999999944, 0.1533333333333333215, 0.1566666666666666485, 0.1599999999999999756 ),
 .UNSPECIFIED. ) 
 CURVE ( )  GEOMETRIC_REPRESENTATION_ITEM ( )  RATIONAL_B_SPLINE_CURVE ( ( 1.000000000000000000, 0.8660254037844387076, 1.000000000000000000, 0.8660254037844387076, 1.000000000000000000, 0.8660254037844398178, 0.9999999999999988898 ) ) 
 REPRESENTATION_ITEM ( '' )  );
#11058=ADVANCED_FACE ( 'NONE', ( #11330 ), #38681, .T. ) ;
#11063=CARTESIAN_POINT ( 'NONE',  ( 12.15000000000000036, -4.330127018922190985, -2.500000000000001332 ) ) ;
#11071=DIRECTION ( 'NONE',  ( -1.000000000000000000, -0.000000000000000000, -0.000000000000000000 ) ) ;
#11073=CARTESIAN_POINT ( 'NONE',  ( 19.88437500061451502, -2.746126346562646425, 4.756430356249996549 ) ) ;
#11076=CARTESIAN_POINT ( 'NONE',  ( 13.55625000122903323, -4.330127018922190985, -2.500000000000001332 ) ) ;
#11084=CARTESIAN_POINT ( 'NONE',  ( 15.88125000122903074, 6.123233995736764310E-16, -4.999999999999998224 ) ) ;
#11091=CARTESIAN_POINT ( 'NONE',  ( 7.734375000614518214, -2.746126346562646425, 4.756430356249996549 ) ) ;
#11113=CARTESIAN_POINT ( 'NONE',  ( 14.03437500061451715, 4.119189519843966529, 2.378215178124999607 ) ) ;
#11141=CARTESIAN_POINT ( 'NONE',  ( 14.43749999999999645, -2.886751345948181946, -4.999999999999904077 ) ) ;
#11147=CARTESIAN_POINT ( 'NONE',  ( 18.15937500061451715, 0.000000000000000000, 4.756430356249998326 ) ) ;
#11154=CARTESIAN_POINT ( 'NONE',  ( 20.36249999999999716, 2.886751345948129099, -4.999999999999998224 ) ) ;
#11157=VECTOR ( 'NONE', #16685, 1000.000000000000000 ) ;
#11159=CARTESIAN_POINT ( 'NONE',  ( 25.39687500061451431, -4.119189519843965641, -2.378215178125001383 ) ) ;
#11167=CARTESIAN_POINT ( 'NONE',  ( 26.89687500061451431, 4.119189519843966529, -2.378215178124998275 ) ) ;
#11169=CARTESIAN_POINT ( 'NONE',  ( 12.45937500061451786, 2.746126346562645981, -4.756430356249997438 ) ) ;
#11172=EDGE_LOOP ( 'NONE', ( #27130, #67871, #42453, #57056 ) ) ;
#11178=CARTESIAN_POINT ( 'NONE',  ( 20.68125000122903145, -4.330127018922194537, 2.499999999999995559 ) ) ;
#11203=CARTESIAN_POINT ( 'NONE',  ( 25.02187500061451431, -5.492252693125287522, -1.008910452111647106E-15 ) ) ;
#11210=ORIENTED_EDGE ( 'NONE', *, *, #55404, .F. ) ;
#11220=AXIS2_PLACEMENT_3D ( 'NONE', #19112, #19851, #48312 ) ;
#11224=CARTESIAN_POINT ( 'NONE',  ( 17.23125000122903572, 6.123233995736764310E-16, -4.999999999999998224 ) ) ;
#11241=CARTESIAN_POINT ( 'NONE',  ( 26.14687500061451431, 5.492252693125287522, 3.363034840372157021E-16 ) ) ;
#11246=CARTESIAN_POINT ( 'NONE',  ( 26.39999999999999858, 0.000000000000000000, 4.999999999999998224 ) ) ;
#11257=CARTESIAN_POINT ( 'NONE',  ( 12.46875000122902932, 2.886751345948126879, 4.999999999999999112 ) ) ;
#11261=CARTESIAN_POINT ( 'NONE',  ( 19.62187500061451573, 5.824947211148865298E-16, -4.756430356249998326 ) ) ;
#11264=ORIENTED_EDGE ( 'NONE', *, *, #1743, .T. ) ;
#11273=CARTESIAN_POINT ( 'NONE',  ( 12.64687500061451786, 0.000000000000000000, 4.756430356249998326 ) ) ;
#11281=CARTESIAN_POINT ( 'NONE',  ( 19.12500000000000000, 4.330127018922191873, 2.499999999999999556 ) ) ;
#11297=CARTESIAN_POINT ( 'NONE',  ( 29.67187500061451644, 4.119189519843966529, 2.378215178124999607 ) ) ;
#11298=CARTESIAN_POINT ( 'NONE',  ( 11.93437500061451573, -4.119189519843968306, 2.378215178124996054 ) ) ;
#11306=LINE ( 'NONE', #39020, #13566 ) ;
#11308=CARTESIAN_POINT ( 'NONE',  ( 29.15625000122903288, 0.000000000000000000, 4.999999999999998224 ) ) ;
#11316=CARTESIAN_POINT ( 'NONE',  ( 26.60625000122903216, -4.330127018922190985, -2.500000000000001332 ) ) ;
#11321=CARTESIAN_POINT ( 'NONE',  ( 0.000000000000000000, -4.999999999999999112, 0.000000000000000000 ) ) ;
#11330=FACE_OUTER_BOUND ( 'NONE', #35477, .T. ) ;
#11344=( BOUNDED_CURVE ( )  B_SPLINE_CURVE ( 2, ( #19326, #19696, #18962, #53698, #8266, #52966, #47066 ),
 .UNSPECIFIED., .F., .F. ) 
 B_SPLINE_CURVE_WITH_KNOTS ( ( 3, 2, 2, 3 ),
 ( 0.8699999999999999956, 0.8733333333333332948, 0.8766666666666667052, 0.8800000000000000044 ),
 .UNSPECIFIED. ) 
 CURVE ( )  GEOMETRIC_REPRESENTATION_ITEM ( )  RATIONAL_B_SPLINE_CURVE ( ( 1.000000000000000000, 0.8660254037844387076, 1.000000000000000000, 0.8660254037844387076, 1.000000000000000000, 0.8660254037844387076, 1.000000000000000000 ) ) 
 REPRESENTATION_ITEM ( '' )  );
#11354=CARTESIAN_POINT ( 'NONE',  ( 27.76875000122903359, 2.886751345948119774, 5.000000000000010658 ) ) ;
#11362=CARTESIAN_POINT ( 'NONE',  ( 19.50937500061451857, -5.492252693125287522, -1.008910452111647106E-15 ) ) ;
#11366=DIRECTION ( 'NONE',  ( -1.000000000000000000, -0.000000000000000000, -0.000000000000000000 ) ) ;
#11377=CARTESIAN_POINT ( 'NONE',  ( 22.84687500061451715, -2.746126346562642428, -4.756430356249999214 ) ) ;
#11380=CARTESIAN_POINT ( 'NONE',  ( 20.32499999999999929, 6.123233995736764310E-16, -4.999999999999998224 ) ) ;
#11394=CARTESIAN_POINT ( 'NONE',  ( 45.00000000000000000, 6.123233995736764310E-16, -4.999999999999998224 ) ) ;
#11400=CARTESIAN_POINT ( 'NONE',  ( 8.221875000614518925, 2.746126346562643317, 4.756430356249998326 ) ) ;
#11411=ORIENTED_EDGE ( 'NONE', *, *, #49257, .T. ) ;
#11412=ORIENTED_EDGE ( 'NONE', *, *, #64823, .F. ) ;
#11422=CARTESIAN_POINT ( 'NONE',  ( 9.571875000614518569, 2.746126346562643317, 4.756430356249998326 ) ) ;
#11423=CARTESIAN_POINT ( 'NONE',  ( 45.00000000000000000, 0.000000000000000000, 0.000000000000000000 ) ) ;
#11433=CARTESIAN_POINT ( 'NONE',  ( 9.600000000000001421, 4.330127018922192761, -2.499999999999997780 ) ) ;
#11436=AXIS2_PLACEMENT_3D ( 'NONE', #24316, #1808, #30953 ) ;
#11442=CARTESIAN_POINT ( 'NONE',  ( 17.33437500061451431, -2.746126346562642428, -4.756430356249999214 ) ) ;
#11445=CARTESIAN_POINT ( 'NONE',  ( 13.06875000122903252, -5.773502691896255534, -1.060575238724906372E-15 ) ) ;
#11452=CARTESIAN_POINT ( 'NONE',  ( 15.76875000122903181, -5.773502691896255534, -1.060575238724906372E-15 ) ) ;
#11458=CARTESIAN_POINT ( 'NONE',  ( 29.18437500061451573, 5.824947211148865298E-16, -4.756430356249998326 ) ) ;
#11466=CARTESIAN_POINT ( 'NONE',  ( 10.65000000000000036, 0.000000000000000000, 4.999999999999998224 ) ) ;
#11479=CARTESIAN_POINT ( 'NONE',  ( 13.77187500061451786, -5.492252693125287522, -1.008910452111647106E-15 ) ) ;
#11483=ORIENTED_EDGE ( 'NONE', *, *, #41079, .T. ) ;
#11487=EDGE_CURVE ( 'NONE', #54979, #24521, #70011, .T. ) ;
#11506=ORIENTED_EDGE ( 'NONE', *, *, #17845, .T. ) ;
#11509=CARTESIAN_POINT ( 'NONE',  ( 19.13437500061451857, -4.119189519843968306, 2.378215178124996054 ) ) ;
#11510=CARTESIAN_POINT ( 'NONE',  ( 14.75625000122903252, 0.000000000000000000, 4.999999999999998224 ) ) ;
#11515=CARTESIAN_POINT ( 'NONE',  ( 20.92500000000000071, 4.330127018922191873, 2.499999999999999556 ) ) ;
#11519=CARTESIAN_POINT ( 'NONE',  ( 25.92187500061451644, 5.824947211148865298E-16, -4.756430356249998326 ) ) ;
#11527=CARTESIAN_POINT ( 'NONE',  ( 24.30937500061451573, 2.746126346562643317, 4.756430356249998326 ) ) ;
#11529=CARTESIAN_POINT ( 'NONE',  ( 12.00937500061451502, 2.746126346562645981, -4.756430356249997438 ) ) ;
#11530=ADVANCED_FACE ( 'NONE', ( #17081 ), #46896, .T. ) ;
#11538=VECTOR ( 'NONE', #13168, 1000.000000000000000 ) ;
#11540=CARTESIAN_POINT ( 'NONE',  ( 11.60625000122903216, 0.000000000000000000, 4.999999999999998224 ) ) ;
#11547=EDGE_CURVE ( 'NONE', #64545, #69242, #17443, .T. ) ;
#11564=EDGE_CURVE ( 'NONE', #19922, #42983, #25119, .T. ) ;
#11569=CARTESIAN_POINT ( 'NONE',  ( 20.93437500061451573, -4.119189519843968306, 2.378215178124996054 ) ) ;
#11571=CARTESIAN_POINT ( 'NONE',  ( 25.03125000122903288, 4.330127018922191873, 2.499999999999999556 ) ) ;
#11576=ORIENTED_EDGE ( 'NONE', *, *, #41629, .F. ) ;
#11588=CARTESIAN_POINT ( 'NONE',  ( 15.84375000122903465, -2.886751345948125991, -5.000000000000000000 ) ) ;
#11603=CARTESIAN_POINT ( 'NONE',  ( 26.55937500061451573, 4.119189519843966529, -2.378215178124998275 ) ) ;
#11608=CARTESIAN_POINT ( 'NONE',  ( 26.02499999999999858, -4.330127018922194537, 2.499999999999995559 ) ) ;
#11614=CARTESIAN_POINT ( 'NONE',  ( 23.00625000122903430, -4.330127018922190985, -2.500000000000001332 ) ) ;
#11617=CARTESIAN_POINT ( 'NONE',  ( 11.68125000122903145, -4.330127018922194537, 2.499999999999995559 ) ) ;
#11619=CARTESIAN_POINT ( 'NONE',  ( 24.43125000122903145, 6.123233995736764310E-16, -4.999999999999998224 ) ) ;
#11621=CARTESIAN_POINT ( 'NONE',  ( 18.94687500061451857, 0.000000000000000000, 4.756430356249998326 ) ) ;
#11629=CARTESIAN_POINT ( 'NONE',  ( 10.89375000122903003, -2.886751345948181946, -4.999999999999904077 ) ) ;
#11633=CARTESIAN_POINT ( 'NONE',  ( 13.39687500061451431, 4.119189519843966529, -2.378215178124998275 ) ) ;
#11640=ORIENTED_EDGE ( 'NONE', *, *, #34544, .T. ) ;
#11643=CARTESIAN_POINT ( 'NONE',  ( 10.95000000000000107, 4.330127018922192761, -2.499999999999997780 ) ) ;
#11648=ORIENTED_EDGE ( 'NONE', *, *, #44780, .F. ) ;
#11654=CARTESIAN_POINT ( 'NONE',  ( 29.10937500061451644, -4.119189519843965641, -2.378215178125001383 ) ) ;
#11658=CARTESIAN_POINT ( 'NONE',  ( 13.77187500061451786, -5.492252693125287522, -1.008910452111647106E-15 ) ) ;
#11675=CARTESIAN_POINT ( 'NONE',  ( 23.94375000122903074, -2.886751345948125991, -5.000000000000000000 ) ) ;
#11681=EDGE_CURVE ( 'NONE', #25555, #19407, #39276, .T. ) ;
#11699=CARTESIAN_POINT ( 'NONE',  ( 45.00000000000000000, 6.123233995736764310E-16, -4.999999999999998224 ) ) ;
#11721=CARTESIAN_POINT ( 'NONE',  ( 18.68437500061451573, -2.746126346562642428, -4.756430356249999214 ) ) ;
#11725=CARTESIAN_POINT ( 'NONE',  ( 45.00000000000000000, 6.123233995736764310E-16, -4.999999999999998224 ) ) ;
#11737=CARTESIAN_POINT ( 'NONE',  ( 19.13437500061451857, -4.119189519843968306, 2.378215178124996054 ) ) ;
#11747=FACE_OUTER_BOUND ( 'NONE', #37781, .T. ) ;
#11754=LINE ( 'NONE', #28738, #36215 ) ;
#11760=CARTESIAN_POINT ( 'NONE',  ( 7.734375000614517326, 4.119189519843966529, 2.378215178124999607 ) ) ;
#11770=EDGE_LOOP ( 'NONE', ( #38255, #68411, #63895, #16632 ) ) ;
#11771=ORIENTED_EDGE ( 'NONE', *, *, #29976, .F. ) ;
#11773=DIRECTION ( 'NONE',  ( -1.000000000000000000, -0.000000000000000000, -0.000000000000000000 ) ) ;
#11782=CARTESIAN_POINT ( 'NONE',  ( 9.271875000614516082, -5.492252693125287522, -1.008910452111647106E-15 ) ) ;
#11792=CARTESIAN_POINT ( 'NONE',  ( 12.00000000000000000, 0.000000000000000000, 4.999999999999998224 ) ) ;
#11803=CARTESIAN_POINT ( 'NONE',  ( 17.89687500061451431, 4.119189519843966529, -2.378215178124998275 ) ) ;
#11806=CARTESIAN_POINT ( 'NONE',  ( 25.09687500061451360, 4.119189519843966529, -2.378215178124998275 ) ) ;
#11820=CARTESIAN_POINT ( 'NONE',  ( 27.08437500061451786, 4.119189519843966529, 2.378215178124999607 ) ) ;
#11839=CARTESIAN_POINT ( 'NONE',  ( 13.54687500061451821, 5.492252693125287522, 3.363034840372157021E-16 ) ) ;
#11852=CARTESIAN_POINT ( 'NONE',  ( 29.30625000122903145, -4.330127018922190985, -2.500000000000001332 ) ) ;
#11869=CARTESIAN_POINT ( 'NONE',  ( 15.60937500061451644, -4.119189519843965641, -2.378215178125001383 ) ) ;
#11876=CARTESIAN_POINT ( 'NONE',  ( 16.76249999999999929, 2.886751345948129099, -4.999999999999998224 ) ) ;
#11880=CARTESIAN_POINT ( 'NONE',  ( 24.42187500061451289, -4.119189519843968306, 2.378215178124996054 ) ) ;
#11887=CARTESIAN_POINT ( 'NONE',  ( 25.50937500061451502, 2.746126346562645981, -4.756430356249997438 ) ) ;
#11889=CARTESIAN_POINT ( 'NONE',  ( 12.15937500061451537, 2.746126346562643317, 4.756430356249998326 ) ) ;
#11897=FACE_OUTER_BOUND ( 'NONE', #26436, .T. ) ;
#11898=LINE ( 'NONE', #29256, #851 ) ;
#11901=CARTESIAN_POINT ( 'NONE',  ( 14.03437500061451892, -2.746126346562646425, 4.756430356249996549 ) ) ;
#11912=CARTESIAN_POINT ( 'NONE',  ( 18.97499999999999787, 6.123233995736764310E-16, -4.999999999999998224 ) ) ;
#11922=CARTESIAN_POINT ( 'NONE',  ( 22.92187500061451644, 2.746126346562645981, -4.756430356249997438 ) ) ;
#11924=CARTESIAN_POINT ( 'NONE',  ( 24.99375000122903145, 5.773502691896255534, 3.535250795749688401E-16 ) ) ;
#11929=ORIENTED_EDGE ( 'NONE', *, *, #22798, .T. ) ;
#11942=CARTESIAN_POINT ( 'NONE',  ( 15.43125000122903323, 6.123233995736764310E-16, -4.999999999999998224 ) ) ;
#11954=VERTEX_POINT ( 'NONE', #37263 ) ;
#11958=CARTESIAN_POINT ( 'NONE',  ( 24.53437500061451715, -4.119189519843968306, 2.378215178124996054 ) ) ;
#11964=CARTESIAN_POINT ( 'NONE',  ( 26.84999999999999787, 0.000000000000000000, 4.999999999999998224 ) ) ;
#11967=ADVANCED_FACE ( 'NONE', ( #25071 ), #70145, .T. ) ;
#11974=CARTESIAN_POINT ( 'NONE',  ( 9.693750001229032520, 5.773502691896255534, 3.535250795749688894E-16 ) ) ;
#11978=CARTESIAN_POINT ( 'NONE',  ( 19.50937500061451857, -5.492252693125287522, -1.008910452111647106E-15 ) ) ;
#11989=CARTESIAN_POINT ( 'NONE',  ( 12.12187500061451573, 4.119189519843966529, 2.378215178124999607 ) ) ;
#11990=ORIENTED_EDGE ( 'NONE', *, *, #25258, .T. ) ;
#11996=CARTESIAN_POINT ( 'NONE',  ( 13.72500000000000142, 4.330127018922191873, 2.499999999999999556 ) ) ;
#12009=CARTESIAN_POINT ( 'NONE',  ( 29.67187500061451644, 2.746126346562645981, -4.756430356249997438 ) ) ;
#12012=CARTESIAN_POINT ( 'NONE',  ( 26.82187500061451502, 5.824947211148865298E-16, -4.756430356249998326 ) ) ;
#12013=CARTESIAN_POINT ( 'NONE',  ( 13.32187500061451502, -5.492252693125287522, -1.008910452111647106E-15 ) ) ;
#12029=CARTESIAN_POINT ( 'NONE',  ( 22.29375000122903216, 5.773502691896255534, 3.535250795749688894E-16 ) ) ;
#12037=CARTESIAN_POINT ( 'NONE',  ( 28.94999999999999929, 4.330127018922192761, -2.499999999999997780 ) ) ;
#12039=ADVANCED_FACE ( 'NONE', ( #59785 ), #48357, .T. ) ;
#12074=EDGE_LOOP ( 'NONE', ( #67690, #43712, #6897, #4856, #61410, #3773 ) ) ;
#12081=CARTESIAN_POINT ( 'NONE',  ( 19.05937500061451217, -5.492252693125287522, -1.008910452111647106E-15 ) ) ;
#12097=CARTESIAN_POINT ( 'NONE',  ( 21.15937500061451715, 4.119189519843966529, -2.378215178124998275 ) ) ;
#12100=CARTESIAN_POINT ( 'NONE',  ( 12.67499999999999893, 6.123233995736764310E-16, -4.999999999999998224 ) ) ;
#12108=ORIENTED_EDGE ( 'NONE', *, *, #55155, .T. ) ;
#12118=CARTESIAN_POINT ( 'NONE',  ( 8.634375000614518569, 4.119189519843966529, 2.378215178124999607 ) ) ;
#12129=CARTESIAN_POINT ( 'NONE',  ( 22.18125000122903145, 6.123233995736764310E-16, -4.999999999999998224 ) ) ;
#12133=( BOUNDED_CURVE ( )  B_SPLINE_CURVE ( 2, ( #18297, #23854, #34947, #23495, #63734, #24216, #29764 ),
 .UNSPECIFIED., .F., .F. ) 
 B_SPLINE_CURVE_WITH_KNOTS ( ( 3, 2, 2, 3 ),
 ( 0.3199999999999999512, 0.3233333333333333059, 0.3266666666666666607, 0.3300000000000000711 ),
 .UNSPECIFIED. ) 
 CURVE ( )  GEOMETRIC_REPRESENTATION_ITEM ( )  RATIONAL_B_SPLINE_CURVE ( ( 1.000000000000002220, 0.8660254037844364872, 1.000000000000000000, 0.8660254037844387076, 1.000000000000000000, 0.8660254037844364872, 1.000000000000002220 ) ) 
 REPRESENTATION_ITEM ( '' )  );
#12139=CARTESIAN_POINT ( 'NONE',  ( 10.28437500061451715, 5.824947211148865298E-16, -4.756430356249998326 ) ) ;
#12152=CARTESIAN_POINT ( 'NONE',  ( 8.400000000000000355, 0.000000000000000000, 4.999999999999998224 ) ) ;
#12157=CARTESIAN_POINT ( 'NONE',  ( 17.63437500061451502, -2.746126346562646425, 4.756430356249996549 ) ) ;
#12160=CARTESIAN_POINT ( 'NONE',  ( 26.55937500061451217, 2.746126346562643317, 4.756430356249998326 ) ) ;
#12164=CARTESIAN_POINT ( 'NONE',  ( 26.92499999999999716, -4.330127018922194537, 2.499999999999995559 ) ) ;
#12166=CARTESIAN_POINT ( 'NONE',  ( 20.99999999999999645, 0.000000000000000000, 4.999999999999998224 ) ) ;
#12175=CARTESIAN_POINT ( 'NONE',  ( 27.68437500061451573, -4.119189519843968306, 2.378215178124996054 ) ) ;
#12184=ORIENTED_EDGE ( 'NONE', *, *, #69324, .F. ) ;
#12194=CARTESIAN_POINT ( 'NONE',  ( 15.00937500061451679, 0.000000000000000000, 4.756430356249998326 ) ) ;
#12208=ORIENTED_EDGE ( 'NONE', *, *, #26195, .T. ) ;
#12217=ADVANCED_FACE ( 'NONE', ( #15446 ), #20256, .T. ) ;
#12225=CARTESIAN_POINT ( 'NONE',  ( 16.92187500061451999, -5.492252693125287522, -1.008910452111647106E-15 ) ) ;
#12226=CARTESIAN_POINT ( 'NONE',  ( 21.22500000000000142, 6.123233995736764310E-16, -4.999999999999998224 ) ) ;
#12231=CARTESIAN_POINT ( 'NONE',  ( 17.88749999999999929, -2.886751345948129988, 4.999999999999997335 ) ) ;
#12235=CARTESIAN_POINT ( 'NONE',  ( 26.07187500061451146, 4.119189519843966529, 2.378215178124999607 ) ) ;
#12243=CARTESIAN_POINT ( 'NONE',  ( 23.74687500061451573, 4.119189519843966529, -2.378215178124998275 ) ) ;
#12245=CARTESIAN_POINT ( 'NONE',  ( 10.05937500061451750, -5.492252693125287522, -1.008910452111647106E-15 ) ) ;
#12253=CARTESIAN_POINT ( 'NONE',  ( 26.26875000122903003, 2.886751345948129099, -4.999999999999997335 ) ) ;
#12254=CARTESIAN_POINT ( 'NONE',  ( 34.99999999999999289, 0.000000000000000000, 0.000000000000000000 ) ) ;
#12257=CARTESIAN_POINT ( 'NONE',  ( 11.55937500061451573, 2.746126346562645981, -4.756430356249997438 ) ) ;
#12265=CYLINDRICAL_SURFACE ( 'NONE', #31328, 4.999999999999998224 ) ;
#12272=DIRECTION ( 'NONE',  ( -1.000000000000000000, -0.000000000000000000, -0.000000000000000000 ) ) ;
#12277=CARTESIAN_POINT ( 'NONE',  ( 22.50937500061451857, 4.119189519843966529, -2.378215178124998275 ) ) ;
#12297=CARTESIAN_POINT ( 'NONE',  ( 16.25625000122903074, -4.330127018922190985, -2.500000000000001332 ) ) ;
#12305=CARTESIAN_POINT ( 'NONE',  ( 10.87500000000000000, 6.123233995736764310E-16, -4.999999999999998224 ) ) ;
#12313=CARTESIAN_POINT ( 'NONE',  ( 24.12187500061451217, -5.492252693125287522, -1.008910452111647106E-15 ) ) ;
#12318=CARTESIAN_POINT ( 'NONE',  ( 25.64999999999999858, -4.330127018922190985, -2.500000000000001332 ) ) ;
#12326=CARTESIAN_POINT ( 'NONE',  ( 8.643750001229031810, -2.886751345948125991, -5.000000000000000000 ) ) ;
#12329=CARTESIAN_POINT ( 'NONE',  ( 17.55937500061451573, 2.746126346562643317, 4.756430356249998326 ) ) ;
#12330=VECTOR ( 'NONE', #1342, 1000.000000000000000 ) ;
#12341=CARTESIAN_POINT ( 'NONE',  ( 11.44687500061451679, -4.119189519843965641, -2.378215178125001383 ) ) ;
#12355=CARTESIAN_POINT ( 'NONE',  ( 10.76250000000000107, -5.773502691896255534, -1.060575238724906372E-15 ) ) ;
#12365=CARTESIAN_POINT ( 'NONE',  ( 15.15000000000000036, 0.000000000000000000, 4.999999999999998224 ) ) ;
#12368=CARTESIAN_POINT ( 'NONE',  ( 28.32187500061451502, 4.119189519843966529, 2.378215178124999607 ) ) ;
#12369=CARTESIAN_POINT ( 'NONE',  ( 13.58437500061451786, 4.119189519843966529, 2.378215178124999607 ) ) ;
#12385=CARTESIAN_POINT ( 'NONE',  ( 24.13125000122903074, 4.330127018922191873, 2.499999999999999556 ) ) ;
#12410=( BOUNDED_SURFACE ( )  B_SPLINE_SURFACE ( 1, 2, ( 
 ( #1045, #19088, #40559, #12480, #62358, #30560, #42012, #36097, #54193, #9122, #25750, #13926, #3957, #15019, #9490, #20549, #37557, #32019, #59715, #47548, #36464, #31659, #71176, #36828, #58980, #20186, #48287, #58617, #8753, #70811, #25376, #42741, #65261, #3590, #64900, #26112, #31286, #26480, #47921, #48651, #14290, #43106, #19826, #60079, #14650, #65632, #49021, #8024, #54555, #37191, #8387, #53087, #59342, #2481, #64162, #71551, #41643, #70450, #42378, #13550, #25006, #19452, #70077, #64532, #30916, #53828, #53457, #2847, #3221, #5408, #38284, #55291, #60812, #54921, #10220, #73004, #27215, #32754, #39392, #61911, #11316, #10585, #20925, #44937, #44583, #15382, #32381, #4685, #43477, #33837, #56379, #27945, #5046, #5771, #50837, #38667, #15745, #33112, #49750, #28302, #61191, #55650, #16472, #72278, #66001, #27582, #50478, #21655, #22026, #39030, #67475, #4329, #21290, #10946, #67115, #37924, #50114, #22388, #66745, #26853, #72643, #16838, #44213, #60442, #16115, #9852, #49385, #61544, #33468, #56015, #71916, #43843, #66370, #24188, #23826, #46742, #57082, #29740, #34191, #17912, #52277, #17558, #35640, #46017, #62280, #39763, #12385, #40475, #68554, #57802, #23105, #11675, #69276, #46377, #18638, #6490, #1679, #57448, #45662, #58162, #41202, #63710, #13102, #7566, #30102, #18269, #6127, #68195, #63360, #237, #62990, #40119, #51920, #6852, #67829, #34921, #29386, #29025, #1317, #68911, #40842, #23471, #35280, #12744, #22745, #51561, #7211, #45295, #17202, #961, #56725, #28658, #51197, #600, #62634, #12029, #34554, #24914, #69632, #25281, #18994, #2043, #71087, #65544, #58889, #8299, #48194, #48561, #30470, #20461, #9401, #70717, #30829, #47457, #52999, #13455, #37097, #69990, #13834, #19360, #36003, #41917, #31566, #53362, #64442, #43015, #14931, #37471, #42284, #52637, #3503, #3129, #47100, #64073, #36373, #24554, #59991, #41556, #59622, #36733, #58522, #7932, #70357, #2759, #64808, #47827, #2394, #19734, #14198, #20092, #59255, #8663, #31194, #9036, #53736, #25658, #42649, #26022, #65173, #14564, #54105, #33024, #39306, #16026, #10853, #4597, #26764, #10496, #38574, #26389, #72189, #61098, #15655, #55562, #4958, #72550, #55204, #67026, #21568, #67387, #38194, #21937, #27127, #50025, #10131, #27861, #27491, #16386, #16749, #71460, #50392, #44493, #4237, #48931, #49661, #20836, #54468, #72917, #44851, #60721, #32663, #38941, #22299, #9761, #61819, #31931, #61459, #44122, #49296, #32295, #65913, #33387, #71829, #66277, #21200, #15293, #43752, #55923, #66649, #5319, #3866, #43389, #37832, #60352, #54830, #1231, #45928, #5683, #151, #6039, #11224, #18183, #63267, #6764, #51470, #40752, #33748, #34467, #56644, #28934, #23017, #12659, #56995, #6402, #40383, #507, #56293, #873, #51828, #40032, #62902, #34832, #68826, #17113, #28573, #29298, #12297, #28219, #68460, #35194, #23380, #62192, #17822, #50748, #45575, #22657, #57358, #11588, #34105, #23737, #46285, #45207, #67740, #68106, #51110, #39672, #17472, #62545, #11942, #33604, #61319, #49520, #39524, #50608, #45066, #56148, #12, #67603, #22160, #9988, #72045, #67248, #5542, #72406, #50253, #71690, #66879, #62050, #43980, #28080, #66135, #44712, #4093, #21788, #60951, #32523, #16606, #21062, #15513, #22519, #38803, #26622, #49159, #44354, #55060, #16247, #38055, #21423, #43613, #4461, #26991, #49881, #10716, #10354, #66501, #61677, #33248, #15883, #11076, #16968, #4817, #38428, #55424, #55786, #5177, #39162, #32884, #27713, #60580, #27350, #72776, #11445, #33965, #16057, #44882, #15687, #61489, #50422, #4988, #72948, #22330, #61850, #44525, #56322, #10886, #56672, #27520, #11257, #67058, #39337, #72583, #17145, #67417, #5711, #6070, #60755, #39703, #16779, #66682, #38225, #16417, #10163, #43783, #62221, #34134, #50054, #21967, #33779, #11617, #72221, #28603, #51139, #28247, #38973, #38606, #21599, #55234, #50778, #61131, #55593, #10526, #4629, #33054, #181, #33415, #55954, #21231, #66310, #32697, #5350, #27159, #45237, #22686, #49693, #44153, #27889, #67770, #41499, #13398, #7512, #57748, #64020, #30416, #18213, #68492, #12690, #57389, #35946, #40785, #63298, #69222, #34862, #62577, #904, #68138, #13047, #41148, #35586, #23049, #30043, #45959, #11974, #18583, #23412, #34497, #52583, #7880, #40416, #538, #46684, #17502, #35227, #58467, #62933, #1989, #57025, #63656, #45605, #7155, #6796, #28966, #58105, #40063, #6431, #24500, #29685, #51504, #17856, #68856, #12326, #52222, #29330, #51860, #1262, #23769, #46321, #1626, #24134, #47044, #69578, #18940, #25601, #70303, #59939, #20778, #53678, #47767, #31137, #14510, #54054, #20410, #59200, #59567, #41858, #69935, #24858, #15239, #54413, #26335, #8608, #42594, #14877, #42958, #52944, #25967, #43335, #9346, #70663, #3072, #48508, #8980 ),
 ( #48139, #47405, #31513, #30775, #71035, #65857, #31879, #3814, #71404, #19676, #37416, #8245, #64754, #20039, #48874, #19305, #53306, #64388, #65120, #65487, #14144, #37776, #60296, #9707, #13778, #36320, #37043, #25221, #3449, #2705, #2341, #42229, #58835, #36679, #72863, #55509, #67333, #72492, #67685, #38518, #22246, #4902, #50339, #10439, #28166, #61404, #16693, #17056, #71776, #50693, #5259, #4544, #49242, #27438, #21145, #54774, #95, #45153, #61041, #32969, #27803, #22601, #10077, #39615, #62134, #44800, #49968, #27073, #32608, #66220, #39251, #49604, #66591, #72131, #15598, #21511, #11167, #21877, #44064, #32241, #4179, #26708, #44438, #43699, #56236, #55872, #38140, #60664, #15968, #55146, #66967, #16332, #61763, #38887, #10799, #33334, #33691, #5629, #23684, #68406, #24412, #29244, #51776, #7071, #45873, #18857, #1176, #69138, #40328, #12608, #29600, #35500, #45518, #11887, #1539, #35142, #41418, #68772, #63576, #57306, #68049, #46232, #12963, #28875, #46961, #6711, #449, #51053, #18128, #40694, #63212, #18497, #34412, #22958, #58020, #57665, #7430, #17768, #41062, #52136, #56940, #69497, #29956, #52497, #1907, #11527, #34048, #24049, #17418, #6344, #46596, #56588, #5984, #39977, #51414, #28514, #62489, #816, #23324, #62849, #12243, #34774, #63934, #14789, #14424, #58381, #2260, #53218, #13319, #31793, #3725, #70950, #48056, #54332, #20689, #8522, #58748, #2983, #47677, #26250, #31051, #53588, #59481, #25136, #71313, #25511, #48424, #19587, #65033, #8893, #37330, #24774, #64301, #53965, #36959, #35858, #70581, #42875, #36594, #47318, #19957, #65398, #8158, #48787, #59115, #52860, #30331, #42509, #31425, #3363, #20321, #13690, #69851, #59854, #25884, #9258, #70213, #7793, #19218, #36234, #41772, #30687, #2615, #42143, #64670, #14055, #61316, #49156, #15510, #33245, #72773, #37687, #4090, #38052, #66876, #60210, #10351, #72403, #26988, #21785, #44351, #10713, #66498, #5174, #32881, #5539, #49517, #55783, #15880, #27710, #21420, #39159, #16244, #50250, #28077, #9623, #61674, #38800, #60577, #32155, #38425, #54688, #65768, #11073, #56145, #72042, #43977, #22157, #33601, #21059, #50605, #9, #44709, #60948, #9984, #43610, #26619, #67245, #32520, #4458, #55057, #71687, #55421, #16603, #4814, #27347, #43248, #15150, #66132, #49878, #18410, #68687, #67959, #39521, #68324, #62047, #45063, #40976, #35412, #28786, #51327, #18047, #63491, #360, #12879, #52410, #40605, #729, #17332, #22867, #56501, #6985, #39891, #56852, #62404, #5894, #11803, #1455, #23238, #34320, #57937, #7344, #29874, #12157, #22516, #46509, #46147, #16965, #33962, #6258, #67600, #11442, #28427, #29516, #6629, #50964, #45425, #40245, #45789, #34685, #17684, #62766, #57216, #29158, #63126, #51690, #1094, #23602, #52051, #12522, #35055, #57582, #69048, #23961, #2174, #64944, #2891, #9166, #59026, #53874, #47593, #35773, #19500, #3266, #19132, #37238, #70122, #63844, #41334, #13968, #42057, #64580, #59388, #24687, #13235, #25794, #25422, #48332, #58663, #31333, #8428, #47231, #59759, #70857, #42783, #20231, #65304, #14694, #19870, #7704, #69764, #14336, #31701, #69413, #58296, #41686, #47965, #18768, #36506, #30964, #8071, #53499, #70493, #42423, #25050, #36870, #8798, #1818, #30603, #24325, #46874, #30239, #53131, #52772, #64209, #13598, #36144, #2530, #16071, #72963, #34149, #72599, #17517, #27903, #43156, #20597, #67433, #22345, #50438, #39719, #5003, #66699, #6085, #5727, #28617, #38988, #11633, #39352, #27537, #40078, #51154, #23065, #56686, #555, #45620, #196, #61145, #50069, #45253, #68154, #48696, #38621, #21982, #28262, #71219, #44897, #11273, #61503, #33794, #56337, #22701, #5365, #17160, #16795, #62593, #10900, #67786, #61866, #62237, #33428, #11989, #50793, #54236, #3633, #10540, #26157, #33068, #44541, #55607, #67072, #16430, #55971, #52958, #47419, #40800, #63313, #30060, #30430, #12341, #2355, #64402, #52598, #12704, #6810, #34876, #68508, #18955, #51876, #68870, #1275, #17871, #23784, #13413, #35241, #46336, #24872, #69949, #19319, #24147, #34512, #58483, #58119, #28982, #45974, #18226, #57041, #41873, #6447, #41515, #18598, #51520, #919, #52236, #29344, #46700, #57762, #23428, #1641, #69236, #2004, #7171, #40430, #41162, #64034, #29699, #35600, #24515, #7893, #62947, #57405, #47059, #7527, #63671, #13061, #69593, #35962, #49255, #15252, #60309, #42606, #3461, #48886, #54426, #13795, #59951, #4192, #20792, #31525, #14522, #9358, #20422, #3826, #26721, #37789, #54065, #71789, #8621, #36335, #8259, #58849, #20051, #43349, #26347, #71416, #65871, #25981, #9720, #42243, #8993, #30789, #42970, #64767, #31891, #21158, #32253, #54786, #43711, #31150, #53320, #14157, #25614, #48520, #2719, #25235, #36691, #47781, #71047, #70315, #48150, #19690, #59213 ) ),
 .UNSPECIFIED., .F., .F., .F. ) 
 B_SPLINE_SURFACE_WITH_KNOTS ( ( 2, 2 ),
 ( 3, 2, 2, 2, 2, 2, 2, 2, 2, 2, 2, 2, 2, 2, 2, 2, 2, 2, 2, 2, 2, 2, 2, 2, 2, 2, 2, 2, 2, 2, 2, 2, 2, 2, 2, 2, 2, 2, 2, 2, 2, 2, 2, 2, 2, 2, 2, 2, 2, 2, 2, 2, 2, 2, 2, 2, 2, 2, 2, 2, 2, 2, 2, 2, 2, 2, 2, 2, 2, 2, 2, 2, 2, 2, 2, 2, 2, 2, 2, 2, 2, 2, 2, 2, 2, 2, 2, 2, 2, 2, 2, 2, 2, 2, 2, 2, 2, 2, 2, 2, 2, 2, 2, 2, 2, 2, 2, 2, 2, 2, 2, 2, 2, 2, 2, 2, 2, 2, 2, 2, 2, 2, 2, 2, 2, 2, 2, 2, 2, 2, 2, 2, 2, 2, 2, 2, 2, 2, 2, 2, 2, 2, 2, 2, 2, 2, 2, 2, 2, 2, 2, 2, 2, 2, 2, 2, 2, 2, 2, 2, 2, 2, 2, 2, 2, 2, 2, 2, 2, 2, 2, 2, 2, 2, 2, 2, 2, 2, 2, 2, 2, 2, 2, 2, 2, 2, 2, 2, 2, 2, 2, 2, 2, 2, 2, 2, 2, 2, 2, 2, 2, 2, 2, 2, 2, 2, 2, 2, 2, 2, 2, 2, 2, 2, 2, 2, 2, 2, 2, 2, 2, 2, 2, 2, 2, 2, 2, 2, 2, 2, 2, 2, 2, 2, 2, 2, 2, 2, 2, 2, 2, 2, 2, 2, 2, 2, 2, 2, 2, 2, 2, 2, 2, 2, 2, 2, 2, 2, 2, 2, 2, 2, 2, 2, 2, 2, 2, 2, 2, 2, 2, 2, 2, 2, 2, 2, 2, 2, 2, 2, 2, 2, 2, 2, 2, 2, 2, 2, 2, 2, 2, 2, 2, 2, 2, 2, 2, 2, 2, 2, 3 ),
 ( 0.000000000000000000, 1.000000000000000000 ),
 ( 0.000000000000000000, 0.003333333333333333547, 0.006666666666666667095, 0.01000000000000000021, 0.01333333333333333419, 0.01666666666666666644, 0.02000000000000000042, 0.02333333333333333440, 0.02666666666666666838, 0.02999999999999999889, 0.03333333333333333287, 0.03666666666666666685, 0.04000000000000000083, 0.04333333333333333481, 0.04666666666666666879, 0.05000000000000000278, 0.05333333333333333676, 0.05666666666666666380, 0.05999999999999999778, 0.06333333333333333870, 0.06666666666666666574, 0.07000000000000000666, 0.07333333333333333370, 0.07666666666666666075, 0.08000000000000000167, 0.08333333333333332871, 0.08666666666666666963, 0.08999999999999999667, 0.09333333333333333759, 0.09666666666666666463, 0.1000000000000000056, 0.1033333333333333326, 0.1066666666666666735, 0.1100000000000000006, 0.1133333333333333276, 0.1166666666666666685, 0.1199999999999999956, 0.1233333333333333365, 0.1266666666666666774, 0.1300000000000000044, 0.1333333333333333315, 0.1366666666666666585, 0.1400000000000000133, 0.1433333333333333404, 0.1466666666666666674, 0.1499999999999999944, 0.1533333333333333215, 0.1566666666666666763, 0.1600000000000000033, 0.1633333333333333304, 0.1666666666666666574, 0.1700000000000000122, 0.1733333333333333393, 0.1766666666666666663, 0.1799999999999999933, 0.1833333333333333204, 0.1866666666666666752, 0.1900000000000000022, 0.1933333333333333293, 0.1966666666666666563, 0.2000000000000000111, 0.2033333333333333381, 0.2066666666666666652, 0.2099999999999999922, 0.2133333333333333470, 0.2166666666666666741, 0.2200000000000000011, 0.2233333333333333282, 0.2266666666666666552, 0.2300000000000000100, 0.2333333333333333370, 0.2366666666666666641, 0.2399999999999999911, 0.2433333333333333459, 0.2466666666666666730, 0.2500000000000000000, 0.2533333333333333548, 0.2566666666666666541, 0.2600000000000000089, 0.2633333333333333082, 0.2666666666666666630, 0.2700000000000000178, 0.2733333333333333171, 0.2766666666666666718, 0.2800000000000000266, 0.2833333333333333259, 0.2866666666666666807, 0.2899999999999999800, 0.2933333333333333348, 0.2966666666666666896, 0.2999999999999999889, 0.3033333333333333437, 0.3066666666666666430, 0.3099999999999999978, 0.3133333333333333526, 0.3166666666666666519, 0.3200000000000000067, 0.3233333333333333059, 0.3266666666666666607, 0.3300000000000000155, 0.3333333333333333148, 0.3366666666666666696, 0.3400000000000000244, 0.3433333333333333237, 0.3466666666666666785, 0.3499999999999999778, 0.3533333333333333326, 0.3566666666666666874, 0.3599999999999999867, 0.3633333333333333415, 0.3666666666666666408, 0.3699999999999999956, 0.3733333333333333504, 0.3766666666666666496, 0.3800000000000000044, 0.3833333333333333592, 0.3866666666666666585, 0.3900000000000000133, 0.3933333333333333126, 0.3966666666666666674, 0.4000000000000000222, 0.4033333333333333215, 0.4066666666666666763, 0.4099999999999999756, 0.4133333333333333304, 0.4166666666666666852, 0.4199999999999999845, 0.4233333333333333393, 0.4266666666666666941, 0.4299999999999999933, 0.4333333333333333481, 0.4366666666666666474, 0.4400000000000000022, 0.4433333333333333570, 0.4466666666666666563, 0.4500000000000000111, 0.4533333333333333104, 0.4566666666666666652, 0.4600000000000000200, 0.4633333333333333193, 0.4666666666666666741, 0.4699999999999999734, 0.4733333333333333282, 0.4766666666666666829, 0.4799999999999999822, 0.4833333333333333370, 0.4866666666666666918, 0.4899999999999999911, 0.4933333333333333459, 0.4966666666666666452, 0.5000000000000000000, 0.5033333333333332993, 0.5066666666666667096, 0.5100000000000000089, 0.5133333333333333082, 0.5166666666666667185, 0.5200000000000000178, 0.5233333333333333171, 0.5266666666666666163, 0.5300000000000000266, 0.5333333333333333259, 0.5366666666666666252, 0.5400000000000000355, 0.5433333333333333348, 0.5466666666666666341, 0.5500000000000000444, 0.5533333333333333437, 0.5566666666666666430, 0.5600000000000000533, 0.5633333333333333526, 0.5666666666666666519, 0.5699999999999999512, 0.5733333333333333615, 0.5766666666666666607, 0.5799999999999999600, 0.5833333333333333703, 0.5866666666666666696, 0.5899999999999999689, 0.5933333333333333792, 0.5966666666666666785, 0.5999999999999999778, 0.6033333333333333881, 0.6066666666666666874, 0.6099999999999999867, 0.6133333333333332860, 0.6166666666666666963, 0.6199999999999999956, 0.6233333333333332948, 0.6266666666666667052, 0.6300000000000000044, 0.6333333333333333037, 0.6366666666666667140, 0.6400000000000000133, 0.6433333333333333126, 0.6466666666666666119, 0.6500000000000000222, 0.6533333333333333215, 0.6566666666666666208, 0.6600000000000000311, 0.6633333333333333304, 0.6666666666666666297, 0.6700000000000000400, 0.6733333333333333393, 0.6766666666666666385, 0.6800000000000000488, 0.6833333333333333481, 0.6866666666666666474, 0.6899999999999999467, 0.6933333333333333570, 0.6966666666666666563, 0.6999999999999999556, 0.7033333333333333659, 0.7066666666666666652, 0.7099999999999999645, 0.7133333333333333748, 0.7166666666666666741, 0.7199999999999999734, 0.7233333333333333837, 0.7266666666666666829, 0.7299999999999999822, 0.7333333333333332815, 0.7366666666666666918, 0.7399999999999999911, 0.7433333333333332904, 0.7466666666666667007, 0.7500000000000000000, 0.7533333333333332993, 0.7566666666666667096, 0.7600000000000000089, 0.7633333333333333082, 0.7666666666666667185, 0.7700000000000000178, 0.7733333333333333171, 0.7766666666666666163, 0.7800000000000000266, 0.7833333333333333259, 0.7866666666666666252, 0.7900000000000000355, 0.7933333333333333348, 0.7966666666666666341, 0.8000000000000000444, 0.8033333333333333437, 0.8066666666666666430, 0.8100000000000000533, 0.8133333333333333526, 0.8166666666666666519, 0.8199999999999999512, 0.8233333333333333615, 0.8266666666666666607, 0.8299999999999999600, 0.8333333333333333703, 0.8366666666666666696, 0.8399999999999999689, 0.8433333333333333792, 0.8466666666666666785, 0.8499999999999999778, 0.8533333333333333881, 0.8566666666666666874, 0.8599999999999999867, 0.8633333333333332860, 0.8666666666666666963, 0.8699999999999999956, 0.8733333333333332948, 0.8766666666666667052, 0.8800000000000000044, 0.8833333333333333037, 0.8866666666666667140, 0.8900000000000000133, 0.8933333333333333126, 0.8966666666666666119, 0.9000000000000000222, 0.9033333333333333215, 0.9066666666666666208, 0.9100000000000000311, 0.9133333333333333304, 0.9166666666666666297, 0.9200000000000000400, 0.9233333333333333393, 0.9266666666666666385, 0.9300000000000000488, 0.9333333333333333481, 0.9366666666666666474, 0.9399999999999999467, 0.9433333333333333570, 0.9466666666666666563, 0.9499999999999999556, 0.9533333333333333659, 0.9566666666666666652, 0.9599999999999999645, 0.9633333333333333748, 0.9666666666666666741, 0.9699999999999999734, 0.9733333333333333837, 0.9766666666666666829, 0.9799999999999999822, 0.9833333333333332815, 0.9866666666666666918, 0.9899999999999999911, 0.9933333333333332904, 0.9966666666666667007, 1.000000000000000000 ),
 .UNSPECIFIED. ) 
 GEOMETRIC_REPRESENTATION_ITEM ( )  RATIONAL_B_SPLINE_SURFACE ( (
 ( 1.000000000000000000, 0.8660254037844387076, 1.000000000000000000, 0.8660254037844387076, 1.000000000000000000, 0.8660254037844387076, 1.000000000000000000, 0.8660254037844387076, 1.000000000000000000, 0.8660254037844387076, 1.000000000000000000, 0.8660254037844387076, 1.000000000000000000, 0.8660254037844387076, 1.000000000000000000, 0.8660254037844387076, 1.000000000000000000, 0.8660254037844387076, 1.000000000000000000, 0.8660254037844387076, 1.000000000000000000, 0.8660254037844387076, 1.000000000000000000, 0.8660254037844387076, 1.000000000000000000, 0.8660254037844387076, 1.000000000000000000, 0.8660254037844387076, 1.000000000000000000, 0.8660254037844387076, 1.000000000000000000, 0.8660254037844387076, 1.000000000000000000, 0.8660254037844387076, 1.000000000000000000, 0.8660254037844387076, 1.000000000000000000, 0.8660254037844387076, 1.000000000000000000, 0.8660254037844387076, 1.000000000000000000, 0.8660254037844387076, 1.000000000000000000, 0.8660254037844387076, 1.000000000000000000, 0.8660254037844387076, 1.000000000000000000, 0.8660254037844387076, 1.000000000000000000, 0.8660254037844387076, 1.000000000000000000, 0.8660254037844387076, 1.000000000000000000, 0.8660254037844387076, 1.000000000000000000, 0.8660254037844387076, 1.000000000000000000, 0.8660254037844387076, 1.000000000000000000, 0.8660254037844387076, 1.000000000000000000, 0.8660254037844387076, 1.000000000000000000, 0.8660254037844387076, 1.000000000000000000, 0.8660254037844387076, 1.000000000000000000, 0.8660254037844387076, 1.000000000000000000, 0.8660254037844387076, 1.000000000000000000, 0.8660254037844387076, 1.000000000000000000, 0.8660254037844387076, 1.000000000000000000, 0.8660254037844387076, 1.000000000000000000, 0.8660254037844387076, 1.000000000000000000, 0.8660254037844387076, 1.000000000000000000, 0.8660254037844387076, 1.000000000000000000, 0.8660254037844387076, 1.000000000000000000, 0.8660254037844387076, 1.000000000000000000, 0.8660254037844387076, 1.000000000000000000, 0.8660254037844387076, 1.000000000000000000, 0.8660254037844387076, 1.000000000000000000, 0.8660254037844387076, 1.000000000000000000, 0.8660254037844387076, 1.000000000000000000, 0.8660254037844387076, 1.000000000000000000, 0.8660254037844387076, 1.000000000000000000, 0.8660254037844387076, 1.000000000000000000, 0.8660254037844387076, 1.000000000000000000, 0.8660254037844387076, 1.000000000000000000, 0.8660254037844387076, 1.000000000000000000, 0.8660254037844387076, 1.000000000000000000, 0.8660254037844387076, 1.000000000000000000, 0.8660254037844387076, 1.000000000000000000, 0.8660254037844387076, 1.000000000000000000, 0.8660254037844387076, 1.000000000000000000, 0.8660254037844387076, 1.000000000000000000, 0.8660254037844387076, 1.000000000000000000, 0.8660254037844387076, 1.000000000000000000, 0.8660254037844387076, 1.000000000000000000, 0.8660254037844387076, 1.000000000000000000, 0.8660254037844387076, 1.000000000000000000, 0.8660254037844387076, 1.000000000000000000, 0.8660254037844387076, 1.000000000000000000, 0.8660254037844387076, 1.000000000000000000, 0.8660254037844387076, 1.000000000000000000, 0.8660254037844387076, 1.000000000000000000, 0.8660254037844387076, 1.000000000000000000, 0.8660254037844387076, 1.000000000000000000, 0.8660254037844387076, 1.000000000000000000, 0.8660254037844387076, 1.000000000000000000, 0.8660254037844387076, 1.000000000000000000, 0.8660254037844387076, 1.000000000000000000, 0.8660254037844387076, 1.000000000000000000, 0.8660254037844387076, 1.000000000000000000, 0.8660254037844387076, 1.000000000000000000, 0.8660254037844387076, 1.000000000000000000, 0.8660254037844387076, 1.000000000000000000, 0.8660254037844387076, 1.000000000000000000, 0.8660254037844387076, 1.000000000000000000, 0.8660254037844387076, 1.000000000000000000, 0.8660254037844387076, 1.000000000000000000, 0.8660254037844387076, 1.000000000000000000, 0.8660254037844387076, 1.000000000000000000, 0.8660254037844387076, 1.000000000000000000, 0.8660254037844387076, 1.000000000000000000, 0.8660254037844387076, 1.000000000000000000, 0.8660254037844387076, 1.000000000000000000, 0.8660254037844387076, 1.000000000000000000, 0.8660254037844387076, 1.000000000000000000, 0.8660254037844387076, 1.000000000000000000, 0.8660254037844387076, 1.000000000000000000, 0.8660254037844387076, 1.000000000000000000, 0.8660254037844387076, 1.000000000000000000, 0.8660254037844387076, 1.000000000000000000, 0.8660254037844387076, 1.000000000000000000, 0.8660254037844387076, 1.000000000000000000, 0.8660254037844387076, 1.000000000000000000, 0.8660254037844387076, 1.000000000000000000, 0.8660254037844387076, 1.000000000000000000, 0.8660254037844387076, 1.000000000000000000, 0.8660254037844387076, 1.000000000000000000, 0.8660254037844387076, 1.000000000000000000, 0.8660254037844387076, 1.000000000000000000, 0.8660254037844387076, 1.000000000000000000, 0.8660254037844387076, 1.000000000000000000, 0.8660254037844387076, 1.000000000000000000, 0.8660254037844387076, 1.000000000000000000, 0.8660254037844387076, 1.000000000000000000, 0.8660254037844387076, 1.000000000000000000, 0.8660254037844387076, 1.000000000000000000, 0.8660254037844387076, 1.000000000000000000, 0.8660254037844387076, 1.000000000000000000, 0.8660254037844387076, 1.000000000000000000, 0.8660254037844387076, 1.000000000000000000, 0.8660254037844387076, 1.000000000000000000, 0.8660254037844387076, 1.000000000000000000, 0.8660254037844387076, 1.000000000000000000, 0.8660254037844387076, 1.000000000000000000, 0.8660254037844387076, 1.000000000000000000, 0.8660254037844387076, 1.000000000000000000, 0.8660254037844387076, 1.000000000000000000, 0.8660254037844387076, 1.000000000000000000, 0.8660254037844387076, 1.000000000000000000, 0.8660254037844387076, 1.000000000000000000, 0.8660254037844387076, 1.000000000000000000, 0.8660254037844387076, 1.000000000000000000, 0.8660254037844387076, 1.000000000000000000, 0.8660254037844387076, 1.000000000000000000, 0.8660254037844387076, 1.000000000000000000, 0.8660254037844387076, 1.000000000000000000, 0.8660254037844387076, 1.000000000000000000, 0.8660254037844387076, 1.000000000000000000, 0.8660254037844387076, 1.000000000000000000, 0.8660254037844387076, 1.000000000000000000, 0.8660254037844387076, 1.000000000000000000, 0.8660254037844387076, 1.000000000000000000, 0.8660254037844387076, 1.000000000000000000, 0.8660254037844387076, 1.000000000000000000, 0.8660254037844387076, 1.000000000000000000, 0.8660254037844387076, 1.000000000000000000, 0.8660254037844387076, 1.000000000000000000, 0.8660254037844387076, 1.000000000000000000, 0.8660254037844387076, 1.000000000000000000, 0.8660254037844387076, 1.000000000000000000, 0.8660254037844387076, 1.000000000000000000, 0.8660254037844387076, 1.000000000000000000, 0.8660254037844387076, 1.000000000000000000, 0.8660254037844387076, 1.000000000000000000, 0.8660254037844387076, 1.000000000000000000, 0.8660254037844387076, 1.000000000000000000, 0.8660254037844387076, 1.000000000000000000, 0.8660254037844387076, 1.000000000000000000, 0.8660254037844387076, 1.000000000000000000, 0.8660254037844387076, 1.000000000000000000, 0.8660254037844387076, 1.000000000000000000, 0.8660254037844387076, 1.000000000000000000, 0.8660254037844387076, 1.000000000000000000, 0.8660254037844387076, 1.000000000000000000, 0.8660254037844387076, 1.000000000000000000, 0.8660254037844387076, 1.000000000000000000, 0.8660254037844387076, 1.000000000000000000, 0.8660254037844387076, 1.000000000000000000, 0.8660254037844387076, 1.000000000000000000, 0.8660254037844387076, 1.000000000000000000, 0.8660254037844387076, 1.000000000000000000, 0.8660254037844387076, 1.000000000000000000, 0.8660254037844387076, 1.000000000000000000, 0.8660254037844387076, 1.000000000000000000, 0.8660254037844387076, 1.000000000000000000, 0.8660254037844387076, 1.000000000000000000, 0.8660254037844387076, 1.000000000000000000, 0.8660254037844387076, 1.000000000000000000, 0.8660254037844387076, 1.000000000000000000, 0.8660254037844387076, 1.000000000000000000, 0.8660254037844387076, 1.000000000000000000, 0.8660254037844387076, 1.000000000000000000, 0.8660254037844387076, 1.000000000000000000, 0.8660254037844387076, 1.000000000000000000, 0.8660254037844387076, 1.000000000000000000, 0.8660254037844387076, 1.000000000000000000, 0.8660254037844387076, 1.000000000000000000, 0.8660254037844387076, 1.000000000000000000, 0.8660254037844387076, 1.000000000000000000, 0.8660254037844387076, 1.000000000000000000, 0.8660254037844387076, 1.000000000000000000, 0.8660254037844387076, 1.000000000000000000, 0.8660254037844387076, 1.000000000000000000, 0.8660254037844387076, 1.000000000000000000, 0.8660254037844387076, 1.000000000000000000, 0.8660254037844387076, 1.000000000000000000, 0.8660254037844387076, 1.000000000000000000, 0.8660254037844387076, 1.000000000000000000, 0.8660254037844387076, 1.000000000000000000, 0.8660254037844387076, 1.000000000000000000, 0.8660254037844387076, 1.000000000000000000, 0.8660254037844387076, 1.000000000000000000, 0.8660254037844387076, 1.000000000000000000, 0.8660254037844387076, 1.000000000000000000, 0.8660254037844387076, 1.000000000000000000, 0.8660254037844387076, 1.000000000000000000, 0.8660254037844387076, 1.000000000000000000, 0.8660254037844387076, 1.000000000000000000, 0.8660254037844387076, 1.000000000000000000, 0.8660254037844387076, 1.000000000000000000, 0.8660254037844387076, 1.000000000000000000, 0.8660254037844387076, 1.000000000000000000, 0.8660254037844387076, 1.000000000000000000, 0.8660254037844387076, 1.000000000000000000, 0.8660254037844387076, 1.000000000000000000, 0.8660254037844387076, 1.000000000000000000, 0.8660254037844387076, 1.000000000000000000, 0.8660254037844387076, 1.000000000000000000, 0.8660254037844387076, 1.000000000000000000, 0.8660254037844387076, 1.000000000000000000, 0.8660254037844387076, 1.000000000000000000, 0.8660254037844387076, 1.000000000000000000, 0.8660254037844387076, 1.000000000000000000, 0.8660254037844387076, 1.000000000000000000, 0.8660254037844387076, 1.000000000000000000, 0.8660254037844387076, 1.000000000000000000, 0.8660254037844387076, 1.000000000000000000, 0.8660254037844387076, 1.000000000000000000, 0.8660254037844387076, 1.000000000000000000, 0.8660254037844387076, 1.000000000000000000, 0.8660254037844387076, 1.000000000000000000, 0.8660254037844387076, 1.000000000000000000, 0.8660254037844387076, 1.000000000000000000, 0.8660254037844387076, 1.000000000000000000, 0.8660254037844387076, 1.000000000000000000, 0.8660254037844387076, 1.000000000000000000, 0.8660254037844387076, 1.000000000000000000, 0.8660254037844387076, 1.000000000000000000, 0.8660254037844387076, 1.000000000000000000, 0.8660254037844387076, 1.000000000000000000, 0.8660254037844387076, 1.000000000000000000, 0.8660254037844387076, 1.000000000000000000, 0.8660254037844387076, 1.000000000000000000, 0.8660254037844387076, 1.000000000000000000, 0.8660254037844387076, 1.000000000000000000, 0.8660254037844387076, 1.000000000000000000, 0.8660254037844387076, 1.000000000000000000, 0.8660254037844387076, 1.000000000000000000, 0.8660254037844387076, 1.000000000000000000, 0.8660254037844387076, 1.000000000000000000, 0.8660254037844387076, 1.000000000000000000, 0.8660254037844387076, 1.000000000000000000, 0.8660254037844387076, 1.000000000000000000, 0.8660254037844387076, 1.000000000000000000, 0.8660254037844387076, 1.000000000000000000, 0.8660254037844387076, 1.000000000000000000, 0.8660254037844387076, 1.000000000000000000, 0.8660254037844387076, 1.000000000000000000, 0.8660254037844387076, 1.000000000000000000, 0.8660254037844387076, 1.000000000000000000, 0.8660254037844387076, 1.000000000000000000, 0.8660254037844387076, 1.000000000000000000, 0.8660254037844387076, 1.000000000000000000, 0.8660254037844387076, 1.000000000000000000, 0.8660254037844387076, 1.000000000000000000, 0.8660254037844387076, 1.000000000000000000, 0.8660254037844387076, 1.000000000000000000, 0.8660254037844387076, 1.000000000000000000, 0.8660254037844387076, 1.000000000000000000, 0.8660254037844387076, 1.000000000000000000, 0.8660254037844387076, 1.000000000000000000, 0.8660254037844387076, 1.000000000000000000, 0.8660254037844387076, 1.000000000000000000, 0.8660254037844387076, 1.000000000000000000, 0.8660254037844387076, 1.000000000000000000, 0.8660254037844387076, 1.000000000000000000, 0.8660254037844387076, 1.000000000000000000, 0.8660254037844387076, 1.000000000000000000, 0.8660254037844387076, 1.000000000000000000, 0.8660254037844387076, 1.000000000000000000, 0.8660254037844387076, 1.000000000000000000, 0.8660254037844387076, 1.000000000000000000, 0.8660254037844387076, 1.000000000000000000, 0.8660254037844387076, 1.000000000000000000, 0.8660254037844387076, 1.000000000000000000, 0.8660254037844387076, 1.000000000000000000, 0.8660254037844387076, 1.000000000000000000, 0.8660254037844387076, 1.000000000000000000, 0.8660254037844387076, 1.000000000000000000, 0.8660254037844387076, 1.000000000000000000, 0.8660254037844387076, 1.000000000000000000, 0.8660254037844387076, 1.000000000000000000, 0.8660254037844387076, 1.000000000000000000, 0.8660254037844387076, 1.000000000000000000, 0.8660254037844387076, 1.000000000000000000, 0.8660254037844387076, 1.000000000000000000, 0.8660254037844387076, 1.000000000000000000, 0.8660254037844387076, 1.000000000000000000, 0.8660254037844387076, 1.000000000000000000, 0.8660254037844387076, 1.000000000000000000, 0.8660254037844387076, 1.000000000000000000, 0.8660254037844387076, 1.000000000000000000),
 ( 1.000000000000000000, 0.8660254037844387076, 1.000000000000000000, 0.8660254037844387076, 1.000000000000000000, 0.8660254037844387076, 1.000000000000000000, 0.8660254037844387076, 1.000000000000000000, 0.8660254037844387076, 1.000000000000000000, 0.8660254037844387076, 1.000000000000000000, 0.8660254037844387076, 1.000000000000000000, 0.8660254037844387076, 1.000000000000000000, 0.8660254037844387076, 1.000000000000000000, 0.8660254037844387076, 1.000000000000000000, 0.8660254037844387076, 1.000000000000000000, 0.8660254037844387076, 1.000000000000000000, 0.8660254037844387076, 1.000000000000000000, 0.8660254037844387076, 1.000000000000000000, 0.8660254037844387076, 1.000000000000000000, 0.8660254037844387076, 1.000000000000000000, 0.8660254037844387076, 1.000000000000000000, 0.8660254037844387076, 1.000000000000000000, 0.8660254037844387076, 1.000000000000000000, 0.8660254037844387076, 1.000000000000000000, 0.8660254037844387076, 1.000000000000000000, 0.8660254037844387076, 1.000000000000000000, 0.8660254037844387076, 1.000000000000000000, 0.8660254037844387076, 1.000000000000000000, 0.8660254037844387076, 1.000000000000000000, 0.8660254037844387076, 1.000000000000000000, 0.8660254037844387076, 1.000000000000000000, 0.8660254037844387076, 1.000000000000000000, 0.8660254037844387076, 1.000000000000000000, 0.8660254037844387076, 1.000000000000000000, 0.8660254037844387076, 1.000000000000000000, 0.8660254037844387076, 1.000000000000000000, 0.8660254037844387076, 1.000000000000000000, 0.8660254037844387076, 1.000000000000000000, 0.8660254037844387076, 1.000000000000000000, 0.8660254037844387076, 1.000000000000000000, 0.8660254037844387076, 1.000000000000000000, 0.8660254037844387076, 1.000000000000000000, 0.8660254037844387076, 1.000000000000000000, 0.8660254037844387076, 1.000000000000000000, 0.8660254037844387076, 1.000000000000000000, 0.8660254037844387076, 1.000000000000000000, 0.8660254037844387076, 1.000000000000000000, 0.8660254037844387076, 1.000000000000000000, 0.8660254037844387076, 1.000000000000000000, 0.8660254037844387076, 1.000000000000000000, 0.8660254037844387076, 1.000000000000000000, 0.8660254037844387076, 1.000000000000000000, 0.8660254037844387076, 1.000000000000000000, 0.8660254037844387076, 1.000000000000000000, 0.8660254037844387076, 1.000000000000000000, 0.8660254037844387076, 1.000000000000000000, 0.8660254037844387076, 1.000000000000000000, 0.8660254037844387076, 1.000000000000000000, 0.8660254037844387076, 1.000000000000000000, 0.8660254037844387076, 1.000000000000000000, 0.8660254037844387076, 1.000000000000000000, 0.8660254037844387076, 1.000000000000000000, 0.8660254037844387076, 1.000000000000000000, 0.8660254037844387076, 1.000000000000000000, 0.8660254037844387076, 1.000000000000000000, 0.8660254037844387076, 1.000000000000000000, 0.8660254037844387076, 1.000000000000000000, 0.8660254037844387076, 1.000000000000000000, 0.8660254037844387076, 1.000000000000000000, 0.8660254037844387076, 1.000000000000000000, 0.8660254037844387076, 1.000000000000000000, 0.8660254037844387076, 1.000000000000000000, 0.8660254037844387076, 1.000000000000000000, 0.8660254037844387076, 1.000000000000000000, 0.8660254037844387076, 1.000000000000000000, 0.8660254037844387076, 1.000000000000000000, 0.8660254037844387076, 1.000000000000000000, 0.8660254037844387076, 1.000000000000000000, 0.8660254037844387076, 1.000000000000000000, 0.8660254037844387076, 1.000000000000000000, 0.8660254037844387076, 1.000000000000000000, 0.8660254037844387076, 1.000000000000000000, 0.8660254037844387076, 1.000000000000000000, 0.8660254037844387076, 1.000000000000000000, 0.8660254037844387076, 1.000000000000000000, 0.8660254037844387076, 1.000000000000000000, 0.8660254037844387076, 1.000000000000000000, 0.8660254037844387076, 1.000000000000000000, 0.8660254037844387076, 1.000000000000000000, 0.8660254037844387076, 1.000000000000000000, 0.8660254037844387076, 1.000000000000000000, 0.8660254037844387076, 1.000000000000000000, 0.8660254037844387076, 1.000000000000000000, 0.8660254037844387076, 1.000000000000000000, 0.8660254037844387076, 1.000000000000000000, 0.8660254037844387076, 1.000000000000000000, 0.8660254037844387076, 1.000000000000000000, 0.8660254037844387076, 1.000000000000000000, 0.8660254037844387076, 1.000000000000000000, 0.8660254037844387076, 1.000000000000000000, 0.8660254037844387076, 1.000000000000000000, 0.8660254037844387076, 1.000000000000000000, 0.8660254037844387076, 1.000000000000000000, 0.8660254037844387076, 1.000000000000000000, 0.8660254037844387076, 1.000000000000000000, 0.8660254037844387076, 1.000000000000000000, 0.8660254037844387076, 1.000000000000000000, 0.8660254037844387076, 1.000000000000000000, 0.8660254037844387076, 1.000000000000000000, 0.8660254037844387076, 1.000000000000000000, 0.8660254037844387076, 1.000000000000000000, 0.8660254037844387076, 1.000000000000000000, 0.8660254037844387076, 1.000000000000000000, 0.8660254037844387076, 1.000000000000000000, 0.8660254037844387076, 1.000000000000000000, 0.8660254037844387076, 1.000000000000000000, 0.8660254037844387076, 1.000000000000000000, 0.8660254037844387076, 1.000000000000000000, 0.8660254037844387076, 1.000000000000000000, 0.8660254037844387076, 1.000000000000000000, 0.8660254037844387076, 1.000000000000000000, 0.8660254037844387076, 1.000000000000000000, 0.8660254037844387076, 1.000000000000000000, 0.8660254037844387076, 1.000000000000000000, 0.8660254037844387076, 1.000000000000000000, 0.8660254037844387076, 1.000000000000000000, 0.8660254037844387076, 1.000000000000000000, 0.8660254037844387076, 1.000000000000000000, 0.8660254037844387076, 1.000000000000000000, 0.8660254037844387076, 1.000000000000000000, 0.8660254037844387076, 1.000000000000000000, 0.8660254037844387076, 1.000000000000000000, 0.8660254037844387076, 1.000000000000000000, 0.8660254037844387076, 1.000000000000000000, 0.8660254037844387076, 1.000000000000000000, 0.8660254037844387076, 1.000000000000000000, 0.8660254037844387076, 1.000000000000000000, 0.8660254037844387076, 1.000000000000000000, 0.8660254037844387076, 1.000000000000000000, 0.8660254037844387076, 1.000000000000000000, 0.8660254037844387076, 1.000000000000000000, 0.8660254037844387076, 1.000000000000000000, 0.8660254037844387076, 1.000000000000000000, 0.8660254037844387076, 1.000000000000000000, 0.8660254037844387076, 1.000000000000000000, 0.8660254037844387076, 1.000000000000000000, 0.8660254037844387076, 1.000000000000000000, 0.8660254037844387076, 1.000000000000000000, 0.8660254037844387076, 1.000000000000000000, 0.8660254037844387076, 1.000000000000000000, 0.8660254037844387076, 1.000000000000000000, 0.8660254037844387076, 1.000000000000000000, 0.8660254037844387076, 1.000000000000000000, 0.8660254037844387076, 1.000000000000000000, 0.8660254037844387076, 1.000000000000000000, 0.8660254037844387076, 1.000000000000000000, 0.8660254037844387076, 1.000000000000000000, 0.8660254037844387076, 1.000000000000000000, 0.8660254037844387076, 1.000000000000000000, 0.8660254037844387076, 1.000000000000000000, 0.8660254037844387076, 1.000000000000000000, 0.8660254037844387076, 1.000000000000000000, 0.8660254037844387076, 1.000000000000000000, 0.8660254037844387076, 1.000000000000000000, 0.8660254037844387076, 1.000000000000000000, 0.8660254037844387076, 1.000000000000000000, 0.8660254037844387076, 1.000000000000000000, 0.8660254037844387076, 1.000000000000000000, 0.8660254037844387076, 1.000000000000000000, 0.8660254037844387076, 1.000000000000000000, 0.8660254037844387076, 1.000000000000000000, 0.8660254037844387076, 1.000000000000000000, 0.8660254037844387076, 1.000000000000000000, 0.8660254037844387076, 1.000000000000000000, 0.8660254037844387076, 1.000000000000000000, 0.8660254037844387076, 1.000000000000000000, 0.8660254037844387076, 1.000000000000000000, 0.8660254037844387076, 1.000000000000000000, 0.8660254037844387076, 1.000000000000000000, 0.8660254037844387076, 1.000000000000000000, 0.8660254037844387076, 1.000000000000000000, 0.8660254037844387076, 1.000000000000000000, 0.8660254037844387076, 1.000000000000000000, 0.8660254037844387076, 1.000000000000000000, 0.8660254037844387076, 1.000000000000000000, 0.8660254037844387076, 1.000000000000000000, 0.8660254037844387076, 1.000000000000000000, 0.8660254037844387076, 1.000000000000000000, 0.8660254037844387076, 1.000000000000000000, 0.8660254037844387076, 1.000000000000000000, 0.8660254037844387076, 1.000000000000000000, 0.8660254037844387076, 1.000000000000000000, 0.8660254037844387076, 1.000000000000000000, 0.8660254037844387076, 1.000000000000000000, 0.8660254037844387076, 1.000000000000000000, 0.8660254037844387076, 1.000000000000000000, 0.8660254037844387076, 1.000000000000000000, 0.8660254037844387076, 1.000000000000000000, 0.8660254037844387076, 1.000000000000000000, 0.8660254037844387076, 1.000000000000000000, 0.8660254037844387076, 1.000000000000000000, 0.8660254037844387076, 1.000000000000000000, 0.8660254037844387076, 1.000000000000000000, 0.8660254037844387076, 1.000000000000000000, 0.8660254037844387076, 1.000000000000000000, 0.8660254037844387076, 1.000000000000000000, 0.8660254037844387076, 1.000000000000000000, 0.8660254037844387076, 1.000000000000000000, 0.8660254037844387076, 1.000000000000000000, 0.8660254037844387076, 1.000000000000000000, 0.8660254037844387076, 1.000000000000000000, 0.8660254037844387076, 1.000000000000000000, 0.8660254037844387076, 1.000000000000000000, 0.8660254037844387076, 1.000000000000000000, 0.8660254037844387076, 1.000000000000000000, 0.8660254037844387076, 1.000000000000000000, 0.8660254037844387076, 1.000000000000000000, 0.8660254037844387076, 1.000000000000000000, 0.8660254037844387076, 1.000000000000000000, 0.8660254037844387076, 1.000000000000000000, 0.8660254037844387076, 1.000000000000000000, 0.8660254037844387076, 1.000000000000000000, 0.8660254037844387076, 1.000000000000000000, 0.8660254037844387076, 1.000000000000000000, 0.8660254037844387076, 1.000000000000000000, 0.8660254037844387076, 1.000000000000000000, 0.8660254037844387076, 1.000000000000000000, 0.8660254037844387076, 1.000000000000000000, 0.8660254037844387076, 1.000000000000000000, 0.8660254037844387076, 1.000000000000000000, 0.8660254037844387076, 1.000000000000000000, 0.8660254037844387076, 1.000000000000000000, 0.8660254037844387076, 1.000000000000000000, 0.8660254037844387076, 1.000000000000000000, 0.8660254037844387076, 1.000000000000000000, 0.8660254037844387076, 1.000000000000000000, 0.8660254037844387076, 1.000000000000000000, 0.8660254037844387076, 1.000000000000000000, 0.8660254037844387076, 1.000000000000000000, 0.8660254037844387076, 1.000000000000000000, 0.8660254037844387076, 1.000000000000000000, 0.8660254037844387076, 1.000000000000000000, 0.8660254037844387076, 1.000000000000000000, 0.8660254037844387076, 1.000000000000000000, 0.8660254037844387076, 1.000000000000000000, 0.8660254037844387076, 1.000000000000000000, 0.8660254037844387076, 1.000000000000000000, 0.8660254037844387076, 1.000000000000000000, 0.8660254037844387076, 1.000000000000000000, 0.8660254037844387076, 1.000000000000000000, 0.8660254037844387076, 1.000000000000000000, 0.8660254037844387076, 1.000000000000000000, 0.8660254037844387076, 1.000000000000000000, 0.8660254037844387076, 1.000000000000000000, 0.8660254037844387076, 1.000000000000000000, 0.8660254037844387076, 1.000000000000000000, 0.8660254037844387076, 1.000000000000000000, 0.8660254037844387076, 1.000000000000000000, 0.8660254037844387076, 1.000000000000000000, 0.8660254037844387076, 1.000000000000000000, 0.8660254037844387076, 1.000000000000000000, 0.8660254037844387076, 1.000000000000000000, 0.8660254037844387076, 1.000000000000000000, 0.8660254037844387076, 1.000000000000000000, 0.8660254037844387076, 1.000000000000000000, 0.8660254037844387076, 1.000000000000000000, 0.8660254037844387076, 1.000000000000000000, 0.8660254037844387076, 1.000000000000000000, 0.8660254037844387076, 1.000000000000000000, 0.8660254037844387076, 1.000000000000000000, 0.8660254037844387076, 1.000000000000000000, 0.8660254037844387076, 1.000000000000000000, 0.8660254037844387076, 1.000000000000000000, 0.8660254037844387076, 1.000000000000000000, 0.8660254037844387076, 1.000000000000000000, 0.8660254037844387076, 1.000000000000000000, 0.8660254037844387076, 1.000000000000000000, 0.8660254037844387076, 1.000000000000000000, 0.8660254037844387076, 1.000000000000000000, 0.8660254037844387076, 1.000000000000000000, 0.8660254037844387076, 1.000000000000000000, 0.8660254037844387076, 1.000000000000000000, 0.8660254037844387076, 1.000000000000000000, 0.8660254037844387076, 1.000000000000000000, 0.8660254037844387076, 1.000000000000000000, 0.8660254037844387076, 1.000000000000000000, 0.8660254037844387076, 1.000000000000000000, 0.8660254037844387076, 1.000000000000000000, 0.8660254037844387076, 1.000000000000000000, 0.8660254037844387076, 1.000000000000000000, 0.8660254037844387076, 1.000000000000000000, 0.8660254037844387076, 1.000000000000000000, 0.8660254037844387076, 1.000000000000000000, 0.8660254037844387076, 1.000000000000000000, 0.8660254037844387076, 1.000000000000000000, 0.8660254037844387076, 1.000000000000000000, 0.8660254037844387076, 1.000000000000000000, 0.8660254037844387076, 1.000000000000000000, 0.8660254037844387076, 1.000000000000000000, 0.8660254037844387076, 1.000000000000000000, 0.8660254037844387076, 1.000000000000000000, 0.8660254037844387076, 1.000000000000000000, 0.8660254037844387076, 1.000000000000000000, 0.8660254037844387076, 1.000000000000000000) ) ) 
 REPRESENTATION_ITEM ( '' )  SURFACE ( )  );
#12439=CARTESIAN_POINT ( 'NONE',  ( 18.75937500061451857, 2.746126346562645981, -4.756430356249997438 ) ) ;
#12453=VECTOR ( 'NONE', #33625, 1000.000000000000000 ) ;
#12459=CARTESIAN_POINT ( 'NONE',  ( 21.12187500061451573, 2.746126346562645981, -4.756430356249997438 ) ) ;
#12480=CARTESIAN_POINT ( 'NONE',  ( 29.49375000122902790, 5.773502691896255534, 3.535250795749688894E-16 ) ) ;
#12482=CYLINDRICAL_SURFACE ( 'NONE', #67937, 4.999999999999998224 ) ;
#12493=EDGE_LOOP ( 'NONE', ( #42371, #23182, #6855, #14243 ) ) ;
#12504=CARTESIAN_POINT ( 'NONE',  ( 21.89999999999999858, 0.000000000000000000, 4.999999999999998224 ) ) ;
#12505=CARTESIAN_POINT ( 'NONE',  ( 8.446875000614518569, -2.746126346562642428, -4.756430356249999214 ) ) ;
#12514=DIRECTION ( 'NONE',  ( -1.000000000000000000, -0.000000000000000000, -0.000000000000000000 ) ) ;
#12522=CARTESIAN_POINT ( 'NONE',  ( 16.65937500061451715, 2.746126346562643317, 4.756430356249998326 ) ) ;
#12525=CARTESIAN_POINT ( 'NONE',  ( 26.93437500061451573, 5.492252693125287522, 3.363034840372157021E-16 ) ) ;
#12539=CARTESIAN_POINT ( 'NONE',  ( 26.10937500061451644, 4.119189519843966529, -2.378215178124998275 ) ) ;
#12557=CARTESIAN_POINT ( 'NONE',  ( 14.85937500061451644, 4.119189519843966529, -2.378215178124998275 ) ) ;
#12570=CARTESIAN_POINT ( 'NONE',  ( 29.26875000122903003, -5.773502691896255534, -1.060575238724906372E-15 ) ) ;
#12571=ORIENTED_EDGE ( 'NONE', *, *, #58478, .T. ) ;
#12574=CARTESIAN_POINT ( 'NONE',  ( 11.10000000000000142, 0.000000000000000000, 4.999999999999998224 ) ) ;
#12589=CARTESIAN_POINT ( 'NONE',  ( 15.79687500061451821, 5.492252693125287522, 3.363034840372157021E-16 ) ) ;
#12596=CARTESIAN_POINT ( 'NONE',  ( 17.84999999999999787, 0.000000000000000000, 4.999999999999998224 ) ) ;
#12601=CARTESIAN_POINT ( 'NONE',  ( 24.34687500061451715, 0.000000000000000000, 4.756430356249998326 ) ) ;
#12603=PLANE ( 'NONE',  #60851 ) ;
#12608=CARTESIAN_POINT ( 'NONE',  ( 25.65937500061451360, 2.746126346562643317, 4.756430356249998326 ) ) ;
#12610=CARTESIAN_POINT ( 'NONE',  ( 11.29687500061451644, 0.000000000000000000, 4.756430356249998326 ) ) ;
#12618=CARTESIAN_POINT ( 'NONE',  ( 12.46875000122903288, 2.886751345948126879, 4.999999999999998224 ) ) ;
#12619=ORIENTED_EDGE ( 'NONE', *, *, #72365, .T. ) ;
#12621=CARTESIAN_POINT ( 'NONE',  ( 12.49687500061451573, 4.119189519843966529, -2.378215178124998275 ) ) ;
#12628=DIRECTION ( 'NONE',  ( -1.000000000000000000, -0.000000000000000000, -0.000000000000000000 ) ) ;
#12640=CARTESIAN_POINT ( 'NONE',  ( 22.09687500061451715, 5.492252693125287522, 3.363034840372157021E-16 ) ) ;
#12659=CARTESIAN_POINT ( 'NONE',  ( 16.81875000122903430, 2.886751345948129099, -4.999999999999998224 ) ) ;
#12661=CARTESIAN_POINT ( 'NONE',  ( 10.25625000122903252, 0.000000000000000000, 4.999999999999998224 ) ) ;
#12675=CARTESIAN_POINT ( 'NONE',  ( 22.73437500061451644, -4.119189519843968306, 2.378215178124996054 ) ) ;
#12681=CARTESIAN_POINT ( 'NONE',  ( 25.31250000000000000, 2.886751345948129099, -4.999999999999998224 ) ) ;
#12684=CARTESIAN_POINT ( 'NONE',  ( 28.93125000122903145, 6.123233995736764310E-16, -4.999999999999998224 ) ) ;
#12690=CARTESIAN_POINT ( 'NONE',  ( 10.29375000122903216, -2.886751345948129988, 4.999999999999997335 ) ) ;
#12693=CARTESIAN_POINT ( 'NONE',  ( 18.30937500061451573, 2.746126346562645981, -4.756430356249997438 ) ) ;
#12704=CARTESIAN_POINT ( 'NONE',  ( 11.29687500061451644, 0.000000000000000000, 4.756430356249998326 ) ) ;
#12717=CARTESIAN_POINT ( 'NONE',  ( 11.73750000000000249, -2.886751345948125991, -5.000000000000000000 ) ) ;
#12725=CARTESIAN_POINT ( 'NONE',  ( 29.03437500061451715, -4.119189519843968306, 2.378215178124996054 ) ) ;
#12727=CARTESIAN_POINT ( 'NONE',  ( 28.02187500061451431, -4.119189519843968306, 2.378215178124996054 ) ) ;
#12728=CARTESIAN_POINT ( 'NONE',  ( 12.30937500061451573, 0.000000000000000000, 4.756430356249998326 ) ) ;
#12744=CARTESIAN_POINT ( 'NONE',  ( 22.74375000122903145, 5.773502691896255534, 3.535250795749688894E-16 ) ) ;
#12746=CARTESIAN_POINT ( 'NONE',  ( 22.57499999999999929, 6.123233995736764310E-16, -4.999999999999998224 ) ) ;
#12765=( BOUNDED_CURVE ( )  B_SPLINE_CURVE ( 2, ( #60075, #65997, #26849, #43839, #3953, #43102, #60808 ),
 .UNSPECIFIED., .F., .F. ) 
 B_SPLINE_CURVE_WITH_KNOTS ( ( 3, 2, 2, 3 ),
 ( 0.2200000000000000011, 0.2233333333333333282, 0.2266666666666666552, 0.2300000000000000100 ),
 .UNSPECIFIED. ) 
 CURVE ( )  GEOMETRIC_REPRESENTATION_ITEM ( )  RATIONAL_B_SPLINE_CURVE ( ( 1.000000000000000000, 0.8660254037844387076, 1.000000000000000000, 0.8660254037844387076, 1.000000000000000000, 0.8660254037844387076, 1.000000000000000000 ) ) 
 REPRESENTATION_ITEM ( '' )  );
#12770=DIRECTION ( 'NONE',  ( 0.000000000000000000, 0.000000000000000000, 1.000000000000000000 ) ) ;
#12795=CARTESIAN_POINT ( 'NONE',  ( 19.92187500061451289, -4.119189519843968306, 2.378215178124996054 ) ) ;
#12803=CARTESIAN_POINT ( 'NONE',  ( 11.41875000122903216, 2.886751345948129099, -4.999999999999997335 ) ) ;
#12813=CARTESIAN_POINT ( 'NONE',  ( 11.15625000122903288, 0.000000000000000000, 4.999999999999998224 ) ) ;
#12814=CARTESIAN_POINT ( 'NONE',  ( 19.92187500061451644, 2.746126346562643317, 4.756430356249998326 ) ) ;
#12825=CARTESIAN_POINT ( 'NONE',  ( 45.00000000000000000, 0.000000000000000000, 4.999999999999998224 ) ) ;
#12826=ORIENTED_EDGE ( 'NONE', *, *, #63077, .T. ) ;
#12828=CARTESIAN_POINT ( 'NONE',  ( 13.83749999999999858, -2.886751345948130876, 4.999999999999996447 ) ) ;
#12835=CARTESIAN_POINT ( 'NONE',  ( 8.400000000000000355, 0.000000000000000000, 4.999999999999998224 ) ) ;
#12838=CARTESIAN_POINT ( 'NONE',  ( 22.85625000122903216, 0.000000000000000000, 4.999999999999998224 ) ) ;
#12847=VERTEX_POINT ( 'NONE', #20202 ) ;
#12848=EDGE_LOOP ( 'NONE', ( #65125, #11411, #25924, #67209 ) ) ;
#12860=CARTESIAN_POINT ( 'NONE',  ( 7.996875000614519280, -2.746126346562642428, -4.756430356249999214 ) ) ;
#12862=DIRECTION ( 'NONE',  ( -1.000000000000000000, -0.000000000000000000, -0.000000000000000000 ) ) ;
#12866=CARTESIAN_POINT ( 'NONE',  ( 11.77500000000000036, 6.123233995736764310E-16, -4.999999999999998224 ) ) ;
#12879=CARTESIAN_POINT ( 'NONE',  ( 18.34687500061451360, 4.119189519843966529, -2.378215178124998275 ) ) ;
#12882=CARTESIAN_POINT ( 'NONE',  ( 25.50937500061451502, 2.746126346562645981, -4.756430356249997438 ) ) ;
#12889=CARTESIAN_POINT ( 'NONE',  ( 21.84375000122903288, 5.773502691896255534, 3.535250795749688401E-16 ) ) ;
#12897=CARTESIAN_POINT ( 'NONE',  ( 27.45937500061451786, 4.119189519843966529, -2.378215178124998275 ) ) ;
#12915=CARTESIAN_POINT ( 'NONE',  ( 11.74687500061451573, 5.492252693125287522, 3.363034840372157021E-16 ) ) ;
#12927=CARTESIAN_POINT ( 'NONE',  ( 23.53125000122902932, 6.123233995736764310E-16, -4.999999999999998224 ) ) ;
#12945=CARTESIAN_POINT ( 'NONE',  ( 15.19687500061451857, -2.746126346562642428, -4.756430356249999214 ) ) ;
#12952=CARTESIAN_POINT ( 'NONE',  ( 16.83749999999999858, 5.773502691896255534, 3.535250795749688894E-16 ) ) ;
#12956=CARTESIAN_POINT ( 'NONE',  ( 23.03437500061451360, -2.746126346562646425, 4.756430356249996549 ) ) ;
#12963=CARTESIAN_POINT ( 'NONE',  ( 25.17187500061451644, 4.119189519843966529, 2.378215178124999607 ) ) ;
#12965=CARTESIAN_POINT ( 'NONE',  ( 10.80937500061451573, 2.746126346562643317, 4.756430356249998326 ) ) ;
#12968=ORIENTED_EDGE ( 'NONE', *, *, #28075, .F. ) ;
#12970=CYLINDRICAL_SURFACE ( 'NONE', #22942, 4.999999999999998224 ) ;
#12975=CARTESIAN_POINT ( 'NONE',  ( 17.62500000000000000, 6.123233995736764310E-16, -4.999999999999998224 ) ) ;
#12978=CARTESIAN_POINT ( 'NONE',  ( 10.84687500061451715, 0.000000000000000000, 4.756430356249998326 ) ) ;
#12981=( BOUNDED_CURVE ( )  B_SPLINE_CURVE ( 2, ( #30503, #6887, #40150, #62669, #68947, #24585, #47133 ),
 .UNSPECIFIED., .F., .F. ) 
 B_SPLINE_CURVE_WITH_KNOTS ( ( 3, 2, 2, 3 ),
 ( 0.9799999999999999822, 0.9833333333333333925, 0.9866666666666668029, 0.9900000000000002132 ),
 .UNSPECIFIED. ) 
 CURVE ( )  GEOMETRIC_REPRESENTATION_ITEM ( )  RATIONAL_B_SPLINE_CURVE ( ( 1.000000000000000000, 0.8660254037844387076, 1.000000000000000000, 0.8660254037844387076, 1.000000000000000000, 0.8660254037844298258, 1.000000000000008882 ) ) 
 REPRESENTATION_ITEM ( '' )  );
#12997=CARTESIAN_POINT ( 'NONE',  ( 22.58437500061451431, 4.119189519843966529, 2.378215178124999607 ) ) ;
#13017=CARTESIAN_POINT ( 'NONE',  ( 9.412499999999999645, -5.773502691896255534, -1.060575238724906372E-15 ) ) ;
#13031=CARTESIAN_POINT ( 'NONE',  ( 22.69687500061451857, -2.746126346562646425, 4.756430356249996549 ) ) ;
#13038=CARTESIAN_POINT ( 'NONE',  ( 24.52499999999999858, 4.330127018922191873, 2.499999999999999556 ) ) ;
#13045=CARTESIAN_POINT ( 'NONE',  ( 15.18750000000000000, -2.886751345948130876, 4.999999999999996447 ) ) ;
#13047=CARTESIAN_POINT ( 'NONE',  ( 9.918750001229033941, -5.773502691896255534, -1.060575238724906372E-15 ) ) ;
#13050=CARTESIAN_POINT ( 'NONE',  ( 18.79687500061451289, 4.119189519843966529, -2.378215178124998275 ) ) ;
#13061=CARTESIAN_POINT ( 'NONE',  ( 9.384375000614516793, 5.492252693125287522, 3.363034840372157021E-16 ) ) ;
#13070=CARTESIAN_POINT ( 'NONE',  ( 9.056250001229033231, -4.330127018922190985, -2.500000000000001332 ) ) ;
#13072=CARTESIAN_POINT ( 'NONE',  ( 29.33437500061451431, -2.746126346562646425, 4.756430356249996549 ) ) ;
#13075=CARTESIAN_POINT ( 'NONE',  ( 11.62500000000000000, -4.330127018922194537, 2.499999999999995559 ) ) ;
#13081=ADVANCED_FACE ( 'NONE', ( #32769 ), #27230, .T. ) ;
#13084=CARTESIAN_POINT ( 'NONE',  ( 28.32187500061451502, 2.746126346562645981, -4.756430356249997438 ) ) ;
#13086=CARTESIAN_POINT ( 'NONE',  ( 27.19687500061451502, -4.119189519843965641, -2.378215178125001383 ) ) ;
#13087=CARTESIAN_POINT ( 'NONE',  ( 11.59687500061451892, -2.746126346562642428, -4.756430356249999214 ) ) ;
#13102=CARTESIAN_POINT ( 'NONE',  ( 23.53125000122902932, 6.123233995736764310E-16, -4.999999999999998224 ) ) ;
#13110=CARTESIAN_POINT ( 'NONE',  ( 7.781250001229034652, 6.123233995736764310E-16, -4.999999999999998224 ) ) ;
#13126=DIRECTION ( 'NONE',  ( -1.000000000000000000, -0.000000000000000000, -0.000000000000000000 ) ) ;
#13130=FACE_OUTER_BOUND ( 'NONE', #12493, .T. ) ;
#13134=CARTESIAN_POINT ( 'NONE',  ( 19.06875000122903074, 2.886751345948045611, -5.000000000000141220 ) ) ;
#13151=CARTESIAN_POINT ( 'NONE',  ( 17.03437500061451715, 5.492252693125287522, 3.363034840372157021E-16 ) ) ;
#13168=DIRECTION ( 'NONE',  ( -1.000000000000000000, -0.000000000000000000, -0.000000000000000000 ) ) ;
#13171=CARTESIAN_POINT ( 'NONE',  ( 19.20937500061451786, -4.119189519843965641, -2.378215178125001383 ) ) ;
#13175=ADVANCED_FACE ( 'NONE', ( #60096 ), #9607, .T. ) ;
#13184=ORIENTED_EDGE ( 'NONE', *, *, #8691, .F. ) ;
#13203=EDGE_LOOP ( 'NONE', ( #47782, #7859, #70996, #57241 ) ) ;
#13217=CARTESIAN_POINT ( 'NONE',  ( 29.43750000000000000, 5.773502691896255534, 3.535250795749688894E-16 ) ) ;
#13224=VECTOR ( 'NONE', #28227, 1000.000000000000000 ) ;
#13235=CARTESIAN_POINT ( 'NONE',  ( 15.72187500061451537, 4.119189519843966529, 2.378215178124999607 ) ) ;
#13238=CARTESIAN_POINT ( 'NONE',  ( 25.05937500061451573, 2.746126346562645981, -4.756430356249997438 ) ) ;
#13252=CARTESIAN_POINT ( 'NONE',  ( 26.52187500061451431, 2.746126346562645981, -4.756430356249997438 ) ) ;
#13255=LINE ( 'NONE', #52433, #24277 ) ;
#13262=ORIENTED_EDGE ( 'NONE', *, *, #17788, .T. ) ;
#13271=CARTESIAN_POINT ( 'NONE',  ( 11.48437500061451644, -4.119189519843968306, 2.378215178124996054 ) ) ;
#13296=ORIENTED_EDGE ( 'NONE', *, *, #66954, .T. ) ;
#13301=CARTESIAN_POINT ( 'NONE',  ( 16.47187500061452070, -5.492252693125287522, -1.008910452111647106E-15 ) ) ;
#13307=CARTESIAN_POINT ( 'NONE',  ( 17.58749999999999858, -2.886751345948125991, -5.000000000000000000 ) ) ;
#13311=CARTESIAN_POINT ( 'NONE',  ( 23.07187500061451502, -4.119189519843968306, 2.378215178124996054 ) ) ;
#13312=ORIENTED_EDGE ( 'NONE', *, *, #50852, .F. ) ;
#13319=CARTESIAN_POINT ( 'NONE',  ( 23.44687500061451502, 0.000000000000000000, 4.756430356249998326 ) ) ;
#13321=CARTESIAN_POINT ( 'NONE',  ( 9.909375000614517148, 2.746126346562643317, 4.756430356249998326 ) ) ;
#13324=ORIENTED_EDGE ( 'NONE', *, *, #43284, .T. ) ;
#13333=CARTESIAN_POINT ( 'NONE',  ( 12.00937500061451502, 2.746126346562645981, -4.756430356249997438 ) ) ;
#13339=ADVANCED_FACE ( 'NONE', ( #32278 ), #54451, .T. ) ;
#13351=CARTESIAN_POINT ( 'NONE',  ( 18.60937500061451644, 0.000000000000000000, 4.756430356249998326 ) ) ;
#13384=CARTESIAN_POINT ( 'NONE',  ( 23.82187500061451502, 2.746126346562645981, -4.756430356249997438 ) ) ;
#13390=CARTESIAN_POINT ( 'NONE',  ( 23.62500000000000000, 4.330127018922191873, 2.499999999999999556 ) ) ;
#13398=CARTESIAN_POINT ( 'NONE',  ( 10.55625000122903323, 4.330127018922192761, -2.499999999999997780 ) ) ;
#13401=CARTESIAN_POINT ( 'NONE',  ( 17.10937500061451644, 2.746126346562643317, 4.756430356249998326 ) ) ;
#13413=CARTESIAN_POINT ( 'NONE',  ( 10.92187500061451644, -4.119189519843968306, 2.378215178124996054 ) ) ;
#13419=ORIENTED_EDGE ( 'NONE', *, *, #36009, .T. ) ;
#13424=CARTESIAN_POINT ( 'NONE',  ( 28.88437500061451502, -2.746126346562646425, 4.756430356249996549 ) ) ;
#13428=CARTESIAN_POINT ( 'NONE',  ( 8.737500000000002487, 5.773502691896255534, 3.535250795749688894E-16 ) ) ;
#13436=CARTESIAN_POINT ( 'NONE',  ( 27.57187500061451857, 2.746126346562643317, 4.756430356249998326 ) ) ;
#13438=CARTESIAN_POINT ( 'NONE',  ( 28.13437500061451502, -2.746126346562641984, -4.756430356249999214 ) ) ;
#13439=CARTESIAN_POINT ( 'NONE',  ( 11.14687500061451608, -2.746126346562642428, -4.756430356249999214 ) ) ;
#13455=CARTESIAN_POINT ( 'NONE',  ( 21.54375000122902861, -2.886751345948129988, 4.999999999999997335 ) ) ;
#13474=EDGE_CURVE ( 'NONE', #69337, #50344, #55362, .T. ) ;
#13481=CARTESIAN_POINT ( 'NONE',  ( -2.928932188134523606, 4.999999999999997335, -2.928932188134523606 ) ) ;
#13512=CARTESIAN_POINT ( 'NONE',  ( 17.48437500061451644, 5.492252693125287522, 3.363034840372157021E-16 ) ) ;
#13521=ORIENTED_EDGE ( 'NONE', *, *, #34883, .F. ) ;
#13529=CARTESIAN_POINT ( 'NONE',  ( 8.418750001229032165, 2.886751345948238789, 4.999999999999807265 ) ) ;
#13532=CARTESIAN_POINT ( 'NONE',  ( 16.84687500061451715, -2.746126346562646425, 4.756430356249996549 ) ) ;
#13550=CARTESIAN_POINT ( 'NONE',  ( 27.39375000122903359, -2.886751345948129988, 4.999999999999997335 ) ) ;
#13566=VECTOR ( 'NONE', #55641, 1000.000000000000000 ) ;
#13578=CARTESIAN_POINT ( 'NONE',  ( 29.92500000000000071, 4.330127018922191873, 2.499999999999999556 ) ) ;
#13584=CARTESIAN_POINT ( 'NONE',  ( 27.48750000000000071, -2.886751345948091796, -5.000000000000060396 ) ) ;
#13598=CARTESIAN_POINT ( 'NONE',  ( 14.18437500061451573, -2.746126346562642428, -4.756430356249999214 ) ) ;
#13601=CARTESIAN_POINT ( 'NONE',  ( 23.44687500061451502, 0.000000000000000000, 4.756430356249998326 ) ) ;
#13617=CARTESIAN_POINT ( 'NONE',  ( 25.99687500061451928, -2.746126346562642428, -4.756430356249999214 ) ) ;
#13638=CARTESIAN_POINT ( 'NONE',  ( 12.42187500061451821, -5.492252693125287522, -1.008910452111647106E-15 ) ) ;
#13649=STYLED_ITEM('',(#73144),#45331);
#13669=CARTESIAN_POINT ( 'NONE',  ( 14.25937500061451679, -4.119189519843965641, -2.378215178125001383 ) ) ;
#13676=CARTESIAN_POINT ( 'NONE',  ( 15.78749999999999964, -2.886751345948125991, -5.000000000000000000 ) ) ;
#13680=CARTESIAN_POINT ( 'NONE',  ( 22.13437500061451146, -2.746126346562646425, 4.756430356249996549 ) ) ;
#13690=CARTESIAN_POINT ( 'NONE',  ( 21.83437500061451786, -2.746126346562642428, -4.756430356249999214 ) ) ;
#13692=CARTESIAN_POINT ( 'NONE',  ( 8.071875000614515017, 4.119189519843966529, 2.378215178124999607 ) ) ;
#13702=ORIENTED_EDGE ( 'NONE', *, *, #1440, .T. ) ;
#13704=CARTESIAN_POINT ( 'NONE',  ( 12.87187500061451750, 5.824947211148865298E-16, -4.756430356249998326 ) ) ;
#13712=CARTESIAN_POINT ( 'NONE',  ( 23.62500000000000000, 4.330127018922191873, 2.499999999999999556 ) ) ;
#13728=CARTESIAN_POINT ( 'NONE',  ( 20.03437500061451715, -4.119189519843968306, 2.378215178124996054 ) ) ;
#13742=ORIENTED_EDGE ( 'NONE', *, *, #55050, .T. ) ;
#13754=DIRECTION ( 'NONE',  ( 0.000000000000000000, 0.000000000000000000, 1.000000000000000000 ) ) ;
#13762=CARTESIAN_POINT ( 'NONE',  ( 20.25937500061451857, 4.119189519843966529, -2.378215178124998275 ) ) ;
#13768=CARTESIAN_POINT ( 'NONE',  ( 23.55000000000000071, 4.330127018922192761, -2.499999999999997780 ) ) ;
#13773=CARTESIAN_POINT ( 'NONE',  ( 45.00000000000000000, 0.000000000000000000, 0.000000000000000000 ) ) ;
#13774=CARTESIAN_POINT ( 'NONE',  ( 45.00000000000000000, 0.000000000000000000, 0.000000000000000000 ) ) ;
#13778=CARTESIAN_POINT ( 'NONE',  ( 28.84687500061451360, 0.000000000000000000, 4.756430356249998326 ) ) ;
#13780=CARTESIAN_POINT ( 'NONE',  ( 16.39687500061451431, -4.119189519843965641, -2.378215178125001383 ) ) ;
#13795=CARTESIAN_POINT ( 'NONE',  ( 9.009375000614516793, 2.746126346562643317, 4.756430356249998326 ) ) ;
#13806=CARTESIAN_POINT ( 'NONE',  ( 28.62187500061451217, 5.824947211148865298E-16, -4.756430356249998326 ) ) ;
#13809=CARTESIAN_POINT ( 'NONE',  ( 7.950000000000001954, 0.000000000000000000, 4.999999999999998224 ) ) ;
#13816=CARTESIAN_POINT ( 'NONE',  ( 26.25937500061451857, 0.000000000000000000, 4.756430356249998326 ) ) ;
#13818=CARTESIAN_POINT ( 'NONE',  ( 10.13437500061451679, -4.119189519843968306, 2.378215178124996054 ) ) ;
#13829=( NAMED_UNIT ( * ) SI_UNIT ( $, .STERADIAN. ) SOLID_ANGLE_UNIT ( ) );
#13834=CARTESIAN_POINT ( 'NONE',  ( 21.43125000122903145, 4.330127018922191873, 2.499999999999999556 ) ) ;
#13837=EDGE_LOOP ( 'NONE', ( #45915, #33207, #62238, #30436, #23367 ) ) ;
#13842=CARTESIAN_POINT ( 'NONE',  ( 7.818750001229033408, 2.886751345948129099, -4.999999999999997335 ) ) ;
#13858=CARTESIAN_POINT ( 'NONE',  ( 19.03125000122902932, 6.123233995736764310E-16, -4.999999999999998224 ) ) ;
#13859=EDGE_CURVE ( 'NONE', #72906, #25370, #17141, .T. ) ;
#13876=CARTESIAN_POINT ( 'NONE',  ( 45.00000000000000000, 6.123233995736764310E-16, -4.999999999999998224 ) ) ;
#13884=CARTESIAN_POINT ( 'NONE',  ( 25.80000000000000071, 4.330127018922192761, -2.499999999999997780 ) ) ;
#13887=CARTESIAN_POINT ( 'NONE',  ( 15.72187500061451537, 4.119189519843966529, 2.378215178124999607 ) ) ;
#13905=CARTESIAN_POINT ( 'NONE',  ( 8.231250001229033941, 6.123233995736764310E-16, -4.999999999999998224 ) ) ;
#13908=CARTESIAN_POINT ( 'NONE',  ( 17.33437500061451431, -4.119189519843968306, 2.378215178124996054 ) ) ;
#13920=ORIENTED_EDGE ( 'NONE', *, *, #21683, .T. ) ;
#13926=CARTESIAN_POINT ( 'NONE',  ( 29.19375000122903074, -2.886751345948129988, 4.999999999999997335 ) ) ;
#13930=DIRECTION ( 'NONE',  ( 0.000000000000000000, 0.000000000000000000, 1.000000000000000000 ) ) ;
#13949=CARTESIAN_POINT ( 'NONE',  ( 7.359375000614516438, 0.000000000000000000, 4.756430356249998326 ) ) ;
#13950=CARTESIAN_POINT ( 'NONE',  ( 29.55000000000000071, 0.000000000000000000, 4.999999999999998224 ) ) ;
#13968=CARTESIAN_POINT ( 'NONE',  ( 15.90937500061451360, -5.492252693125287522, -1.008910452111647106E-15 ) ) ;
#13971=CARTESIAN_POINT ( 'NONE',  ( 22.99687500061451573, 0.000000000000000000, 4.756430356249998326 ) ) ;
#13975=DIRECTION ( 'NONE',  ( -1.000000000000000000, -0.000000000000000000, -0.000000000000000000 ) ) ;
#13979=CARTESIAN_POINT ( 'NONE',  ( 11.77500000000000036, 6.123233995736764310E-16, -4.999999999999998224 ) ) ;
#13986=CARTESIAN_POINT ( 'NONE',  ( 23.85937500061451644, 4.119189519843966529, -2.378215178124998275 ) ) ;
#13989=DIRECTION ( 'NONE',  ( -1.000000000000000000, -0.000000000000000000, -0.000000000000000000 ) ) ;
#13996=CARTESIAN_POINT ( 'NONE',  ( 25.25625000122903074, -4.330127018922190985, -2.500000000000001332 ) ) ;
#14007=CARTESIAN_POINT ( 'NONE',  ( 12.68437500061451573, 4.119189519843966529, 2.378215178124999607 ) ) ;
#14023=CARTESIAN_POINT ( 'NONE',  ( 16.05000000000000071, 0.000000000000000000, 4.999999999999998224 ) ) ;
#14031=ORIENTED_EDGE ( 'NONE', *, *, #71606, .F. ) ;
#14034=CARTESIAN_POINT ( 'NONE',  ( 14.14687500061451786, -2.746126346562646425, 4.756430356249996549 ) ) ;
#14038=EDGE_CURVE ( 'NONE', #40656, #17484, #4410, .T. ) ;
#14042=CARTESIAN_POINT ( 'NONE',  ( 15.97499999999999964, 4.330127018922191873, 2.499999999999999556 ) ) ;
#14045=CARTESIAN_POINT ( 'NONE',  ( 24.75000000000000000, -4.330127018922190985, -2.500000000000001332 ) ) ;
#14046=CARTESIAN_POINT ( 'NONE',  ( 23.44687500061451502, 0.000000000000000000, 4.756430356249998326 ) ) ;
#14047=CARTESIAN_POINT ( 'NONE',  ( 26.21250000000000213, 2.886751345948157077, -4.999999999999949374 ) ) ;
#14055=CARTESIAN_POINT ( 'NONE',  ( 21.30937500061451217, -5.492252693125287522, -1.008910452111647106E-15 ) ) ;
#14057=CARTESIAN_POINT ( 'NONE',  ( 9.796875000614514661, 4.119189519843966529, -2.378215178124998275 ) ) ;
#14066=EDGE_LOOP ( 'NONE', ( #71595, #38453, #53600, #54566 ) ) ;
#14068=CARTESIAN_POINT ( 'NONE',  ( 8.259375000614515017, -5.492252693125287522, -1.008910452111647106E-15 ) ) ;
#14089=CARTESIAN_POINT ( 'NONE',  ( 19.20937500061451786, -4.119189519843965641, -2.378215178125001383 ) ) ;
#14102=ORIENTED_EDGE ( 'NONE', *, *, #36894, .F. ) ;
#14109=CARTESIAN_POINT ( 'NONE',  ( 20.60625000122902861, 0.000000000000000000, 4.999999999999998224 ) ) ;
#14116=CARTESIAN_POINT ( 'NONE',  ( -5.000000000000004441, 0.000000000000000000, 4.999999999999998224 ) ) ;
#14125=CARTESIAN_POINT ( 'NONE',  ( 21.08437500061451786, 5.824947211148865298E-16, -4.756430356249998326 ) ) ;
#14133=CARTESIAN_POINT ( 'NONE',  ( 22.12500000000000000, 6.123233995736764310E-16, -4.999999999999998224 ) ) ;
#14139=DIRECTION ( 'NONE',  ( 0.000000000000000000, 0.000000000000000000, 1.000000000000000000 ) ) ;
#14144=CARTESIAN_POINT ( 'NONE',  ( 28.99687500061451217, -4.119189519843965641, -2.378215178125001383 ) ) ;
#14146=CARTESIAN_POINT ( 'NONE',  ( 16.32187500061451502, -4.119189519843968306, 2.378215178124996054 ) ) ;
#14157=CARTESIAN_POINT ( 'NONE',  ( 7.659375000614514484, 2.746126346562643317, 4.756430356249998326 ) ) ;
#14158=VERTEX_POINT ( 'NONE', #22108 ) ;
#14168=CARTESIAN_POINT ( 'NONE',  ( 28.92187500061451644, -4.119189519843968306, 2.378215178124996054 ) ) ;
#14169=ORIENTED_EDGE ( 'NONE', *, *, #1145, .F. ) ;
#14172=CARTESIAN_POINT ( 'NONE',  ( 7.724999999999999645, 6.123233995736764310E-16, -4.999999999999998224 ) ) ;
#14179=CARTESIAN_POINT ( 'NONE',  ( 27.68437500061451573, -4.119189519843968306, 2.378215178124996054 ) ) ;
#14181=CARTESIAN_POINT ( 'NONE',  ( 11.18437500061451928, 5.824947211148865298E-16, -4.756430356249998326 ) ) ;
#14189=LINE ( 'NONE', #3118, #61961 ) ;
#14198=CARTESIAN_POINT ( 'NONE',  ( 20.30625000122903145, -4.330127018922190985, -2.500000000000001332 ) ) ;
#14206=CARTESIAN_POINT ( 'NONE',  ( 13.57500000000000107, 6.123233995736764310E-16, -4.999999999999998224 ) ) ;
#14214=CARTESIAN_POINT ( 'NONE',  ( 28.39687500061452141, 5.492252693125287522, 3.363034840372157021E-16 ) ) ;
#14239=LINE ( 'NONE', #64851, #7703 ) ;
#14243=ORIENTED_EDGE ( 'NONE', *, *, #25676, .F. ) ;
#14247=FACE_OUTER_BOUND ( 'NONE', #20157, .T. ) ;
#14250=CARTESIAN_POINT ( 'NONE',  ( 17.29687500061451644, -4.119189519843965641, -2.378215178125001383 ) ) ;
#14266=DIRECTION ( 'NONE',  ( -1.000000000000000000, -0.000000000000000000, -0.000000000000000000 ) ) ;
#14269=CARTESIAN_POINT ( 'NONE',  ( 26.94375000122903430, -2.886751345948088243, 5.000000000000068390 ) ) ;
#14270=CARTESIAN_POINT ( 'NONE',  ( 17.44687500061451857, -2.746126346562642428, -4.756430356249999214 ) ) ;
#14279=EDGE_CURVE ( 'NONE', #31892, #68516, #60087, .T. ) ;
#14286=LINE ( 'NONE', #2843, #35536 ) ;
#14290=CARTESIAN_POINT ( 'NONE',  ( 28.10625000122902861, 4.330127018922192761, -2.499999999999997780 ) ) ;
#14292=CARTESIAN_POINT ( 'NONE',  ( 26.86875000122903145, 2.886751345948168623, 4.999999999999926281 ) ) ;
#14294=CARTESIAN_POINT ( 'NONE',  ( -2.928932188134524939, 4.999999999999996447, 2.928932188134524939 ) ) ;
#14306=EDGE_CURVE ( 'NONE', #32563, #34347, #61994, .T. ) ;
#14315=CARTESIAN_POINT ( 'NONE',  ( 28.80000000000000071, -4.330127018922190985, -2.500000000000001332 ) ) ;
#14319=EDGE_CURVE ( 'NONE', #60669, #64001, #56457, .T. ) ;
#14322=CARTESIAN_POINT ( 'NONE',  ( 27.44999999999999929, -4.330127018922190985, -2.500000000000001332 ) ) ;
#14325=CARTESIAN_POINT ( 'NONE',  ( 9.206250001229033586, 4.330127018922192761, -2.499999999999997780 ) ) ;
#14336=CARTESIAN_POINT ( 'NONE',  ( 15.08437500061451431, -2.746126346562642428, -4.756430356249999214 ) ) ;
#14339=CARTESIAN_POINT ( 'NONE',  ( 23.59687500061451360, -4.119189519843965641, -2.378215178125001383 ) ) ;
#14344=CARTESIAN_POINT ( 'NONE',  ( 15.37500000000000000, 6.123233995736764310E-16, -4.999999999999998224 ) ) ;
#14349=CARTESIAN_POINT ( 'NONE',  ( 11.84999999999999964, 4.330127018922192761, -2.499999999999997780 ) ) ;
#14356=CARTESIAN_POINT ( 'NONE',  ( 25.58437500061451431, 5.824947211148865298E-16, -4.756430356249998326 ) ) ;
#14366=LINE ( 'NONE', #59421, #36018 ) ;
#14376=CARTESIAN_POINT ( 'NONE',  ( 11.78437500061451892, 4.119189519843966529, 2.378215178124999607 ) ) ;
#14399=ORIENTED_EDGE ( 'NONE', *, *, #23115, .F. ) ;
#14403=CARTESIAN_POINT ( 'NONE',  ( 13.13437500061451857, 4.119189519843966529, 2.378215178124999607 ) ) ;
#14411=CARTESIAN_POINT ( 'NONE',  ( 14.55000000000000071, 4.330127018922192761, -2.499999999999997780 ) ) ;
#14413=DIRECTION ( 'NONE',  ( 0.000000000000000000, 0.000000000000000000, 1.000000000000000000 ) ) ;
#14419=DIRECTION ( 'NONE',  ( 0.000000000000000000, 0.000000000000000000, 1.000000000000000000 ) ) ;
#14424=CARTESIAN_POINT ( 'NONE',  ( 23.59687500061451360, -4.119189519843965641, -2.378215178125001383 ) ) ;
#14426=CARTESIAN_POINT ( 'NONE',  ( 8.259375000614515017, -5.492252693125287522, -1.008910452111647106E-15 ) ) ;
#14435=CARTESIAN_POINT ( 'NONE',  ( 10.05000000000000071, 4.330127018922192761, -2.499999999999997780 ) ) ;
#14437=CARTESIAN_POINT ( 'NONE',  ( 9.009375000614516793, 2.746126346562643317, 4.756430356249998326 ) ) ;
#14448=ORIENTED_EDGE ( 'NONE', *, *, #23321, .T. ) ;
#14457=CARTESIAN_POINT ( 'NONE',  ( 22.83750000000000213, -2.886751345948157965, 4.999999999999948486 ) ) ;
#14461=CARTESIAN_POINT ( 'NONE',  ( 20.44687500061451857, -2.746126346562646425, 4.756430356249996549 ) ) ;
#14492=CARTESIAN_POINT ( 'NONE',  ( 20.29687500061451644, 5.492252693125287522, 3.363034840372157021E-16 ) ) ;
#14496=( BOUNDED_CURVE ( )  B_SPLINE_CURVE ( 2, ( #37269, #59791, #53160, #36535, #26187, #25826, #42814 ),
 .UNSPECIFIED., .F., .F. ) 
 B_SPLINE_CURVE_WITH_KNOTS ( ( 3, 2, 2, 3 ),
 ( 0.9900000000000002132, 0.9933333333333334014, 0.9966666666666668117, 1.000000000000000000 ),
 .UNSPECIFIED. ) 
 CURVE ( )  GEOMETRIC_REPRESENTATION_ITEM ( )  RATIONAL_B_SPLINE_CURVE ( ( 0.9999999999999911182, 0.8660254037844475894, 1.000000000000000000, 0.8660254037844387076, 1.000000000000000000, 0.8660254037844387076, 1.000000000000000000 ) ) 
 REPRESENTATION_ITEM ( '' )  );
#14499=CARTESIAN_POINT ( 'NONE',  ( 23.09999999999999787, 4.330127018922192761, -2.499999999999997780 ) ) ;
#14504=CARTESIAN_POINT ( 'NONE',  ( 11.86875000122902790, 2.886751345948073588, -5.000000000000094147 ) ) ;
#14507=EDGE_CURVE ( 'NONE', #30573, #42983, #34271, .T. ) ;
#14510=CARTESIAN_POINT ( 'NONE',  ( 7.931250001229031454, 4.330127018922191873, 2.499999999999999556 ) ) ;
#14512=CARTESIAN_POINT ( 'NONE',  ( 15.94687500061451502, -4.119189519843965641, -2.378215178125001383 ) ) ;
#14515=ORIENTED_EDGE ( 'NONE', *, *, #3480, .F. ) ;
#14521=CARTESIAN_POINT ( 'NONE',  ( 16.63125000122903074, -4.330127018922194537, 2.499999999999995559 ) ) ;
#14522=CARTESIAN_POINT ( 'NONE',  ( 8.821875000614515017, 5.824947211148865298E-16, -4.756430356249998326 ) ) ;
#14533=CARTESIAN_POINT ( 'NONE',  ( 27.87187500061451217, 4.119189519843966529, 2.378215178124999607 ) ) ;
#14543=CARTESIAN_POINT ( 'NONE',  ( 27.04687500061450933, 5.492252693125287522, 3.363034840372157021E-16 ) ) ;
#14545=CARTESIAN_POINT ( 'NONE',  ( 9.646875000614516082, -2.746126346562646425, 4.756430356249996549 ) ) ;
#14554=EDGE_CURVE ( 'NONE', #67801, #3601, #34638, .T. ) ;
#14564=CARTESIAN_POINT ( 'NONE',  ( 19.89375000122903359, -2.886751345948125991, -5.000000000000000000 ) ) ;
#14567=ORIENTED_EDGE ( 'NONE', *, *, #43413, .F. ) ;
#14579=CARTESIAN_POINT ( 'NONE',  ( 27.68437500061451573, -4.119189519843968306, 2.378215178124996054 ) ) ;
#14594=CARTESIAN_POINT ( 'NONE',  ( 23.25000000000000000, 0.000000000000000000, 4.999999999999998224 ) ) ;
#14603=CARTESIAN_POINT ( 'NONE',  ( 25.50000000000000000, 0.000000000000000000, 4.999999999999998224 ) ) ;
#14610=ORIENTED_EDGE ( 'NONE', *, *, #30034, .F. ) ;
#14614=CARTESIAN_POINT ( 'NONE',  ( 16.02187500061451431, 5.824947211148865298E-16, -4.756430356249998326 ) ) ;
#14628=LINE ( 'NONE', #37168, #38368 ) ;
#14632=CARTESIAN_POINT ( 'NONE',  ( 18.30937500061451928, -4.119189519843965641, -2.378215178125001383 ) ) ;
#14641=EDGE_CURVE ( 'NONE', #48464, #15624, #49758, .T. ) ;
#14643=FACE_OUTER_BOUND ( 'NONE', #60250, .T. ) ;
#14646=CARTESIAN_POINT ( 'NONE',  ( 21.69375000122902719, -2.886751345948181946, -4.999999999999904077 ) ) ;
#14650=CARTESIAN_POINT ( 'NONE',  ( 27.95625000122903359, -4.330127018922190985, -2.500000000000001332 ) ) ;
#14661=ORIENTED_EDGE ( 'NONE', *, *, #73043, .F. ) ;
#14663=CARTESIAN_POINT ( 'NONE',  ( 45.00000000000000000, 0.000000000000000000, 0.000000000000000000 ) ) ;
#14665=DIRECTION ( 'NONE',  ( 0.000000000000000000, 0.000000000000000000, -1.000000000000000000 ) ) ;
#14674=CARTESIAN_POINT ( 'NONE',  ( 29.32499999999999929, 6.123233995736764310E-16, -4.999999999999998224 ) ) ;
#14683=CARTESIAN_POINT ( 'NONE',  ( 9.318750001229034297, 2.886751345948126879, 4.999999999999998224 ) ) ;
#14684=EDGE_CURVE ( 'NONE', #24462, #36109, #11754, .T. ) ;
#14694=CARTESIAN_POINT ( 'NONE',  ( 15.23437500061451644, 5.492252693125287522, 3.363034840372157021E-16 ) ) ;
#14695=VERTEX_POINT ( 'NONE', #30195 ) ;
#14698=CARTESIAN_POINT ( 'NONE',  ( 23.25937500061451502, 2.746126346562645981, -4.756430356249997438 ) ) ;
#14709=CARTESIAN_POINT ( 'NONE',  ( 13.50000000000000178, -4.330127018922190985, -2.500000000000001332 ) ) ;
#14717=CARTESIAN_POINT ( 'NONE',  ( 24.45937500061451786, 0.000000000000000000, 4.756430356249998326 ) ) ;
#14727=CARTESIAN_POINT ( 'NONE',  ( 25.29375000122902861, -2.886751345948167735, -4.999999999999927169 ) ) ;
#14738=CARTESIAN_POINT ( 'NONE',  ( 9.796875000614518214, -2.746126346562641984, -4.756430356249999214 ) ) ;
#14751=ORIENTED_EDGE ( 'NONE', *, *, #37851, .F. ) ;
#14761=EDGE_LOOP ( 'NONE', ( #54032, #64419, #61101, #22985 ) ) ;
#14765=CARTESIAN_POINT ( 'NONE',  ( 12.79687500061451821, -2.746126346562646425, 4.756430356249996549 ) ) ;
#14770=( BOUNDED_CURVE ( )  B_SPLINE_CURVE ( 2, ( #35868, #12618, #68783, #6355, #52508, #68061, #1550 ),
 .UNSPECIFIED., .F., .F. ) 
 B_SPLINE_CURVE_WITH_KNOTS ( ( 3, 2, 2, 3 ),
 ( 0.7600000000000000089, 0.7633333333333333082, 0.7666666666666668295, 0.7700000000000001288 ),
 .UNSPECIFIED. ) 
 CURVE ( )  GEOMETRIC_REPRESENTATION_ITEM ( )  RATIONAL_B_SPLINE_CURVE ( ( 1.000000000000000000, 0.8660254037844387076, 1.000000000000000000, 0.8660254037844387076, 1.000000000000000000, 0.8660254037844342667, 1.000000000000004441 ) ) 
 REPRESENTATION_ITEM ( '' )  );
#14771=AXIS2_PLACEMENT_3D ( 'NONE', #1105, #44361, #16614 ) ;
#14775=CARTESIAN_POINT ( 'NONE',  ( 15.63749999999999751, -2.886751345948129988, 4.999999999999997335 ) ) ;
#14777=CARTESIAN_POINT ( 'NONE',  ( 16.76249999999999929, 2.886751345948129099, -4.999999999999997335 ) ) ;
#14789=CARTESIAN_POINT ( 'NONE',  ( 23.63437500061451502, -2.746126346562642428, -4.756430356249999214 ) ) ;
#14791=CARTESIAN_POINT ( 'NONE',  ( 8.784375000614515372, -2.746126346562641984, -4.756430356249999214 ) ) ;
#14801=CARTESIAN_POINT ( 'NONE',  ( 9.759375000614516793, 2.746126346562645981, -4.756430356249997438 ) ) ;
#14823=ADVANCED_FACE ( 'NONE', ( #47188 ), #12410, .T. ) ;
#14825=CARTESIAN_POINT ( 'NONE',  ( 20.59687500061451715, -2.746126346562641984, -4.756430356249999214 ) ) ;
#14838=VECTOR ( 'NONE', #42080, 1000.000000000000000 ) ;
#14855=ORIENTED_EDGE ( 'NONE', *, *, #17032, .F. ) ;
#14859=CARTESIAN_POINT ( 'NONE',  ( 20.89687500061452141, -2.746126346562646425, 4.756430356249996549 ) ) ;
#14865=CARTESIAN_POINT ( 'NONE',  ( 21.22500000000000142, 6.123233995736764310E-16, -4.999999999999998224 ) ) ;
#14877=CARTESIAN_POINT ( 'NONE',  ( 7.443750001229033408, 5.773502691896255534, 3.535250795749688894E-16 ) ) ;
#14879=CARTESIAN_POINT ( 'NONE',  ( 16.84687500061451715, -4.119189519843965641, -2.378215178125001383 ) ) ;
#14885=CARTESIAN_POINT ( 'NONE',  ( 25.94999999999999929, 0.000000000000000000, 4.999999999999998224 ) ) ;
#14888=LINE ( 'NONE', #64766, #32510 ) ;
#14895=DIRECTION ( 'NONE',  ( -1.000000000000000000, -0.000000000000000000, -0.000000000000000000 ) ) ;
#14900=CARTESIAN_POINT ( 'NONE',  ( 16.29375000122903216, -2.886751345948126435, -5.000000000000000000 ) ) ;
#14911=CARTESIAN_POINT ( 'NONE',  ( 25.95937500061451431, -4.119189519843965641, -2.378215178125001383 ) ) ;
#14913=CARTESIAN_POINT ( 'NONE',  ( 8.296875000614516438, -2.746126346562646425, 4.756430356249996549 ) ) ;
#14931=CARTESIAN_POINT ( 'NONE',  ( 21.13125000122903074, -4.330127018922194537, 2.499999999999995559 ) ) ;
#14948=CARTESIAN_POINT ( 'NONE',  ( 28.88437500061451502, 4.119189519843966529, 2.378215178124999607 ) ) ;
#14984=CARTESIAN_POINT ( 'NONE',  ( 13.92187500061451644, 4.119189519843966529, 2.378215178124999607 ) ) ;
#14998=CARTESIAN_POINT ( 'NONE',  ( 15.31875000122903252, -5.773502691896255534, -1.060575238724906372E-15 ) ) ;
#14999=CARTESIAN_POINT ( 'NONE',  ( 9.656250001229032875, 4.330127018922192761, -2.499999999999997780 ) ) ;
#15002=CARTESIAN_POINT ( 'NONE',  ( 8.643750001229031810, -2.886751345948181946, -4.999999999999904077 ) ) ;
#15003=CARTESIAN_POINT ( 'NONE',  ( 18.04687500061451999, 5.492252693125287522, 3.363034840372157021E-16 ) ) ;
#15019=CARTESIAN_POINT ( 'NONE',  ( 29.11875000122903501, 2.886751345948126879, 4.999999999999999112 ) ) ;
#15045=CARTESIAN_POINT ( 'NONE',  ( 28.23750000000000426, -2.886751345948129988, 4.999999999999997335 ) ) ;
#15050=EDGE_CURVE ( 'NONE', #42983, #31892, #42611, .T. ) ;
#15055=CARTESIAN_POINT ( 'NONE',  ( 22.53749999999999787, -2.886751345948153968, -4.999999999999952038 ) ) ;
#15068=CARTESIAN_POINT ( 'NONE',  ( 20.55937500061451217, 2.746126346562645981, -4.756430356249997438 ) ) ;
#15072=CARTESIAN_POINT ( 'NONE',  ( 15.59999999999999964, 0.000000000000000000, 4.999999999999998224 ) ) ;
#15077=CARTESIAN_POINT ( 'NONE',  ( 12.59999999999999964, -4.330127018922190985, -2.500000000000001332 ) ) ;
#15084=CARTESIAN_POINT ( 'NONE',  ( 25.09687500061451715, -2.746126346562642428, -4.756430356249999214 ) ) ;
#15095=ORIENTED_EDGE ( 'NONE', *, *, #2515, .T. ) ;
#15105=CARTESIAN_POINT ( 'NONE',  ( 9.984375000614518214, 4.119189519843966529, 2.378215178124999607 ) ) ;
#15120=CARTESIAN_POINT ( 'NONE',  ( 14.75625000122903252, 0.000000000000000000, 4.999999999999998224 ) ) ;
#15131=CARTESIAN_POINT ( 'NONE',  ( 13.35937500061451821, -4.119189519843965641, -2.378215178125001383 ) ) ;
#15146=CARTESIAN_POINT ( 'NONE',  ( 20.11875000122903145, 2.886751345948182834, 4.999999999999902300 ) ) ;
#15150=CARTESIAN_POINT ( 'NONE',  ( 18.98437500061451289, -2.746126346562646425, 4.756430356249996549 ) ) ;
#15165=CARTESIAN_POINT ( 'NONE',  ( 9.721875000614517148, 5.824947211148865298E-16, -4.756430356249998326 ) ) ;
#15171=LINE ( 'NONE', #61339, #57274 ) ;
#15188=CARTESIAN_POINT ( 'NONE',  ( 16.54687500061451644, -2.746126346562641984, -4.756430356249999214 ) ) ;
#15202=DIRECTION ( 'NONE',  ( -1.000000000000000000, -0.000000000000000000, -0.000000000000000000 ) ) ;
#15217=ORIENTED_EDGE ( 'NONE', *, *, #29254, .T. ) ;
#15221=CARTESIAN_POINT ( 'NONE',  ( 21.30937500061451573, 0.000000000000000000, 4.756430356249998326 ) ) ;
#15227=CARTESIAN_POINT ( 'NONE',  ( 22.76249999999999574, 2.886751345948126879, 4.999999999999999112 ) ) ;
#15231=CARTESIAN_POINT ( 'NONE',  ( 21.67500000000000071, 6.123233995736764310E-16, -4.999999999999998224 ) ) ;
#15232=CARTESIAN_POINT ( 'NONE',  ( 18.50625000122903430, -4.330127018922190985, -2.500000000000001332 ) ) ;
#15239=CARTESIAN_POINT ( 'NONE',  ( 7.631250001229033408, -4.330127018922194537, 2.499999999999995559 ) ) ;
#15241=CARTESIAN_POINT ( 'NONE',  ( 14.37187500061451573, 4.119189519843966529, 2.378215178124999607 ) ) ;
#15248=CARTESIAN_POINT ( 'NONE',  ( 12.22499999999999964, 6.123233995736764310E-16, -4.999999999999998224 ) ) ;
#15252=CARTESIAN_POINT ( 'NONE',  ( 9.234375000614514661, -2.746126346562642428, -4.756430356249999214 ) ) ;
#15257=ORIENTED_EDGE ( 'NONE', *, *, #11681, .T. ) ;
#15261=CARTESIAN_POINT ( 'NONE',  ( 45.00000000000000000, 0.000000000000000000, 4.999999999999998224 ) ) ;
#15274=CARTESIAN_POINT ( 'NONE',  ( 24.90937500061451715, 0.000000000000000000, 4.756430356249998326 ) ) ;
#15276=CARTESIAN_POINT ( 'NONE',  ( 7.734375000614517326, 4.119189519843966529, 2.378215178124999607 ) ) ;
#15293=CARTESIAN_POINT ( 'NONE',  ( 17.79375000122903572, 5.773502691896255534, 3.535250795749688894E-16 ) ) ;
#15295=CARTESIAN_POINT ( 'NONE',  ( 21.28125000122903288, 6.123233995736764310E-16, -4.999999999999998224 ) ) ;
#15301=CARTESIAN_POINT ( 'NONE',  ( 45.00000000000000000, 0.000000000000000000, 4.999999999999998224 ) ) ;
#15303=ADVANCED_FACE ( 'NONE', ( #4915, #1187 ), #7805, .F. ) ;
#15309=CARTESIAN_POINT ( 'NONE',  ( 28.09687500061451360, -2.746126346562646425, 4.756430356249996549 ) ) ;
#15317=CARTESIAN_POINT ( 'NONE',  ( 7.406250001229033764, 4.330127018922192761, -2.499999999999997780 ) ) ;
#15330=LINE ( 'NONE', #4637, #32466 ) ;
#15334=EDGE_CURVE ( 'NONE', #9134, #61283, #11898, .T. ) ;
#15338=ORIENTED_EDGE ( 'NONE', *, *, #24303, .F. ) ;
#15345=CARTESIAN_POINT ( 'NONE',  ( 15.08437500061451431, -2.746126346562642428, -4.756430356249999214 ) ) ;
#15359=CARTESIAN_POINT ( 'NONE',  ( 9.468750001229032875, -5.773502691896255534, -1.060575238724906372E-15 ) ) ;
#15364=CARTESIAN_POINT ( 'NONE',  ( 16.32187500061451502, 2.746126346562643317, 4.756430356249998326 ) ) ;
#15375=CARTESIAN_POINT ( 'NONE',  ( 13.18125000122903323, 6.123233995736764310E-16, -4.999999999999998224 ) ) ;
#15382=CARTESIAN_POINT ( 'NONE',  ( 26.41875000122903216, 2.886751345948126879, 4.999999999999999112 ) ) ;
#15384=LINE ( 'NONE', #3592, #7753 ) ;
#15410=( BOUNDED_CURVE ( )  B_SPLINE_CURVE ( 2, ( #10924, #61892, #11297, #50459, #39743, #56361, #40102, #62615, #32735, #5751, #28285, #22009, #219, #55272, #4667, #33093, #45277, #67810, #27197, #49732, #72259, #44194, #66725, #38646, #44565, #68535, #18621, #2028, #68894, #1299, #24172, #40824, #52622, #41186, #7194, #17896, #34535, #57065, #12368, #62972, #45998, #23452, #6834, #13438, #30084, #18251, #12727, #58144, #6472, #52260, #23809, #24539, #34903, #46724, #29007, #51544, #945, #63341, #35988, #35263, #46360, #63695, #7550, #51901, #47083, #41540, #57785, #40456, #13086, #69259, #29722, #57430, #35624, #29369, #1663, #69617, #18979, #64058, #12012, #23316, #16326, #67678, #4894, #34404, #45511, #68399, #809, #67326, #27428, #45865, #17760, #27795, #45145, #61398, #40320, #66960, #441, #62842, #12235, #51045, #34765, #5977, #11519, #22951, #72484, #17049, #49960, #39606, #33684, #56932, #28158, #68041, #5253, #16686, #6336, #28507, #11159, #50332, #28867, #44432, #51406, #38879, #55864, #10791, #22594, #33326, #72856, #22238, #56580, #61756, #62127, #34041, #50686, #62482, #39242, #21870, #44793, #56229, #17411, #39968, #5622, #89, #11880, #1532, #12601, #2606, #42135, #6704, #64661, #35133, #46225, #1169, #29237, #19579, #57658, #2250, #30678, #7421, #63568, #58373, #29949, #7064, #29592, #24039, #52129, #68764, #58740, #41055, #14046, #57299, #18122, #46589, #51770, #36224, #52489, #24404, #64293, #23678, #13311, #12956, #8151, #7785, #40687, #63204, #69131, #1900, #18489, #58013, #35493, #46953, #69490, #18849, #53210, #41410, #63926, #35850, #52852, #30322, #47309, #24766, #69843, #19209, #41764, #13680, #25128, #47669, #70204, #54865, #10167, #67774, #72587, #67421, #5354, #28251, #33783, #27163, #60387, #5715, #50782, #60759, #4992, #67062, #39341, #44886, #27892, #50426, #185, #4273, #21603, #38977, #44529, #10890, #32328, #27524, #22690, #50057, #66686, #16783, #61133, #33418, #38229, #56326, #26797, #9795, #61493, #21235, #55238, #38610, #49331, #22334, #45241, #44157, #4633, #66314, #37868, #71863, #43787, #15691, #32701, #49697, #72224, #61853, #16419, #16061, #10530, #55958, #33058, #55597, #21970, #72952, #11261, #40067, #57029, #11978, #6074, #18586, #908, #47047, #17149, #51143, #6435, #7159, #39707, #62225, #68859, #17860, #23416, #24503, #11621, #52586, #542, #6799, #13050, #45608, #18215, #23053, #28970, #35230, #46687, #29688, #69225, #63659, #68142, #51508, #45963, #12693, #34137, #52225, #40788, #17506, #62581, #41151, #51863, #63301, #1992, #35589, #34501, #56676, #68496, #28607, #1265, #40419, #58108, #62936, #23772, #12329, #34865, #1629, #57751, #57392, #7515, #46324, #30046, #24136, #29333, #59569, #37418, #13401, #53308, #70665, #3075, #3816, #59202, #54056, #14879, #71037, #31139, #25603, #20041, #48141, #42596, #65489, #35948, #18943, #65122, #52946, #13780, #70305, #14146, #30418, #47407, #58469, #2343, #64390, #64022, #69937, #19307, #42231, #14512, #20412, #9348, #7882, #37045, #48510, #41860, #24860, #36322, #26337, #53680, #25969, #8983, #58837, #31515, #8247, #30777, #3451, #42960, #41502, #59941, #31881, #54415, #69581, #2707, #25223, #47769, #19678, #64756, #36681, #8610, #21879, #43337, #33336, #67335, #50341, #10441, #4904, #49970, #27440, #55511, #44802, #15241, #71406, #72494, #32243, #66222, #49606, #66594, #9709, #26710, #54776, #44440, #43701, #65859, #49244, #71779, #21513, #66969, #72865, #61765, #37778, #16334, #60298, #55874, #16695, #55148, #15600, #4181, #39253, #33693, #20781, #56239, #21147, #38142, #38889, #5261, #61407, #60666, #10079, #10801, #32610, #4546, #15970, #27075, #72133, #44066, #38520, #61043, #32971, #22248, #27805, #5631, #11169, #48876, #17770, #18130, #50695, #58022, #6713, #28877, #11889, #35503, #22603, #63578, #11529, #40330, #24051, #56590, #29246, #34050, #68051, #46234, #40697, #57667, #34414, #7073, #41064, #56942, #5986, #68774, #1178, #34776, #28516, #12610, #67687, #51056, #63214, #35144, #451, #97, #45155, #22960, #28168, #17058, #62136, #17420, #12965, #29602, #51416, #68408, #52138, #39617, #57308, #6346, #1541, #45520, #51778, #39979, #62491, #818, #23326, #45876, #46598, #69140, #18499, #62851, #12245, #23686, #20323, #36236, #13321, #25513, #53590, #14057, #35860, #65035, #46963, #58383, #48058, #19959, #70215, #30689, #24414, #52862, #37332, #42145, #36961, #70583, #70952, #3365, #69853, #29958, #48426, #42877, #30334, #47679, #63936, #65400, #69499, #2985, #14791, #7432, #18859, #64303, #8524, #36596, #42511, #1909, #19589, #52499, #64672, #58750, #59483, #53220, #14426, #7795, #19220, #8895, #31053, #13692, #2262, #31427, #8160, #25138, #41420, #24776, #47320, #59117, #2617, #53967, #25886, #41774, #44356, #21064, #38805, #50255, #72778, #38430, #49522, #9626, #9990, #16249 ),
 .UNSPECIFIED., .F., .F. ) 
 B_SPLINE_CURVE_WITH_KNOTS ( ( 3, 2, 2, 2, 2, 2, 2, 2, 2, 2, 2, 2, 2, 2, 2, 2, 2, 2, 2, 2, 2, 2, 2, 2, 2, 2, 2, 2, 2, 2, 2, 2, 2, 2, 2, 2, 2, 2, 2, 2, 2, 2, 2, 2, 2, 2, 2, 2, 2, 2, 2, 2, 2, 2, 2, 2, 2, 2, 2, 2, 2, 2, 2, 2, 2, 2, 2, 2, 2, 2, 2, 2, 2, 2, 2, 2, 2, 2, 2, 2, 2, 2, 2, 2, 2, 2, 2, 2, 2, 2, 2, 2, 2, 2, 2, 2, 2, 2, 2, 2, 2, 2, 2, 2, 2, 2, 2, 2, 2, 2, 2, 2, 2, 2, 2, 2, 2, 2, 2, 2, 2, 2, 2, 2, 2, 2, 2, 2, 2, 2, 2, 2, 2, 2, 2, 2, 2, 2, 2, 2, 2, 2, 2, 2, 2, 2, 2, 2, 2, 2, 2, 2, 2, 2, 2, 2, 2, 2, 2, 2, 2, 2, 2, 2, 2, 2, 2, 2, 2, 2, 2, 2, 2, 2, 2, 2, 2, 2, 2, 2, 2, 2, 2, 2, 2, 2, 2, 2, 2, 2, 2, 2, 2, 2, 2, 2, 2, 2, 2, 2, 2, 2, 2, 2, 2, 2, 2, 2, 2, 2, 2, 2, 2, 2, 2, 2, 2, 2, 2, 2, 2, 2, 2, 2, 2, 2, 2, 2, 2, 2, 2, 2, 2, 2, 2, 2, 2, 2, 2, 2, 2, 2, 2, 2, 2, 2, 2, 2, 2, 2, 2, 2, 2, 2, 2, 2, 2, 2, 2, 2, 2, 2, 2, 2, 2, 2, 2, 2, 2, 2, 2, 2, 2, 2, 2, 2, 2, 2, 2, 2, 2, 2, 2, 2, 2, 2, 2, 2, 2, 2, 2, 2, 2, 2, 2, 2, 2, 2, 2, 2, 3 ),
 ( 0.000000000000000000, 0.003333333333333333547, 0.006666666666666667095, 0.01000000000000000021, 0.01333333333333333419, 0.01666666666666666644, 0.02000000000000000042, 0.02333333333333333440, 0.02666666666666666838, 0.02999999999999999889, 0.03333333333333333287, 0.03666666666666666685, 0.04000000000000000083, 0.04333333333333333481, 0.04666666666666666879, 0.05000000000000000278, 0.05333333333333333676, 0.05666666666666666380, 0.05999999999999999778, 0.06333333333333333870, 0.06666666666666666574, 0.07000000000000000666, 0.07333333333333333370, 0.07666666666666666075, 0.08000000000000000167, 0.08333333333333332871, 0.08666666666666666963, 0.08999999999999999667, 0.09333333333333333759, 0.09666666666666666463, 0.1000000000000000056, 0.1033333333333333326, 0.1066666666666666735, 0.1100000000000000006, 0.1133333333333333276, 0.1166666666666666685, 0.1199999999999999956, 0.1233333333333333365, 0.1266666666666666774, 0.1300000000000000044, 0.1333333333333333315, 0.1366666666666666585, 0.1400000000000000133, 0.1433333333333333404, 0.1466666666666666674, 0.1499999999999999944, 0.1533333333333333215, 0.1566666666666666763, 0.1600000000000000033, 0.1633333333333333304, 0.1666666666666666574, 0.1700000000000000122, 0.1733333333333333393, 0.1766666666666666663, 0.1799999999999999933, 0.1833333333333333204, 0.1866666666666666752, 0.1900000000000000022, 0.1933333333333333293, 0.1966666666666666563, 0.2000000000000000111, 0.2033333333333333381, 0.2066666666666666652, 0.2099999999999999922, 0.2133333333333333470, 0.2166666666666666741, 0.2200000000000000011, 0.2233333333333333282, 0.2266666666666666552, 0.2300000000000000100, 0.2333333333333333370, 0.2366666666666666641, 0.2399999999999999911, 0.2433333333333333459, 0.2466666666666666730, 0.2500000000000000000, 0.2533333333333333548, 0.2566666666666666541, 0.2600000000000000089, 0.2633333333333333082, 0.2666666666666666630, 0.2700000000000000178, 0.2733333333333333171, 0.2766666666666666718, 0.2800000000000000266, 0.2833333333333333259, 0.2866666666666666807, 0.2899999999999999800, 0.2933333333333333348, 0.2966666666666666896, 0.2999999999999999889, 0.3033333333333333437, 0.3066666666666666430, 0.3099999999999999978, 0.3133333333333333526, 0.3166666666666666519, 0.3200000000000000067, 0.3233333333333333059, 0.3266666666666666607, 0.3300000000000000155, 0.3333333333333333148, 0.3366666666666666696, 0.3400000000000000244, 0.3433333333333333237, 0.3466666666666666785, 0.3499999999999999778, 0.3533333333333333326, 0.3566666666666666874, 0.3599999999999999867, 0.3633333333333333415, 0.3666666666666666408, 0.3699999999999999956, 0.3733333333333333504, 0.3766666666666666496, 0.3800000000000000044, 0.3833333333333333592, 0.3866666666666666585, 0.3900000000000000133, 0.3933333333333333126, 0.3966666666666666674, 0.4000000000000000222, 0.4033333333333333215, 0.4066666666666666763, 0.4099999999999999756, 0.4133333333333333304, 0.4166666666666666852, 0.4199999999999999845, 0.4233333333333333393, 0.4266666666666666941, 0.4299999999999999933, 0.4333333333333333481, 0.4366666666666666474, 0.4400000000000000022, 0.4433333333333333570, 0.4466666666666666563, 0.4500000000000000111, 0.4533333333333333104, 0.4566666666666666652, 0.4600000000000000200, 0.4633333333333333193, 0.4666666666666666741, 0.4699999999999999734, 0.4733333333333333282, 0.4766666666666666829, 0.4799999999999999822, 0.4833333333333333370, 0.4866666666666666918, 0.4899999999999999911, 0.4933333333333333459, 0.4966666666666666452, 0.5000000000000000000, 0.5033333333333332993, 0.5066666666666667096, 0.5100000000000000089, 0.5133333333333333082, 0.5166666666666667185, 0.5200000000000000178, 0.5233333333333333171, 0.5266666666666666163, 0.5300000000000000266, 0.5333333333333333259, 0.5366666666666666252, 0.5400000000000000355, 0.5433333333333333348, 0.5466666666666666341, 0.5500000000000000444, 0.5533333333333333437, 0.5566666666666666430, 0.5600000000000000533, 0.5633333333333333526, 0.5666666666666666519, 0.5699999999999999512, 0.5733333333333333615, 0.5766666666666666607, 0.5799999999999999600, 0.5833333333333333703, 0.5866666666666666696, 0.5899999999999999689, 0.5933333333333333792, 0.5966666666666666785, 0.5999999999999999778, 0.6033333333333333881, 0.6066666666666666874, 0.6099999999999999867, 0.6133333333333332860, 0.6166666666666666963, 0.6199999999999999956, 0.6233333333333332948, 0.6266666666666667052, 0.6300000000000000044, 0.6333333333333333037, 0.6366666666666667140, 0.6400000000000000133, 0.6433333333333333126, 0.6466666666666666119, 0.6500000000000000222, 0.6533333333333333215, 0.6566666666666666208, 0.6600000000000000311, 0.6633333333333333304, 0.6666666666666666297, 0.6700000000000000400, 0.6733333333333333393, 0.6766666666666666385, 0.6800000000000000488, 0.6833333333333333481, 0.6866666666666666474, 0.6899999999999999467, 0.6933333333333333570, 0.6966666666666666563, 0.6999999999999999556, 0.7033333333333333659, 0.7066666666666666652, 0.7099999999999999645, 0.7133333333333333748, 0.7166666666666666741, 0.7199999999999999734, 0.7233333333333333837, 0.7266666666666666829, 0.7299999999999999822, 0.7333333333333332815, 0.7366666666666666918, 0.7399999999999999911, 0.7433333333333332904, 0.7466666666666667007, 0.7500000000000000000, 0.7533333333333332993, 0.7566666666666667096, 0.7600000000000000089, 0.7633333333333333082, 0.7666666666666667185, 0.7700000000000000178, 0.7733333333333333171, 0.7766666666666666163, 0.7800000000000000266, 0.7833333333333333259, 0.7866666666666666252, 0.7900000000000000355, 0.7933333333333333348, 0.7966666666666666341, 0.8000000000000000444, 0.8033333333333333437, 0.8066666666666666430, 0.8100000000000000533, 0.8133333333333333526, 0.8166666666666666519, 0.8199999999999999512, 0.8233333333333333615, 0.8266666666666666607, 0.8299999999999999600, 0.8333333333333333703, 0.8366666666666666696, 0.8399999999999999689, 0.8433333333333333792, 0.8466666666666666785, 0.8499999999999999778, 0.8533333333333333881, 0.8566666666666666874, 0.8599999999999999867, 0.8633333333333332860, 0.8666666666666666963, 0.8699999999999999956, 0.8733333333333332948, 0.8766666666666667052, 0.8800000000000000044, 0.8833333333333333037, 0.8866666666666667140, 0.8900000000000000133, 0.8933333333333333126, 0.8966666666666666119, 0.9000000000000000222, 0.9033333333333333215, 0.9066666666666666208, 0.9100000000000000311, 0.9133333333333333304, 0.9166666666666666297, 0.9200000000000000400, 0.9233333333333333393, 0.9266666666666666385, 0.9300000000000000488, 0.9333333333333333481, 0.9366666666666666474, 0.9399999999999999467, 0.9433333333333333570, 0.9466666666666666563, 0.9499999999999999556, 0.9533333333333333659, 0.9566666666666666652, 0.9599999999999999645, 0.9633333333333333748, 0.9666666666666666741, 0.9699999999999999734, 0.9733333333333333837, 0.9766666666666666829, 0.9799999999999999822, 0.9833333333333332815, 0.9866666666666666918, 0.9899999999999999911, 0.9933333333333332904, 0.9966666666666667007, 1.000000000000000000 ),
 .UNSPECIFIED. ) 
 CURVE ( )  GEOMETRIC_REPRESENTATION_ITEM ( )  RATIONAL_B_SPLINE_CURVE ( ( 1.000000000000000000, 0.8660254037844387076, 1.000000000000000000, 0.8660254037844387076, 1.000000000000000000, 0.8660254037844387076, 1.000000000000000000, 0.8660254037844387076, 1.000000000000000000, 0.8660254037844387076, 1.000000000000000000, 0.8660254037844387076, 1.000000000000000000, 0.8660254037844387076, 1.000000000000000000, 0.8660254037844387076, 1.000000000000000000, 0.8660254037844387076, 1.000000000000000000, 0.8660254037844387076, 1.000000000000000000, 0.8660254037844387076, 1.000000000000000000, 0.8660254037844387076, 1.000000000000000000, 0.8660254037844387076, 1.000000000000000000, 0.8660254037844387076, 1.000000000000000000, 0.8660254037844387076, 1.000000000000000000, 0.8660254037844387076, 1.000000000000000000, 0.8660254037844387076, 1.000000000000000000, 0.8660254037844387076, 1.000000000000000000, 0.8660254037844387076, 1.000000000000000000, 0.8660254037844387076, 1.000000000000000000, 0.8660254037844387076, 1.000000000000000000, 0.8660254037844387076, 1.000000000000000000, 0.8660254037844387076, 1.000000000000000000, 0.8660254037844387076, 1.000000000000000000, 0.8660254037844387076, 1.000000000000000000, 0.8660254037844387076, 1.000000000000000000, 0.8660254037844387076, 1.000000000000000000, 0.8660254037844387076, 1.000000000000000000, 0.8660254037844387076, 1.000000000000000000, 0.8660254037844387076, 1.000000000000000000, 0.8660254037844387076, 1.000000000000000000, 0.8660254037844387076, 1.000000000000000000, 0.8660254037844387076, 1.000000000000000000, 0.8660254037844387076, 1.000000000000000000, 0.8660254037844387076, 1.000000000000000000, 0.8660254037844387076, 1.000000000000000000, 0.8660254037844387076, 1.000000000000000000, 0.8660254037844387076, 1.000000000000000000, 0.8660254037844387076, 1.000000000000000000, 0.8660254037844387076, 1.000000000000000000, 0.8660254037844387076, 1.000000000000000000, 0.8660254037844387076, 1.000000000000000000, 0.8660254037844387076, 1.000000000000000000, 0.8660254037844387076, 1.000000000000000000, 0.8660254037844387076, 1.000000000000000000, 0.8660254037844387076, 1.000000000000000000, 0.8660254037844387076, 1.000000000000000000, 0.8660254037844387076, 1.000000000000000000, 0.8660254037844387076, 1.000000000000000000, 0.8660254037844387076, 1.000000000000000000, 0.8660254037844387076, 1.000000000000000000, 0.8660254037844387076, 1.000000000000000000, 0.8660254037844387076, 1.000000000000000000, 0.8660254037844387076, 1.000000000000000000, 0.8660254037844387076, 1.000000000000000000, 0.8660254037844387076, 1.000000000000000000, 0.8660254037844387076, 1.000000000000000000, 0.8660254037844387076, 1.000000000000000000, 0.8660254037844387076, 1.000000000000000000, 0.8660254037844387076, 1.000000000000000000, 0.8660254037844387076, 1.000000000000000000, 0.8660254037844387076, 1.000000000000000000, 0.8660254037844387076, 1.000000000000000000, 0.8660254037844387076, 1.000000000000000000, 0.8660254037844387076, 1.000000000000000000, 0.8660254037844387076, 1.000000000000000000, 0.8660254037844387076, 1.000000000000000000, 0.8660254037844387076, 1.000000000000000000, 0.8660254037844387076, 1.000000000000000000, 0.8660254037844387076, 1.000000000000000000, 0.8660254037844387076, 1.000000000000000000, 0.8660254037844387076, 1.000000000000000000, 0.8660254037844387076, 1.000000000000000000, 0.8660254037844387076, 1.000000000000000000, 0.8660254037844387076, 1.000000000000000000, 0.8660254037844387076, 1.000000000000000000, 0.8660254037844387076, 1.000000000000000000, 0.8660254037844387076, 1.000000000000000000, 0.8660254037844387076, 1.000000000000000000, 0.8660254037844387076, 1.000000000000000000, 0.8660254037844387076, 1.000000000000000000, 0.8660254037844387076, 1.000000000000000000, 0.8660254037844387076, 1.000000000000000000, 0.8660254037844387076, 1.000000000000000000, 0.8660254037844387076, 1.000000000000000000, 0.8660254037844387076, 1.000000000000000000, 0.8660254037844387076, 1.000000000000000000, 0.8660254037844387076, 1.000000000000000000, 0.8660254037844387076, 1.000000000000000000, 0.8660254037844387076, 1.000000000000000000, 0.8660254037844387076, 1.000000000000000000, 0.8660254037844387076, 1.000000000000000000, 0.8660254037844387076, 1.000000000000000000, 0.8660254037844387076, 1.000000000000000000, 0.8660254037844387076, 1.000000000000000000, 0.8660254037844387076, 1.000000000000000000, 0.8660254037844387076, 1.000000000000000000, 0.8660254037844387076, 1.000000000000000000, 0.8660254037844387076, 1.000000000000000000, 0.8660254037844387076, 1.000000000000000000, 0.8660254037844387076, 1.000000000000000000, 0.8660254037844387076, 1.000000000000000000, 0.8660254037844387076, 1.000000000000000000, 0.8660254037844387076, 1.000000000000000000, 0.8660254037844387076, 1.000000000000000000, 0.8660254037844387076, 1.000000000000000000, 0.8660254037844387076, 1.000000000000000000, 0.8660254037844387076, 1.000000000000000000, 0.8660254037844387076, 1.000000000000000000, 0.8660254037844387076, 1.000000000000000000, 0.8660254037844387076, 1.000000000000000000, 0.8660254037844387076, 1.000000000000000000, 0.8660254037844387076, 1.000000000000000000, 0.8660254037844387076, 1.000000000000000000, 0.8660254037844387076, 1.000000000000000000, 0.8660254037844387076, 1.000000000000000000, 0.8660254037844387076, 1.000000000000000000, 0.8660254037844387076, 1.000000000000000000, 0.8660254037844387076, 1.000000000000000000, 0.8660254037844387076, 1.000000000000000000, 0.8660254037844387076, 1.000000000000000000, 0.8660254037844387076, 1.000000000000000000, 0.8660254037844387076, 1.000000000000000000, 0.8660254037844387076, 1.000000000000000000, 0.8660254037844387076, 1.000000000000000000, 0.8660254037844387076, 1.000000000000000000, 0.8660254037844387076, 1.000000000000000000, 0.8660254037844387076, 1.000000000000000000, 0.8660254037844387076, 1.000000000000000000, 0.8660254037844387076, 1.000000000000000000, 0.8660254037844387076, 1.000000000000000000, 0.8660254037844387076, 1.000000000000000000, 0.8660254037844387076, 1.000000000000000000, 0.8660254037844387076, 1.000000000000000000, 0.8660254037844387076, 1.000000000000000000, 0.8660254037844387076, 1.000000000000000000, 0.8660254037844387076, 1.000000000000000000, 0.8660254037844387076, 1.000000000000000000, 0.8660254037844387076, 1.000000000000000000, 0.8660254037844387076, 1.000000000000000000, 0.8660254037844387076, 1.000000000000000000, 0.8660254037844387076, 1.000000000000000000, 0.8660254037844387076, 1.000000000000000000, 0.8660254037844387076, 1.000000000000000000, 0.8660254037844387076, 1.000000000000000000, 0.8660254037844387076, 1.000000000000000000, 0.8660254037844387076, 1.000000000000000000, 0.8660254037844387076, 1.000000000000000000, 0.8660254037844387076, 1.000000000000000000, 0.8660254037844387076, 1.000000000000000000, 0.8660254037844387076, 1.000000000000000000, 0.8660254037844387076, 1.000000000000000000, 0.8660254037844387076, 1.000000000000000000, 0.8660254037844387076, 1.000000000000000000, 0.8660254037844387076, 1.000000000000000000, 0.8660254037844387076, 1.000000000000000000, 0.8660254037844387076, 1.000000000000000000, 0.8660254037844387076, 1.000000000000000000, 0.8660254037844387076, 1.000000000000000000, 0.8660254037844387076, 1.000000000000000000, 0.8660254037844387076, 1.000000000000000000, 0.8660254037844387076, 1.000000000000000000, 0.8660254037844387076, 1.000000000000000000, 0.8660254037844387076, 1.000000000000000000, 0.8660254037844387076, 1.000000000000000000, 0.8660254037844387076, 1.000000000000000000, 0.8660254037844387076, 1.000000000000000000, 0.8660254037844387076, 1.000000000000000000, 0.8660254037844387076, 1.000000000000000000, 0.8660254037844387076, 1.000000000000000000, 0.8660254037844387076, 1.000000000000000000, 0.8660254037844387076, 1.000000000000000000, 0.8660254037844387076, 1.000000000000000000, 0.8660254037844387076, 1.000000000000000000, 0.8660254037844387076, 1.000000000000000000, 0.8660254037844387076, 1.000000000000000000, 0.8660254037844387076, 1.000000000000000000, 0.8660254037844387076, 1.000000000000000000, 0.8660254037844387076, 1.000000000000000000, 0.8660254037844387076, 1.000000000000000000, 0.8660254037844387076, 1.000000000000000000, 0.8660254037844387076, 1.000000000000000000, 0.8660254037844387076, 1.000000000000000000, 0.8660254037844387076, 1.000000000000000000, 0.8660254037844387076, 1.000000000000000000, 0.8660254037844387076, 1.000000000000000000, 0.8660254037844387076, 1.000000000000000000, 0.8660254037844387076, 1.000000000000000000, 0.8660254037844387076, 1.000000000000000000, 0.8660254037844387076, 1.000000000000000000, 0.8660254037844387076, 1.000000000000000000, 0.8660254037844387076, 1.000000000000000000, 0.8660254037844387076, 1.000000000000000000, 0.8660254037844387076, 1.000000000000000000, 0.8660254037844387076, 1.000000000000000000, 0.8660254037844387076, 1.000000000000000000, 0.8660254037844387076, 1.000000000000000000, 0.8660254037844387076, 1.000000000000000000, 0.8660254037844387076, 1.000000000000000000, 0.8660254037844387076, 1.000000000000000000, 0.8660254037844387076, 1.000000000000000000, 0.8660254037844387076, 1.000000000000000000, 0.8660254037844387076, 1.000000000000000000, 0.8660254037844387076, 1.000000000000000000, 0.8660254037844387076, 1.000000000000000000, 0.8660254037844387076, 1.000000000000000000, 0.8660254037844387076, 1.000000000000000000, 0.8660254037844387076, 1.000000000000000000, 0.8660254037844387076, 1.000000000000000000, 0.8660254037844387076, 1.000000000000000000, 0.8660254037844387076, 1.000000000000000000, 0.8660254037844387076, 1.000000000000000000, 0.8660254037844387076, 1.000000000000000000, 0.8660254037844387076, 1.000000000000000000, 0.8660254037844387076, 1.000000000000000000, 0.8660254037844387076, 1.000000000000000000, 0.8660254037844387076, 1.000000000000000000, 0.8660254037844387076, 1.000000000000000000, 0.8660254037844387076, 1.000000000000000000, 0.8660254037844387076, 1.000000000000000000, 0.8660254037844387076, 1.000000000000000000, 0.8660254037844387076, 1.000000000000000000, 0.8660254037844387076, 1.000000000000000000, 0.8660254037844387076, 1.000000000000000000, 0.8660254037844387076, 1.000000000000000000, 0.8660254037844387076, 1.000000000000000000, 0.8660254037844387076, 1.000000000000000000, 0.8660254037844387076, 1.000000000000000000, 0.8660254037844387076, 1.000000000000000000, 0.8660254037844387076, 1.000000000000000000, 0.8660254037844387076, 1.000000000000000000, 0.8660254037844387076, 1.000000000000000000, 0.8660254037844387076, 1.000000000000000000, 0.8660254037844387076, 1.000000000000000000, 0.8660254037844387076, 1.000000000000000000, 0.8660254037844387076, 1.000000000000000000, 0.8660254037844387076, 1.000000000000000000, 0.8660254037844387076, 1.000000000000000000, 0.8660254037844387076, 1.000000000000000000, 0.8660254037844387076, 1.000000000000000000, 0.8660254037844387076, 1.000000000000000000, 0.8660254037844387076, 1.000000000000000000, 0.8660254037844387076, 1.000000000000000000, 0.8660254037844387076, 1.000000000000000000, 0.8660254037844387076, 1.000000000000000000, 0.8660254037844387076, 1.000000000000000000, 0.8660254037844387076, 1.000000000000000000, 0.8660254037844387076, 1.000000000000000000, 0.8660254037844387076, 1.000000000000000000, 0.8660254037844387076, 1.000000000000000000, 0.8660254037844387076, 1.000000000000000000, 0.8660254037844387076, 1.000000000000000000, 0.8660254037844387076, 1.000000000000000000, 0.8660254037844387076, 1.000000000000000000, 0.8660254037844387076, 1.000000000000000000, 0.8660254037844387076, 1.000000000000000000, 0.8660254037844387076, 1.000000000000000000, 0.8660254037844387076, 1.000000000000000000, 0.8660254037844387076, 1.000000000000000000, 0.8660254037844387076, 1.000000000000000000, 0.8660254037844387076, 1.000000000000000000, 0.8660254037844387076, 1.000000000000000000, 0.8660254037844387076, 1.000000000000000000, 0.8660254037844387076, 1.000000000000000000, 0.8660254037844387076, 1.000000000000000000, 0.8660254037844387076, 1.000000000000000000, 0.8660254037844387076, 1.000000000000000000, 0.8660254037844387076, 1.000000000000000000, 0.8660254037844387076, 1.000000000000000000, 0.8660254037844387076, 1.000000000000000000, 0.8660254037844387076, 1.000000000000000000, 0.8660254037844387076, 1.000000000000000000, 0.8660254037844387076, 1.000000000000000000, 0.8660254037844387076, 1.000000000000000000, 0.8660254037844387076, 1.000000000000000000, 0.8660254037844387076, 1.000000000000000000, 0.8660254037844387076, 1.000000000000000000, 0.8660254037844387076, 1.000000000000000000, 0.8660254037844387076, 1.000000000000000000, 0.8660254037844387076, 1.000000000000000000, 0.8660254037844387076, 1.000000000000000000, 0.8660254037844387076, 1.000000000000000000, 0.8660254037844387076, 1.000000000000000000, 0.8660254037844387076, 1.000000000000000000, 0.8660254037844387076, 1.000000000000000000, 0.8660254037844387076, 1.000000000000000000, 0.8660254037844387076, 1.000000000000000000, 0.8660254037844387076, 1.000000000000000000, 0.8660254037844387076, 1.000000000000000000, 0.8660254037844387076, 1.000000000000000000, 0.8660254037844387076, 1.000000000000000000, 0.8660254037844387076, 1.000000000000000000, 0.8660254037844387076, 1.000000000000000000, 0.8660254037844387076, 1.000000000000000000, 0.8660254037844387076, 1.000000000000000000, 0.8660254037844387076, 1.000000000000000000, 0.8660254037844387076, 1.000000000000000000, 0.8660254037844387076, 1.000000000000000000, 0.8660254037844387076, 1.000000000000000000, 0.8660254037844387076, 1.000000000000000000 ) ) 
 REPRESENTATION_ITEM ( '' )  );
#15415=CARTESIAN_POINT ( 'NONE',  ( 27.50625000122903074, -4.330127018922190985, -2.500000000000001332 ) ) ;
#15426=CARTESIAN_POINT ( 'NONE',  ( 21.75937500061451502, -5.492252693125287522, -1.008910452111647106E-15 ) ) ;
#15435=CARTESIAN_POINT ( 'NONE',  ( 12.56250000000000178, -5.773502691896255534, -1.060575238724906372E-15 ) ) ;
#15442=CARTESIAN_POINT ( 'NONE',  ( 22.54687500061451999, 5.492252693125287522, 3.363034840372157021E-16 ) ) ;
#15446=FACE_OUTER_BOUND ( 'NONE', #40806, .T. ) ;
#15464=CARTESIAN_POINT ( 'NONE',  ( 10.77187500061451786, 2.746126346562645981, -4.756430356249997438 ) ) ;
#15480=AXIS2_PLACEMENT_3D ( 'NONE', #66874, #15508, #25882 ) ;
#15491=CARTESIAN_POINT ( 'NONE',  ( 12.42187500061451821, -5.492252693125287522, -1.008910452111647106E-15 ) ) ;
#15500=CARTESIAN_POINT ( 'NONE',  ( 16.83749999999999858, 5.773502691896255534, 3.535250795749688401E-16 ) ) ;
#15508=DIRECTION ( 'NONE',  ( -1.000000000000000000, -0.000000000000000000, -0.000000000000000000 ) ) ;
#15510=CARTESIAN_POINT ( 'NONE',  ( 21.19687500061451502, 0.000000000000000000, 4.756430356249998326 ) ) ;
#15513=CARTESIAN_POINT ( 'NONE',  ( 14.30625000122903145, 0.000000000000000000, 4.999999999999998224 ) ) ;
#15527=CARTESIAN_POINT ( 'NONE',  ( 8.596875000614515372, 0.000000000000000000, 4.756430356249998326 ) ) ;
#15548=CARTESIAN_POINT ( 'NONE',  ( 17.89687500061451431, -2.746126346562641984, -4.756430356249999214 ) ) ;
#15556=EDGE_CURVE ( 'NONE', #63037, #1518, #64831, .T. ) ;
#15582=CARTESIAN_POINT ( 'NONE',  ( 18.53437500061451715, 4.119189519843966529, 2.378215178124999607 ) ) ;
#15588=CARTESIAN_POINT ( 'NONE',  ( 21.78750000000000142, 5.773502691896255534, 3.535250795749688894E-16 ) ) ;
#15598=CARTESIAN_POINT ( 'NONE',  ( 26.97187500061451360, 4.119189519843966529, 2.378215178124999607 ) ) ;
#15600=CARTESIAN_POINT ( 'NONE',  ( 13.43437500061451750, 5.492252693125287522, 3.363034840372157021E-16 ) ) ;
#15601=EDGE_CURVE ( 'NONE', #60669, #32563, #14770, .T. ) ;
#15624=VERTEX_POINT ( 'NONE', #18139 ) ;
#15629=EDGE_CURVE ( 'NONE', #8998, #45106, #27518, .T. ) ;
#15634=CARTESIAN_POINT ( 'NONE',  ( 24.04687500061451644, -2.746126346562646425, 4.756430356249996549 ) ) ;
#15636=CARTESIAN_POINT ( 'NONE',  ( 8.184375000614515727, 4.119189519843966529, 2.378215178124999607 ) ) ;
#15641=ORIENTED_EDGE ( 'NONE', *, *, #19119, .F. ) ;
#15645=( BOUNDED_CURVE ( )  B_SPLINE_CURVE ( 2, ( #28361, #50897, #297, #22806, #45358, #63779, #23896 ),
 .UNSPECIFIED., .F., .F. ) 
 B_SPLINE_CURVE_WITH_KNOTS ( ( 3, 2, 2, 3 ),
 ( 0.5200000000000000178, 0.5233333333333333171, 0.5266666666666666163, 0.5300000000000000266 ),
 .UNSPECIFIED. ) 
 CURVE ( )  GEOMETRIC_REPRESENTATION_ITEM ( )  RATIONAL_B_SPLINE_CURVE ( ( 1.000000000000000000, 0.8660254037844387076, 1.000000000000000000, 0.8660254037844387076, 1.000000000000000000, 0.8660254037844387076, 1.000000000000000000 ) ) 
 REPRESENTATION_ITEM ( '' )  );
#15647=CARTESIAN_POINT ( 'NONE',  ( 23.30625000122903145, 0.000000000000000000, 4.999999999999998224 ) ) ;
#15655=CARTESIAN_POINT ( 'NONE',  ( 19.40625000122902932, -4.330127018922190985, -2.500000000000001332 ) ) ;
#15664=CYLINDRICAL_SURFACE ( 'NONE', #34433, 4.999999999999998224 ) ;
#15666=EDGE_CURVE ( 'NONE', #30697, #34725, #16714, .T. ) ;
#15673=CARTESIAN_POINT ( 'NONE',  ( 28.65937500061451715, -4.119189519843965641, -2.378215178125001383 ) ) ;
#15685=CARTESIAN_POINT ( 'NONE',  ( 14.02499999999999858, 6.123233995736764310E-16, -4.999999999999998224 ) ) ;
#15687=CARTESIAN_POINT ( 'NONE',  ( 12.91875000122903394, 2.886751345948126879, 4.999999999999999112 ) ) ;
#15691=CARTESIAN_POINT ( 'NONE',  ( 20.10937500061451289, 2.746126346562645981, -4.756430356249997438 ) ) ;
#15694=EDGE_LOOP ( 'NONE', ( #53929, #7935, #15854, #16422 ) ) ;
#15710=CARTESIAN_POINT ( 'NONE',  ( 13.20937500061451431, -5.492252693125287522, -1.008910452111647106E-15 ) ) ;
#15728=CARTESIAN_POINT ( 'NONE',  ( 14.10937500061451644, 0.000000000000000000, 4.756430356249998326 ) ) ;
#15745=CARTESIAN_POINT ( 'NONE',  ( 26.00625000122903074, 0.000000000000000000, 4.999999999999998224 ) ) ;
#15747=DIRECTION ( 'NONE',  ( -1.000000000000000000, -0.000000000000000000, -0.000000000000000000 ) ) ;
#15774=EDGE_CURVE ( 'NONE', #26800, #29126, #35052, .T. ) ;
#15789=ORIENTED_EDGE ( 'NONE', *, *, #34218, .T. ) ;
#15796=CARTESIAN_POINT ( 'NONE',  ( 20.70937500061451786, 2.746126346562643317, 4.756430356249998326 ) ) ;
#15805=CARTESIAN_POINT ( 'NONE',  ( 12.37500000000000000, 4.330127018922191873, 2.499999999999999556 ) ) ;
#15812=CARTESIAN_POINT ( 'NONE',  ( 23.03437500061451715, 4.119189519843966529, 2.378215178124999607 ) ) ;
#15834=CARTESIAN_POINT ( 'NONE',  ( 10.17187500061451999, -5.492252693125287522, -1.008910452111647106E-15 ) ) ;
#15842=ORIENTED_EDGE ( 'NONE', *, *, #22474, .F. ) ;
#15854=ORIENTED_EDGE ( 'NONE', *, *, #41629, .T. ) ;
#15857=CARTESIAN_POINT ( 'NONE',  ( 11.10937500061451644, -4.119189519843965641, -2.378215178125001383 ) ) ;
#15867=DIRECTION ( 'NONE',  ( -1.000000000000000000, -0.000000000000000000, -0.000000000000000000 ) ) ;
#15878=EDGE_CURVE ( 'NONE', #68160, #47688, #54927, .T. ) ;
#15880=CARTESIAN_POINT ( 'NONE',  ( 20.44687500061451502, -4.119189519843965641, -2.378215178125001383 ) ) ;
#15883=CARTESIAN_POINT ( 'NONE',  ( 13.59375000122903288, -2.886751345948125991, -5.000000000000000000 ) ) ;
#15896=CARTESIAN_POINT ( 'NONE',  ( 28.47187500061451715, 2.746126346562643317, 4.756430356249998326 ) ) ;
#15901=FACE_OUTER_BOUND ( 'NONE', #49932, .T. ) ;
#15917=CARTESIAN_POINT ( 'NONE',  ( 17.74687500061451928, -2.746126346562646425, 4.756430356249996549 ) ) ;
#15929=VECTOR ( 'NONE', #38365, 1000.000000000000000 ) ;
#15937=CARTESIAN_POINT ( 'NONE',  ( 34.99999999999999289, -2.499999999999999556, 3.499999999999999556 ) ) ;
#15951=CARTESIAN_POINT ( 'NONE',  ( 18.38437500061451857, 5.824947211148865298E-16, -4.756430356249998326 ) ) ;
#15957=CARTESIAN_POINT ( 'NONE',  ( 20.88749999999999929, 5.773502691896255534, 3.535250795749688894E-16 ) ) ;
#15960=DIRECTION ( 'NONE',  ( -1.000000000000000000, -0.000000000000000000, -0.000000000000000000 ) ) ;
#15966=ADVANCED_FACE ( 'NONE', ( #13130 ), #46047, .T. ) ;
#15968=CARTESIAN_POINT ( 'NONE',  ( 26.44687500061451502, 4.119189519843966529, -2.378215178124998275 ) ) ;
#15970=CARTESIAN_POINT ( 'NONE',  ( 12.83437500061451786, -2.746126346562641984, -4.756430356249999214 ) ) ;
#15976=DIRECTION ( 'NONE',  ( -1.000000000000000000, -0.000000000000000000, -0.000000000000000000 ) ) ;
#15987=ORIENTED_EDGE ( 'NONE', *, *, #66859, .F. ) ;
#16005=CARTESIAN_POINT ( 'NONE',  ( 23.55937500061451573, 0.000000000000000000, 4.756430356249998326 ) ) ;
#16018=CARTESIAN_POINT ( 'NONE',  ( 45.00000000000000000, 0.000000000000000000, 0.000000000000000000 ) ) ;
#16026=CARTESIAN_POINT ( 'NONE',  ( 19.74375000122903145, -2.886751345948129988, 4.999999999999997335 ) ) ;
#16042=CARTESIAN_POINT ( 'NONE',  ( 25.28437500061451715, 4.119189519843966529, 2.378215178124999607 ) ) ;
#16055=CARTESIAN_POINT ( 'NONE',  ( 27.59999999999999787, 4.330127018922192761, -2.499999999999997780 ) ) ;
#16057=CARTESIAN_POINT ( 'NONE',  ( 12.99375000122903323, -2.886751345948129988, 4.999999999999997335 ) ) ;
#16061=CARTESIAN_POINT ( 'NONE',  ( 19.88437500061451502, -2.746126346562646425, 4.756430356249996549 ) ) ;
#16071=CARTESIAN_POINT ( 'NONE',  ( 14.07187500061451679, -4.119189519843968306, 2.378215178124996054 ) ) ;
#16072=ORIENTED_EDGE ( 'NONE', *, *, #893, .F. ) ;
#16081=CARTESIAN_POINT ( 'NONE',  ( 15.00937500061451502, -5.492252693125287522, -1.008910452111647106E-15 ) ) ;
#16097=CARTESIAN_POINT ( 'NONE',  ( 15.12187500061451750, -5.492252693125287522, -1.008910452111647106E-15 ) ) ;
#16108=( BOUNDED_CURVE ( )  B_SPLINE_CURVE ( 2, ( #32782, #60110, #20583, #55319, #4713, #26514, #27247 ),
 .UNSPECIFIED., .F., .F. ) 
 B_SPLINE_CURVE_WITH_KNOTS ( ( 3, 2, 2, 3 ),
 ( 0.7700000000000001288, 0.7733333333333334281, 0.7766666666666667274, 0.7800000000000001377 ),
 .UNSPECIFIED. ) 
 CURVE ( )  GEOMETRIC_REPRESENTATION_ITEM ( )  RATIONAL_B_SPLINE_CURVE ( ( 0.9999999999999955591, 0.8660254037844431485, 1.000000000000000000, 0.8660254037844387076, 1.000000000000000000, 0.8660254037844342667, 1.000000000000004441 ) ) 
 REPRESENTATION_ITEM ( '' )  );
#16115=CARTESIAN_POINT ( 'NONE',  ( 24.95625000122903003, 4.330127018922192761, -2.499999999999997780 ) ) ;
#16159=ORIENTED_EDGE ( 'NONE', *, *, #14554, .F. ) ;
#16165=CARTESIAN_POINT ( 'NONE',  ( 20.67187500061451289, 4.119189519843966529, 2.378215178124999607 ) ) ;
#16174=CARTESIAN_POINT ( 'NONE',  ( 11.06250000000000000, 2.886751345948126879, 4.999999999999999112 ) ) ;
#16182=CARTESIAN_POINT ( 'NONE',  ( 21.53437500061451715, 5.824947211148865298E-16, -4.756430356249998326 ) ) ;
#16185=DIRECTION ( 'NONE',  ( 0.000000000000000000, 0.000000000000000000, 1.000000000000000000 ) ) ;
#16193=ORIENTED_EDGE ( 'NONE', *, *, #8865, .F. ) ;
#16204=CARTESIAN_POINT ( 'NONE',  ( 9.459375000614517859, 4.119189519843966529, -2.378215178124998275 ) ) ;
#16214=CARTESIAN_POINT ( 'NONE',  ( 34.99999999999999289, -2.499999999999999556, -3.499999999999999556 ) ) ;
#16227=CARTESIAN_POINT ( 'NONE',  ( 11.67187500061451821, 2.746126346562645981, -4.756430356249997438 ) ) ;
#16236=CARTESIAN_POINT ( 'NONE',  ( 12.03749999999999964, -2.886751345948130876, 4.999999999999996447 ) ) ;
#16244=CARTESIAN_POINT ( 'NONE',  ( 20.29687500061451289, 0.000000000000000000, 4.756430356249998326 ) ) ;
#16247=CARTESIAN_POINT ( 'NONE',  ( 14.04375000122903394, -2.886751345948125991, -5.000000000000000000 ) ) ;
#16249=CARTESIAN_POINT ( 'NONE',  ( 7.246875000614514839, 0.000000000000000000, 4.756430356249998326 ) ) ;
#16253=CARTESIAN_POINT ( 'NONE',  ( 21.50625000122903074, 0.000000000000000000, 4.999999999999998224 ) ) ;
#16263=CARTESIAN_POINT ( 'NONE',  ( 8.146875000614516082, 0.000000000000000000, 4.756430356249998326 ) ) ;
#16283=VECTOR ( 'NONE', #25048, 1000.000000000000000 ) ;
#16285=CARTESIAN_POINT ( 'NONE',  ( 17.10937500061451999, 4.119189519843966529, -2.378215178124998275 ) ) ;
#16317=CARTESIAN_POINT ( 'NONE',  ( 19.02187500061451786, 2.746126346562643317, 4.756430356249998326 ) ) ;
#16319=CARTESIAN_POINT ( 'NONE',  ( 34.99999999999999289, -2.499999999999999556, 3.499999999999999556 ) ) ;
#16323=CARTESIAN_POINT ( 'NONE',  ( 19.65000000000000213, 0.000000000000000000, 4.999999999999998224 ) ) ;
#16326=CARTESIAN_POINT ( 'NONE',  ( 26.74687500061451573, -4.119189519843965641, -2.378215178125001383 ) ) ;
#16327=CARTESIAN_POINT ( 'NONE',  ( 18.80625000122903501, 0.000000000000000000, 4.999999999999998224 ) ) ;
#16332=CARTESIAN_POINT ( 'NONE',  ( 26.33437500061451431, -2.746126346562642428, -4.756430356249999214 ) ) ;
#16334=CARTESIAN_POINT ( 'NONE',  ( 13.62187500061451750, -4.119189519843968306, 2.378215178124996054 ) ) ;
#16366=CARTESIAN_POINT ( 'NONE',  ( 24.08437500061451786, -4.119189519843968306, 2.378215178124996054 ) ) ;
#16368=CARTESIAN_POINT ( 'NONE',  ( 9.084375000614517859, 4.119189519843966529, 2.378215178124999607 ) ) ;
#16373=ORIENTED_EDGE ( 'NONE', *, *, #59244, .F. ) ;
#16377=EDGE_CURVE ( 'NONE', #14158, #53411, #26418, .T. ) ;
#16386=CARTESIAN_POINT ( 'NONE',  ( 18.84375000122903288, -2.886751345948129988, 4.999999999999997335 ) ) ;
#16403=CARTESIAN_POINT ( 'NONE',  ( 25.47187500061451715, -5.492252693125287522, -1.008910452111647106E-15 ) ) ;
#16409=CARTESIAN_POINT ( 'NONE',  ( 26.81250000000000000, 2.886751345948126879, 4.999999999999999112 ) ) ;
#16417=CARTESIAN_POINT ( 'NONE',  ( 11.98125000122903394, 4.330127018922191873, 2.499999999999999556 ) ) ;
#16419=CARTESIAN_POINT ( 'NONE',  ( 19.92187500061451289, -4.119189519843968306, 2.378215178124996054 ) ) ;
#16422=ORIENTED_EDGE ( 'NONE', *, *, #74, .F. ) ;
#16426=DIRECTION ( 'NONE',  ( -1.000000000000000000, -0.000000000000000000, -0.000000000000000000 ) ) ;
#16430=CARTESIAN_POINT ( 'NONE',  ( 11.74687500061451573, 0.000000000000000000, 4.756430356249998326 ) ) ;
#16433=( BOUNDED_CURVE ( )  B_SPLINE_CURVE ( 2, ( #12305, #34840, #40761, #67750, #57367, #56302, #29307 ),
 .UNSPECIFIED., .F., .F. ) 
 B_SPLINE_CURVE_WITH_KNOTS ( ( 3, 2, 2, 3 ),
 ( 0.8500000000000001998, 0.8533333333333336101, 0.8566666666666669094, 0.8600000000000002087 ),
 .UNSPECIFIED. ) 
 CURVE ( )  GEOMETRIC_REPRESENTATION_ITEM ( )  RATIONAL_B_SPLINE_CURVE ( ( 0.9999999999999911182, 0.8660254037844475894, 1.000000000000000000, 0.8660254037844387076, 1.000000000000000000, 0.8660254037844298258, 1.000000000000008882 ) ) 
 REPRESENTATION_ITEM ( '' )  );
#16436=ORIENTED_EDGE ( 'NONE', *, *, #1440, .F. ) ;
#16437=CARTESIAN_POINT ( 'NONE',  ( 21.09375000122903288, -2.886751345948130876, 4.999999999999996447 ) ) ;
#16454=CARTESIAN_POINT ( 'NONE',  ( 15.19687500061451857, -2.746126346562642428, -4.756430356249999214 ) ) ;
#16464=CARTESIAN_POINT ( 'NONE',  ( 13.03125000122903110, -4.330127018922194537, 2.499999999999995559 ) ) ;
#16472=CARTESIAN_POINT ( 'NONE',  ( 25.78125000122903288, 6.123233995736764310E-16, -4.999999999999998224 ) ) ;
#16477=CARTESIAN_POINT ( 'NONE',  ( -5.000000000000004441, 0.000000000000000000, 4.999999999999998224 ) ) ;
#16485=CARTESIAN_POINT ( 'NONE',  ( 23.98125000122903216, 6.123233995736764310E-16, -4.999999999999998224 ) ) ;
#16499=DIRECTION ( 'NONE',  ( -1.000000000000000000, -0.000000000000000000, -0.000000000000000000 ) ) ;
#16510=CARTESIAN_POINT ( 'NONE',  ( 34.99999999999999289, -2.499999999999999556, -3.499999999999999556 ) ) ;
#16514=CARTESIAN_POINT ( 'NONE',  ( 29.11875000122902790, 2.886751345948106007, 5.000000000000033751 ) ) ;
#16519=EDGE_CURVE ( 'NONE', #34969, #23351, #37001, .T. ) ;
#16523=CARTESIAN_POINT ( 'NONE',  ( 20.89687500061451786, -4.119189519843965641, -2.378215178125001383 ) ) ;
#16533=CARTESIAN_POINT ( 'NONE',  ( 11.51250000000000107, 2.886751345948126879, 4.999999999999999112 ) ) ;
#16540=CARTESIAN_POINT ( 'NONE',  ( 23.44687500061451502, 5.492252693125287522, 3.363034840372157021E-16 ) ) ;
#16543=CARTESIAN_POINT ( 'NONE',  ( 28.29375000122902506, -2.886751345948110004, 5.000000000000031974 ) ) ;
#16550=CARTESIAN_POINT ( 'NONE',  ( 12.00000000000000000, 0.000000000000000000, 4.999999999999998224 ) ) ;
#16563=CARTESIAN_POINT ( 'NONE',  ( 8.559375000614515727, 4.119189519843966529, -2.378215178124998275 ) ) ;
#16573=CARTESIAN_POINT ( 'NONE',  ( 45.00000000000000000, 0.000000000000000000, 0.000000000000000000 ) ) ;
#16584=CARTESIAN_POINT ( 'NONE',  ( 11.70937500061451608, 4.119189519843966529, -2.378215178124998275 ) ) ;
#16594=DIRECTION ( 'NONE',  ( -1.000000000000000000, -0.000000000000000000, -0.000000000000000000 ) ) ;
#16603=CARTESIAN_POINT ( 'NONE',  ( 19.13437500061451502, -2.746126346562642428, -4.756430356249999214 ) ) ;
#16606=CARTESIAN_POINT ( 'NONE',  ( 14.38125000122903252, -4.330127018922194537, 2.499999999999995559 ) ) ;
#16613=CARTESIAN_POINT ( 'NONE',  ( 21.75000000000000000, 4.330127018922192761, -2.499999999999997780 ) ) ;
#16614=DIRECTION ( 'NONE',  ( 0.000000000000000000, 0.000000000000000000, 1.000000000000000000 ) ) ;
#16621=CARTESIAN_POINT ( 'NONE',  ( 29.55937500061451573, -4.119189519843965641, -2.378215178125001383 ) ) ;
#16624=EDGE_CURVE ( 'NONE', #6077, #19923, #72580, .T. ) ;
#16628=DIRECTION ( 'NONE',  ( -1.000000000000000000, -0.000000000000000000, -0.000000000000000000 ) ) ;
#16632=ORIENTED_EDGE ( 'NONE', *, *, #3173, .F. ) ;
#16644=CARTESIAN_POINT ( 'NONE',  ( 16.73437500061451644, 4.119189519843966529, 2.378215178124999607 ) ) ;
#16675=CARTESIAN_POINT ( 'NONE',  ( 18.45937500061451431, 4.119189519843966529, -2.378215178124998275 ) ) ;
#16678=EDGE_CURVE ( 'NONE', #26340, #39358, #24271, .T. ) ;
#16682=CARTESIAN_POINT ( 'NONE',  ( 19.12500000000000000, 4.330127018922191873, 2.499999999999999556 ) ) ;
#16685=DIRECTION ( 'NONE',  ( -0.000000000000000000, -1.000000000000000000, 8.673617379884035472E-17 ) ) ;
#16686=CARTESIAN_POINT ( 'NONE',  ( 25.50937500061451502, 2.746126346562645981, -4.756430356249997438 ) ) ;
#16693=CARTESIAN_POINT ( 'NONE',  ( 28.02187500061451431, -4.119189519843968306, 2.378215178124996054 ) ) ;
#16695=CARTESIAN_POINT ( 'NONE',  ( 13.50937500061451679, 2.746126346562643317, 4.756430356249998326 ) ) ;
#16705=CARTESIAN_POINT ( 'NONE',  ( 20.71875000122903288, -5.773502691896255534, -1.060575238724906372E-15 ) ) ;
#16714=( BOUNDED_CURVE ( )  B_SPLINE_CURVE ( 2, ( #58392, #45532, #59125, #32169, #14435, #9269, #53599 ),
 .UNSPECIFIED., .F., .F. ) 
 B_SPLINE_CURVE_WITH_KNOTS ( ( 3, 2, 2, 3 ),
 ( 0.8800000000000000044, 0.8833333333333333037, 0.8866666666666667140, 0.8900000000000000133 ),
 .UNSPECIFIED. ) 
 CURVE ( )  GEOMETRIC_REPRESENTATION_ITEM ( )  RATIONAL_B_SPLINE_CURVE ( ( 1.000000000000000000, 0.8660254037844387076, 1.000000000000000000, 0.8660254037844387076, 1.000000000000000000, 0.8660254037844387076, 1.000000000000000000 ) ) 
 REPRESENTATION_ITEM ( '' )  );
#16731=CARTESIAN_POINT ( 'NONE',  ( 23.29687500061451644, -2.746126346562641984, -4.756430356249999214 ) ) ;
#16739=CARTESIAN_POINT ( 'NONE',  ( 19.98749999999999716, 5.773502691896255534, 3.535250795749688401E-16 ) ) ;
#16742=CARTESIAN_POINT ( 'NONE',  ( 14.98125000122903216, 6.123233995736764310E-16, -4.999999999999998224 ) ) ;
#16749=CARTESIAN_POINT ( 'NONE',  ( 18.80625000122903501, 0.000000000000000000, 4.999999999999998224 ) ) ;
#16751=CYLINDRICAL_SURFACE ( 'NONE', #43208, 4.999999999999998224 ) ;
#16765=CARTESIAN_POINT ( 'NONE',  ( 24.79687500061451999, 5.492252693125287522, 3.363034840372157021E-16 ) ) ;
#16771=CARTESIAN_POINT ( 'NONE',  ( 27.71250000000000568, 2.886751345948126879, 4.999999999999999112 ) ) ;
#16779=CARTESIAN_POINT ( 'NONE',  ( 12.09375000122903465, -2.886751345948129988, 4.999999999999997335 ) ) ;
#16780=CARTESIAN_POINT ( 'NONE',  ( 13.31250000000000178, 2.886751345948126879, 4.999999999999998224 ) ) ;
#16783=CARTESIAN_POINT ( 'NONE',  ( 20.85937500061451644, -5.492252693125287522, -1.008910452111647106E-15 ) ) ;
#16786=VERTEX_POINT ( 'NONE', #15685 ) ;
#16795=CARTESIAN_POINT ( 'NONE',  ( 12.38437500061451502, -2.746126346562642428, -4.756430356249999214 ) ) ;
#16803=LINE ( 'NONE', #56345, #2966 ) ;
#16805=CARTESIAN_POINT ( 'NONE',  ( 12.37500000000000000, 4.330127018922191873, 2.499999999999999556 ) ) ;
#16810=VERTEX_POINT ( 'NONE', #23046 ) ;
#16820=CARTESIAN_POINT ( 'NONE',  ( 16.28437500061452070, 4.119189519843966529, 2.378215178124999607 ) ) ;
#16838=CARTESIAN_POINT ( 'NONE',  ( 25.06875000122903074, 2.886751345948126879, 4.999999999999999112 ) ) ;
#16864=( BOUNDED_CURVE ( )  B_SPLINE_CURVE ( 2, ( #15375, #10577, #33104, #3950, #16464, #60435, #20918 ),
 .UNSPECIFIED., .F., .F. ) 
 B_SPLINE_CURVE_WITH_KNOTS ( ( 3, 2, 2, 3 ),
 ( 0.7299999999999999822, 0.7333333333333332815, 0.7366666666666666918, 0.7399999999999999911 ),
 .UNSPECIFIED. ) 
 CURVE ( )  GEOMETRIC_REPRESENTATION_ITEM ( )  RATIONAL_B_SPLINE_CURVE ( ( 1.000000000000000000, 0.8660254037844387076, 1.000000000000000000, 0.8660254037844387076, 1.000000000000000000, 0.8660254037844387076, 1.000000000000000000 ) ) 
 REPRESENTATION_ITEM ( '' )  );
#16884=CARTESIAN_POINT ( 'NONE',  ( 19.02187500061451431, -4.119189519843968306, 2.378215178124996054 ) ) ;
#16898=CARTESIAN_POINT ( 'NONE',  ( 22.27499999999999858, 4.330127018922191873, 2.499999999999999556 ) ) ;
#16899=CARTESIAN_POINT ( 'NONE',  ( 21.94687500061451857, -2.746126346562642428, -4.756430356249999214 ) ) ;
#16902=CARTESIAN_POINT ( 'NONE',  ( 45.00000000000000000, 0.000000000000000000, 0.000000000000000000 ) ) ;
#16909=CARTESIAN_POINT ( 'NONE',  ( -2.928932188134524939, -4.999999999999996447, -2.928932188134524939 ) ) ;
#16946=CARTESIAN_POINT ( 'NONE',  ( 10.88437500061451679, 4.119189519843966529, 2.378215178124999607 ) ) ;
#16947=DIRECTION ( 'NONE',  ( -1.000000000000000000, -0.000000000000000000, -0.000000000000000000 ) ) ;
#16955=CARTESIAN_POINT ( 'NONE',  ( 14.30625000122903145, 0.000000000000000000, 4.999999999999998224 ) ) ;
#16965=CARTESIAN_POINT ( 'NONE',  ( 17.48437500061451644, 5.492252693125287522, 3.363034840372157021E-16 ) ) ;
#16968=CARTESIAN_POINT ( 'NONE',  ( 13.51875000122903536, -5.773502691896255534, -1.060575238724906372E-15 ) ) ;
#16974=CARTESIAN_POINT ( 'NONE',  ( 21.07499999999999929, -4.330127018922194537, 2.499999999999995559 ) ) ;
#16976=CARTESIAN_POINT ( 'NONE',  ( 29.80312500061451431, 0.000000000000000000, 4.756430356249998326 ) ) ;
#16982=CARTESIAN_POINT ( 'NONE',  ( 29.25937500061451502, 4.119189519843966529, -2.378215178124998275 ) ) ;
#16985=CARTESIAN_POINT ( 'NONE',  ( 26.68125000122903145, 6.123233995736764310E-16, -4.999999999999998224 ) ) ;
#16988=CARTESIAN_POINT ( 'NONE',  ( 45.00000000000000000, 0.000000000000000000, 4.999999999999998224 ) ) ;
#16990=CYLINDRICAL_SURFACE ( 'NONE', #28859, 4.999999999999998224 ) ;
#16992=ORIENTED_EDGE ( 'NONE', *, *, #3406, .F. ) ;
#17004=CARTESIAN_POINT ( 'NONE',  ( 15.27187500061451786, 2.746126346562645981, -4.756430356249997438 ) ) ;
#17032=EDGE_CURVE ( 'NONE', #61955, #20756, #52114, .T. ) ;
#17036=CARTESIAN_POINT ( 'NONE',  ( 17.67187500061451644, 2.746126346562643317, 4.756430356249998326 ) ) ;
#17037=EDGE_CURVE ( 'NONE', #36109, #6463, #9164, .T. ) ;
#17040=EDGE_CURVE ( 'NONE', #65810, #41603, #3141, .T. ) ;
#17044=CARTESIAN_POINT ( 'NONE',  ( 20.13749999999999929, -2.886751345948129988, 4.999999999999997335 ) ) ;
#17049=CARTESIAN_POINT ( 'NONE',  ( 25.80937500061451573, -5.492252693125287522, -1.008910452111647106E-15 ) ) ;
#17056=CARTESIAN_POINT ( 'NONE',  ( 27.98437500061451644, -2.746126346562646425, 4.756430356249996549 ) ) ;
#17058=CARTESIAN_POINT ( 'NONE',  ( 10.92187500061451644, -4.119189519843968306, 2.378215178124996054 ) ) ;
#17063=CARTESIAN_POINT ( 'NONE',  ( 16.53750000000000142, -2.886751345948130876, 4.999999999999996447 ) ) ;
#17064=CARTESIAN_POINT ( 'NONE',  ( 20.99999999999999645, 0.000000000000000000, 4.999999999999998224 ) ) ;
#17068=CARTESIAN_POINT ( 'NONE',  ( 17.94375000122903074, -2.886751345948130876, 4.999999999999996447 ) ) ;
#17081=FACE_OUTER_BOUND ( 'NONE', #20364, .T. ) ;
#17093=CARTESIAN_POINT ( 'NONE',  ( 20.89687500061451786, -2.746126346562646425, 4.756430356249996549 ) ) ;
#17101=CARTESIAN_POINT ( 'NONE',  ( 19.91250000000000142, 2.886751345948129099, -4.999999999999997335 ) ) ;
#17108=VECTOR ( 'NONE', #1308, 1000.000000000000000 ) ;
#17113=CARTESIAN_POINT ( 'NONE',  ( 16.36875000122903145, 2.886751345948129099, -4.999999999999998224 ) ) ;
#17128=CARTESIAN_POINT ( 'NONE',  ( 26.40937500061451715, -4.119189519843965641, -2.378215178125001383 ) ) ;
#17134=CARTESIAN_POINT ( 'NONE',  ( 26.62500000000000000, 6.123233995736764310E-16, -4.999999999999998224 ) ) ;
#17135=AXIS2_PLACEMENT_3D ( 'NONE', #16018, #9753, #67018 ) ;
#17141=( BOUNDED_CURVE ( )  B_SPLINE_CURVE ( 2, ( #47714, #58418, #25173, #24809, #43195, #38004, #63970 ),
 .UNSPECIFIED., .F., .F. ) 
 B_SPLINE_CURVE_WITH_KNOTS ( ( 3, 2, 2, 3 ),
 ( 0.04000000000000007022, 0.04333333333333339726, 0.04666666666666672431, 0.05000000000000005135 ),
 .UNSPECIFIED. ) 
 CURVE ( )  GEOMETRIC_REPRESENTATION_ITEM ( )  RATIONAL_B_SPLINE_CURVE ( ( 0.9999999999999972244, 0.8660254037844414832, 1.000000000000000000, 0.8660254037844387076, 1.000000000000000000, 0.8660254037844367092, 1.000000000000001998 ) ) 
 REPRESENTATION_ITEM ( '' )  );
#17145=CARTESIAN_POINT ( 'NONE',  ( 12.31875000122903430, 2.886751345948129099, -4.999999999999998224 ) ) ;
#17149=CARTESIAN_POINT ( 'NONE',  ( 19.32187500061451857, 4.119189519843966529, 2.378215178124999607 ) ) ;
#17152=VERTEX_POINT ( 'NONE', #39166 ) ;
#17160=CARTESIAN_POINT ( 'NONE',  ( 12.42187500061451466, 5.824947211148865298E-16, -4.756430356249998326 ) ) ;
#17167=DIRECTION ( 'NONE',  ( -1.000000000000000000, -0.000000000000000000, -0.000000000000000000 ) ) ;
#17174=ORIENTED_EDGE ( 'NONE', *, *, #8310, .F. ) ;
#17177=EDGE_CURVE ( 'NONE', #23570, #35566, #71960, .T. ) ;
#17185=CARTESIAN_POINT ( 'NONE',  ( 12.72187500061451537, 2.746126346562643317, 4.756430356249998326 ) ) ;
#17202=CARTESIAN_POINT ( 'NONE',  ( 22.55625000122903145, -4.330127018922190985, -2.500000000000001332 ) ) ;
#17205=ORIENTED_EDGE ( 'NONE', *, *, #55050, .F. ) ;
#17215=VECTOR ( 'NONE', #5085, 1000.000000000000000 ) ;
#17227=LINE ( 'NONE', #11699, #38230 ) ;
#17243=ORIENTED_EDGE ( 'NONE', *, *, #72027, .T. ) ;
#17249=CARTESIAN_POINT ( 'NONE',  ( 18.45937500061451431, 2.746126346562643317, 4.756430356249998326 ) ) ;
#17264=CARTESIAN_POINT ( 'NONE',  ( 26.17500000000000071, 6.123233995736764310E-16, -4.999999999999998224 ) ) ;
#17265=CARTESIAN_POINT ( 'NONE',  ( 20.14687500061451786, -2.746126346562642428, -4.756430356249999214 ) ) ;
#17268=CARTESIAN_POINT ( 'NONE',  ( 12.71250000000000036, 2.886751345948073588, -5.000000000000094147 ) ) ;
#17276=EDGE_LOOP ( 'NONE', ( #61359, #68784, #50990, #14661 ) ) ;
#17283=DIRECTION ( 'NONE',  ( -1.000000000000000000, -0.000000000000000000, -0.000000000000000000 ) ) ;
#17288=CARTESIAN_POINT ( 'NONE',  ( 7.959375000614516971, -4.119189519843965641, -2.378215178125001383 ) ) ;
#17293=EDGE_CURVE ( 'NONE', #28919, #42612, #69157, .T. ) ;
#17298=DIRECTION ( 'NONE',  ( 0.000000000000000000, 0.000000000000000000, -1.000000000000000000 ) ) ;
#17311=CARTESIAN_POINT ( 'NONE',  ( 9.684375000614517504, -4.119189519843968306, 2.378215178124996054 ) ) ;
#17332=CARTESIAN_POINT ( 'NONE',  ( 18.19687500061451502, -4.119189519843965641, -2.378215178125001383 ) ) ;
#17335=CARTESIAN_POINT ( 'NONE',  ( 25.69687500061451502, 0.000000000000000000, 4.756430356249998326 ) ) ;
#17342=CARTESIAN_POINT ( 'NONE',  ( 21.86250000000000426, 2.886751345948126879, 4.999999999999998224 ) ) ;
#17349=CARTESIAN_POINT ( 'NONE',  ( 28.09687500061451360, -2.746126346562646425, 4.756430356249996549 ) ) ;
#17370=CARTESIAN_POINT ( 'NONE',  ( 14.07187500061451679, 2.746126346562643317, 4.756430356249998326 ) ) ;
#17401=CARTESIAN_POINT ( 'NONE',  ( 16.73437500061451644, 4.119189519843966529, 2.378215178124999607 ) ) ;
#17407=CARTESIAN_POINT ( 'NONE',  ( 19.98749999999999716, 5.773502691896255534, 3.535250795749688894E-16 ) ) ;
#17411=CARTESIAN_POINT ( 'NONE',  ( 24.57187500061451502, 5.824947211148865298E-16, -4.756430356249998326 ) ) ;
#17418=CARTESIAN_POINT ( 'NONE',  ( 24.19687500061451502, 4.119189519843966529, -2.378215178124998275 ) ) ;
#17420=CARTESIAN_POINT ( 'NONE',  ( 10.84687500061451715, 0.000000000000000000, 4.756430356249998326 ) ) ;
#17425=CARTESIAN_POINT ( 'NONE',  ( 8.118750001229031454, -5.773502691896255534, -1.060575238724906372E-15 ) ) ;
#17428=DIRECTION ( 'NONE',  ( 0.000000000000000000, 0.000000000000000000, 1.000000000000000000 ) ) ;
#17430=EDGE_LOOP ( 'NONE', ( #11648, #46745, #28254, #37515 ) ) ;
#17432=CARTESIAN_POINT ( 'NONE',  ( 13.43437500061451750, 5.492252693125287522, 3.363034840372157021E-16 ) ) ;
#17437=EDGE_CURVE ( 'NONE', #61419, #36820, #57589, .T. ) ;
#17443=LINE ( 'NONE', #33719, #6693 ) ;
#17453=CARTESIAN_POINT ( 'NONE',  ( 22.05937500061451573, 4.119189519843966529, -2.378215178124998275 ) ) ;
#17464=CARTESIAN_POINT ( 'NONE',  ( 15.16875000122903394, 2.886751345948182834, 4.999999999999902300 ) ) ;
#17472=CARTESIAN_POINT ( 'NONE',  ( 15.50625000122903430, 4.330127018922192761, -2.499999999999997780 ) ) ;
#17481=CARTESIAN_POINT ( 'NONE',  ( 22.34999999999999787, 0.000000000000000000, 4.999999999999998224 ) ) ;
#17484=VERTEX_POINT ( 'NONE', #29523 ) ;
#17488=CARTESIAN_POINT ( 'NONE',  ( 22.39687500061451075, -2.746126346562642428, -4.756430356249999214 ) ) ;
#17494=CARTESIAN_POINT ( 'NONE',  ( 27.11249999999999716, 2.886751345948129099, -4.999999999999998224 ) ) ;
#17502=CARTESIAN_POINT ( 'NONE',  ( 9.356250001229033941, 0.000000000000000000, 4.999999999999998224 ) ) ;
#17503=CARTESIAN_POINT ( 'NONE',  ( 9.000000000000001776, -4.330127018922190985, -2.500000000000001332 ) ) ;
#17506=CARTESIAN_POINT ( 'NONE',  ( 18.15937500061451360, -5.492252693125287522, -1.008910452111647106E-15 ) ) ;
#17512=CARTESIAN_POINT ( 'NONE',  ( 27.78750000000000142, -2.886751345948157965, 4.999999999999948486 ) ) ;
#17517=CARTESIAN_POINT ( 'NONE',  ( 13.92187500061451644, 4.119189519843966529, 2.378215178124999607 ) ) ;
#17537=CARTESIAN_POINT ( 'NONE',  ( 27.94687500061451502, 5.492252693125287522, 3.363034840372157021E-16 ) ) ;
#17540=CARTESIAN_POINT ( 'NONE',  ( 22.40625000122903288, 0.000000000000000000, 4.999999999999998224 ) ) ;
#17541=CARTESIAN_POINT ( 'NONE',  ( 11.63437500061451857, 5.824947211148865298E-16, -4.756430356249998326 ) ) ;
#17551=FACE_OUTER_BOUND ( 'NONE', #26812, .T. ) ;
#17558=CARTESIAN_POINT ( 'NONE',  ( 24.31875000122902719, -5.773502691896255534, -1.060575238724906372E-15 ) ) ;
#17585=EDGE_CURVE ( 'NONE', #58199, #68160, #8743, .T. ) ;
#17606=CARTESIAN_POINT ( 'NONE',  ( 19.28437500061451715, 5.492252693125287522, 3.363034840372157021E-16 ) ) ;
#17621=CARTESIAN_POINT ( 'NONE',  ( 45.00000000000000000, 0.000000000000000000, 4.999999999999998224 ) ) ;
#17623=CARTESIAN_POINT ( 'NONE',  ( 20.03437500061451715, -4.119189519843968306, 2.378215178124996054 ) ) ;
#17633=ORIENTED_EDGE ( 'NONE', *, *, #33344, .T. ) ;
#17643=CARTESIAN_POINT ( 'NONE',  ( 7.359375000614516438, 0.000000000000000000, 4.756430356249998326 ) ) ;
#17653=VERTEX_POINT ( 'NONE', #20977 ) ;
#17663=CARTESIAN_POINT ( 'NONE',  ( 9.909375000614517148, 4.119189519843966529, -2.378215178124998275 ) ) ;
#17684=CARTESIAN_POINT ( 'NONE',  ( 16.99687500061451573, 4.119189519843966529, -2.378215178124998275 ) ) ;
#17687=CARTESIAN_POINT ( 'NONE',  ( 27.15937500061451360, -5.492252693125287522, -1.008910452111647106E-15 ) ) ;
#17691=CARTESIAN_POINT ( 'NONE',  ( 28.68749999999999289, -2.886751345948110004, 5.000000000000031974 ) ) ;
#17701=CARTESIAN_POINT ( 'NONE',  ( 26.29687500061451644, -2.746126346562646425, 4.756430356249996549 ) ) ;
#17708=CARTESIAN_POINT ( 'NONE',  ( 14.51249999999999929, 2.886751345948073588, -5.000000000000094147 ) ) ;
#17720=CARTESIAN_POINT ( 'NONE',  ( 14.82187500061451502, 2.746126346562645981, -4.756430356249997438 ) ) ;
#17725=ORIENTED_EDGE ( 'NONE', *, *, #5848, .T. ) ;
#17734=CARTESIAN_POINT ( 'NONE',  ( 29.34375000122902932, -2.886751345948115777, -5.000000000000017764 ) ) ;
#17747=EDGE_LOOP ( 'NONE', ( #41863, #72371, #21386, #59473 ) ) ;
#17750=CARTESIAN_POINT ( 'NONE',  ( 16.80937500061451573, 0.000000000000000000, 4.756430356249998326 ) ) ;
#17756=CARTESIAN_POINT ( 'NONE',  ( 18.59999999999999787, 4.330127018922192761, -2.499999999999997780 ) ) ;
#17760=CARTESIAN_POINT ( 'NONE',  ( 26.37187500061451573, 5.824947211148865298E-16, -4.756430356249998326 ) ) ;
#17768=CARTESIAN_POINT ( 'NONE',  ( 24.60937500061451644, 2.746126346562645981, -4.756430356249997438 ) ) ;
#17770=CARTESIAN_POINT ( 'NONE',  ( 12.38437500061451502, -2.746126346562641984, -4.756430356249999214 ) ) ;
#17782=CARTESIAN_POINT ( 'NONE',  ( 11.18437500061451573, 5.492252693125287522, 3.363034840372157021E-16 ) ) ;
#17788=EDGE_CURVE ( 'NONE', #1656, #34631, #65313, .T. ) ;
#17800=CARTESIAN_POINT ( 'NONE',  ( 11.51249999999999929, 2.886751345948182834, 4.999999999999902300 ) ) ;
#17802=CARTESIAN_POINT ( 'NONE',  ( 21.30937500061451573, 0.000000000000000000, 4.756430356249998326 ) ) ;
#17809=ORIENTED_EDGE ( 'NONE', *, *, #71833, .T. ) ;
#17819=CARTESIAN_POINT ( 'NONE',  ( 28.53749999999999787, 5.773502691896255534, 3.535250795749688401E-16 ) ) ;
#17822=CARTESIAN_POINT ( 'NONE',  ( 16.03125000122903288, 4.330127018922191873, 2.499999999999999556 ) ) ;
#17824=DIRECTION ( 'NONE',  ( -1.000000000000000000, -0.000000000000000000, -0.000000000000000000 ) ) ;
#17834=ORIENTED_EDGE ( 'NONE', *, *, #9426, .T. ) ;
#17838=CARTESIAN_POINT ( 'NONE',  ( 23.37187500061451573, 2.746126346562645981, -4.756430356249997438 ) ) ;
#17844=CARTESIAN_POINT ( 'NONE',  ( 23.51249999999999574, 2.886751345948129099, -4.999999999999998224 ) ) ;
#17845=EDGE_CURVE ( 'NONE', #54880, #36109, #44143, .T. ) ;
#17850=FACE_OUTER_BOUND ( 'NONE', #7257, .T. ) ;
#17853=EDGE_CURVE ( 'NONE', #24521, #12847, #63953, .T. ) ;
#17856=CARTESIAN_POINT ( 'NONE',  ( 8.718750001229032875, 2.886751345948129099, -4.999999999999998224 ) ) ;
#17860=CARTESIAN_POINT ( 'NONE',  ( 19.05937500061451573, -5.492252693125287522, -1.008910452111647106E-15 ) ) ;
#17871=CARTESIAN_POINT ( 'NONE',  ( 10.99687500061451573, -4.119189519843965641, -2.378215178125001383 ) ) ;
#17884=CARTESIAN_POINT ( 'NONE',  ( 11.66249999999999964, -5.773502691896255534, -1.060575238724906372E-15 ) ) ;
#17893=CARTESIAN_POINT ( 'NONE',  ( 28.20937500061451786, -4.119189519843965641, -2.378215178125001383 ) ) ;
#17896=CARTESIAN_POINT ( 'NONE',  ( 28.43437500061451573, -2.746126346562646425, 4.756430356249996549 ) ) ;
#17897=CARTESIAN_POINT ( 'NONE',  ( 12.90937500061451537, -4.119189519843965641, -2.378215178125001383 ) ) ;
#17905=CYLINDRICAL_SURFACE ( 'NONE', #46620, 4.999999999999998224 ) ;
#17912=CARTESIAN_POINT ( 'NONE',  ( 24.39375000122903003, -2.886751345948125991, -5.000000000000000000 ) ) ;
#17915=ORIENTED_EDGE ( 'NONE', *, *, #49500, .F. ) ;
#17933=( BOUNDED_CURVE ( )  B_SPLINE_CURVE ( 2, ( #35173, #17800, #6742, #47349, #40360, #58052, #41448 ),
 .UNSPECIFIED., .F., .F. ) 
 B_SPLINE_CURVE_WITH_KNOTS ( ( 3, 2, 2, 3 ),
 ( 0.8200000000000000622, 0.8233333333333334725, 0.8266666666666667718, 0.8300000000000000711 ),
 .UNSPECIFIED. ) 
 CURVE ( )  GEOMETRIC_REPRESENTATION_ITEM ( )  RATIONAL_B_SPLINE_CURVE ( ( 0.9999999999999955591, 0.8660254037844431485, 1.000000000000000000, 0.8660254037844387076, 1.000000000000000000, 0.8660254037844342667, 1.000000000000004441 ) ) 
 REPRESENTATION_ITEM ( '' )  );
#17954=LINE ( 'NONE', #70031, #67950 ) ;
#17963=CARTESIAN_POINT ( 'NONE',  ( 19.20937500061451786, 2.746126346562645981, -4.756430356249997438 ) ) ;
#17982=CARTESIAN_POINT ( 'NONE',  ( 20.22187500061451715, 2.746126346562645981, -4.756430356249997438 ) ) ;
#17993=DIRECTION ( 'NONE',  ( -1.000000000000000000, -0.000000000000000000, -0.000000000000000000 ) ) ;
#17998=CARTESIAN_POINT ( 'NONE',  ( 45.00000000000000000, 6.123233995736764310E-16, -4.999999999999998224 ) ) ;
#18005=CARTESIAN_POINT ( 'NONE',  ( 45.00000000000000000, 0.000000000000000000, 0.000000000000000000 ) ) ;
#18012=DIRECTION ( 'NONE',  ( 0.000000000000000000, 0.000000000000000000, 1.000000000000000000 ) ) ;
#18029=CARTESIAN_POINT ( 'NONE',  ( 8.484375000614518214, 5.824947211148865298E-16, -4.756430356249998326 ) ) ;
#18047=CARTESIAN_POINT ( 'NONE',  ( 18.45937500061451431, 2.746126346562643317, 4.756430356249998326 ) ) ;
#18050=CARTESIAN_POINT ( 'NONE',  ( 25.73437500061451644, -2.746126346562646425, 4.756430356249996549 ) ) ;
#18064=CARTESIAN_POINT ( 'NONE',  ( 26.40937500061451715, -4.119189519843965641, -2.378215178125001383 ) ) ;
#18082=CARTESIAN_POINT ( 'NONE',  ( 14.25937500061451679, -4.119189519843965641, -2.378215178125001383 ) ) ;
#18111=CARTESIAN_POINT ( 'NONE',  ( 15.90937500061451892, 0.000000000000000000, 4.756430356249998326 ) ) ;
#18118=CARTESIAN_POINT ( 'NONE',  ( 17.17500000000000071, 6.123233995736764310E-16, -4.999999999999998224 ) ) ;
#18122=CARTESIAN_POINT ( 'NONE',  ( 23.37187500061451573, 4.119189519843966529, 2.378215178124999607 ) ) ;
#18128=CARTESIAN_POINT ( 'NONE',  ( 24.94687500061451502, -4.119189519843965641, -2.378215178125001383 ) ) ;
#18130=CARTESIAN_POINT ( 'NONE',  ( 12.34687500061451537, -4.119189519843965641, -2.378215178125001383 ) ) ;
#18135=CARTESIAN_POINT ( 'NONE',  ( 16.61250000000000071, -5.773502691896255534, -1.060575238724906372E-15 ) ) ;
#18138=CARTESIAN_POINT ( 'NONE',  ( 26.38125000122903430, 4.330127018922191873, 2.499999999999999556 ) ) ;
#18139=CARTESIAN_POINT ( 'NONE',  ( 20.83125000122903359, 6.123233995736764310E-16, -4.999999999999998224 ) ) ;
#18142=CARTESIAN_POINT ( 'NONE',  ( 12.68437500061451750, -2.746126346562646425, 4.756430356249996549 ) ) ;
#18160=CARTESIAN_POINT ( 'NONE',  ( 12.20625000122903181, -4.330127018922190985, -2.500000000000001332 ) ) ;
#18162=CARTESIAN_POINT ( 'NONE',  ( 21.87187500061451573, -5.492252693125287522, -1.008910452111647106E-15 ) ) ;
#18169=VERTEX_POINT ( 'NONE', #73056 ) ;
#18180=CARTESIAN_POINT ( 'NONE',  ( 21.37499999999999645, 4.330127018922191873, 2.499999999999999556 ) ) ;
#18183=CARTESIAN_POINT ( 'NONE',  ( 17.19375000122903430, -2.886751345948125991, -5.000000000000000000 ) ) ;
#18198=CARTESIAN_POINT ( 'NONE',  ( 22.77187500061451786, -5.492252693125287522, -1.008910452111647106E-15 ) ) ;
#18202=( BOUNDED_CURVE ( )  B_SPLINE_CURVE ( 2, ( #31046, #69134, #24042, #31421, #53214, #2254, #58376 ),
 .UNSPECIFIED., .F., .F. ) 
 B_SPLINE_CURVE_WITH_KNOTS ( ( 3, 2, 2, 3 ),
 ( 0.1499999999999999944, 0.1533333333333333215, 0.1566666666666666485, 0.1599999999999999756 ),
 .UNSPECIFIED. ) 
 CURVE ( )  GEOMETRIC_REPRESENTATION_ITEM ( )  RATIONAL_B_SPLINE_CURVE ( ( 1.000000000000000000, 0.8660254037844387076, 1.000000000000000000, 0.8660254037844387076, 1.000000000000000000, 0.8660254037844398178, 0.9999999999999988898 ) ) 
 REPRESENTATION_ITEM ( '' )  );
#18205=CARTESIAN_POINT ( 'NONE',  ( 25.01249999999999929, 2.886751345948126879, 4.999999999999999112 ) ) ;
#18213=CARTESIAN_POINT ( 'NONE',  ( 10.36875000122903323, -5.773502691896255534, -1.060575238724906372E-15 ) ) ;
#18215=CARTESIAN_POINT ( 'NONE',  ( 18.72187500061451360, 5.824947211148865298E-16, -4.756430356249998326 ) ) ;
#18222=CARTESIAN_POINT ( 'NONE',  ( 20.36249999999999361, 2.886751345948073588, -5.000000000000094147 ) ) ;
#18226=CARTESIAN_POINT ( 'NONE',  ( 10.47187500061451715, -4.119189519843968306, 2.378215178124996054 ) ) ;
#18232=AXIS2_PLACEMENT_3D ( 'NONE', #49001, #59697, #53808 ) ;
#18240=CARTESIAN_POINT ( 'NONE',  ( 9.487500000000000711, -2.886751345948125991, -5.000000000000000000 ) ) ;
#18249=CARTESIAN_POINT ( 'NONE',  ( 29.29687500061450933, 5.492252693125287522, 3.363034840372157021E-16 ) ) ;
#18251=CARTESIAN_POINT ( 'NONE',  ( 28.05937500061451217, -5.492252693125287522, -1.008910452111647106E-15 ) ) ;
#18252=CARTESIAN_POINT ( 'NONE',  ( 12.23437500061451821, 4.119189519843966529, 2.378215178124999607 ) ) ;
#18269=CARTESIAN_POINT ( 'NONE',  ( 23.41875000122903216, -5.773502691896255534, -1.060575238724906372E-15 ) ) ;
#18276=CARTESIAN_POINT ( 'NONE',  ( 25.44375000122903074, 5.773502691896255534, 3.535250795749688401E-16 ) ) ;
#18297=CARTESIAN_POINT ( 'NONE',  ( 22.40625000122903288, 0.000000000000000000, 4.999999999999998224 ) ) ;
#18322=CARTESIAN_POINT ( 'NONE',  ( 19.24687500061451573, 4.119189519843966529, -2.378215178124998275 ) ) ;
#18332=ORIENTED_EDGE ( 'NONE', *, *, #67527, .T. ) ;
#18340=CARTESIAN_POINT ( 'NONE',  ( 19.43437500061451928, 4.119189519843966529, 2.378215178124999607 ) ) ;
#18354=ORIENTED_EDGE ( 'NONE', *, *, #44062, .T. ) ;
#18365=DIRECTION ( 'NONE',  ( -1.000000000000000000, -0.000000000000000000, -0.000000000000000000 ) ) ;
#18370=( BOUNDED_CURVE ( )  B_SPLINE_CURVE ( 2, ( #38662, #32377, #60438, #27211, #54917, #49746, #59711 ),
 .UNSPECIFIED., .F., .F. ) 
 B_SPLINE_CURVE_WITH_KNOTS ( ( 3, 2, 2, 3 ),
 ( 0.1900000000000000855, 0.1933333333333333848, 0.1966666666666667118, 0.2000000000000000389 ),
 .UNSPECIFIED. ) 
 CURVE ( )  GEOMETRIC_REPRESENTATION_ITEM ( )  RATIONAL_B_SPLINE_CURVE ( ( 0.9999999999999966693, 0.8660254037844420383, 1.000000000000000000, 0.8660254037844387076, 1.000000000000000000, 0.8660254037844375974, 1.000000000000001110 ) ) 
 REPRESENTATION_ITEM ( '' )  );
#18371=EDGE_CURVE ( 'NONE', #38724, #1846, #55340, .T. ) ;
#18378=VERTEX_POINT ( 'NONE', #28349 ) ;
#18389=CARTESIAN_POINT ( 'NONE',  ( 8.034375000614518925, 5.824947211148865298E-16, -4.756430356249998326 ) ) ;
#18391=CARTESIAN_POINT ( 'NONE',  ( 20.15625000122903288, 0.000000000000000000, 4.999999999999998224 ) ) ;
#18400=CARTESIAN_POINT ( 'NONE',  ( 45.00000000000000000, 0.000000000000000000, 4.999999999999998224 ) ) ;
#18410=CARTESIAN_POINT ( 'NONE',  ( 18.87187500061451573, 4.119189519843966529, 2.378215178124999607 ) ) ;
#18413=CARTESIAN_POINT ( 'NONE',  ( 25.99687500061451573, 4.119189519843966529, -2.378215178124998275 ) ) ;
#18428=CARTESIAN_POINT ( 'NONE',  ( 26.67187500061451644, 2.746126346562643317, 4.756430356249998326 ) ) ;
#18435=( BOUNDED_CURVE ( )  B_SPLINE_CURVE ( 2, ( #56029, #66758, #66382, #54935, #50127, #44597, #49397 ),
 .UNSPECIFIED., .F., .F. ) 
 B_SPLINE_CURVE_WITH_KNOTS ( ( 3, 2, 2, 3 ),
 ( 0.7000000000000001776, 0.7033333333333335879, 0.7066666666666668872, 0.7100000000000001865 ),
 .UNSPECIFIED. ) 
 CURVE ( )  GEOMETRIC_REPRESENTATION_ITEM ( )  RATIONAL_B_SPLINE_CURVE ( ( 0.9999999999999911182, 0.8660254037844475894, 1.000000000000000000, 0.8660254037844387076, 1.000000000000000000, 0.8660254037844298258, 1.000000000000008882 ) ) 
 REPRESENTATION_ITEM ( '' )  );
#18448=CARTESIAN_POINT ( 'NONE',  ( 14.70937500061451786, -4.119189519843965641, -2.378215178125001383 ) ) ;
#18479=CARTESIAN_POINT ( 'NONE',  ( 17.25937500061451502, 0.000000000000000000, 4.756430356249998326 ) ) ;
#18485=CARTESIAN_POINT ( 'NONE',  ( 16.94999999999999929, 0.000000000000000000, 4.999999999999998224 ) ) ;
#18489=CARTESIAN_POINT ( 'NONE',  ( 22.77187500061451431, 5.824947211148865298E-16, -4.756430356249998326 ) ) ;
#18490=ORIENTED_EDGE ( 'NONE', *, *, #62721, .F. ) ;
#18491=EDGE_CURVE ( 'NONE', #10316, #70443, #62689, .T. ) ;
#18497=CARTESIAN_POINT ( 'NONE',  ( 24.83437500061451075, -2.746126346562646425, 4.756430356249996549 ) ) ;
#18499=CARTESIAN_POINT ( 'NONE',  ( 10.13437500061451679, -2.746126346562641984, -4.756430356249999214 ) ) ;
#18507=CARTESIAN_POINT ( 'NONE',  ( 26.34375000122902577, 5.773502691896255534, 3.535250795749688401E-16 ) ) ;
#18511=CARTESIAN_POINT ( 'NONE',  ( 12.72187500061451537, -4.119189519843968306, 2.378215178124996054 ) ) ;
#18519=CARTESIAN_POINT ( 'NONE',  ( 23.47499999999999787, 6.123233995736764310E-16, -4.999999999999998224 ) ) ;
#18528=CARTESIAN_POINT ( 'NONE',  ( 29.96249999999999858, 2.886751345948126879, 4.999999999999998224 ) ) ;
#18531=CARTESIAN_POINT ( 'NONE',  ( 21.19687500061451502, 5.492252693125287522, 3.363034840372157021E-16 ) ) ;
#18548=CARTESIAN_POINT ( 'NONE',  ( 28.42499999999999716, 6.123233995736764310E-16, -4.999999999999998224 ) ) ;
#18552=CARTESIAN_POINT ( 'NONE',  ( 9.487499999999997158, -2.886751345948126435, -5.000000000000000000 ) ) ;
#18566=CARTESIAN_POINT ( 'NONE',  ( 24.45937500061451786, 0.000000000000000000, 4.756430356249998326 ) ) ;
#18569=CARTESIAN_POINT ( 'NONE',  ( 29.13749999999999929, -2.886751345948095349, 5.000000000000058620 ) ) ;
#18572=CARTESIAN_POINT ( 'NONE',  ( 25.42500000000000071, 4.330127018922191873, 2.499999999999999556 ) ) ;
#18576=VECTOR ( 'NONE', #68259, 1000.000000000000000 ) ;
#18578=CARTESIAN_POINT ( 'NONE',  ( 24.37500000000000000, 6.123233995736764310E-16, -4.999999999999998224 ) ) ;
#18580=( BOUNDED_CURVE ( )  B_SPLINE_CURVE ( 2, ( #11510, #45855, #51035, #44785, #5245, #27787, #432 ),
 .UNSPECIFIED., .F., .F. ) 
 B_SPLINE_CURVE_WITH_KNOTS ( ( 3, 2, 2, 3 ),
 ( 0.6600000000000000311, 0.6633333333333333304, 0.6666666666666666297, 0.6700000000000000400 ),
 .UNSPECIFIED. ) 
 CURVE ( )  GEOMETRIC_REPRESENTATION_ITEM ( )  RATIONAL_B_SPLINE_CURVE ( ( 1.000000000000000000, 0.8660254037844387076, 1.000000000000000000, 0.8660254037844387076, 1.000000000000000000, 0.8660254037844387076, 1.000000000000000000 ) ) 
 REPRESENTATION_ITEM ( '' )  );
#18581=CARTESIAN_POINT ( 'NONE',  ( 15.22500000000000142, -4.330127018922194537, 2.499999999999995559 ) ) ;
#18583=CARTESIAN_POINT ( 'NONE',  ( 9.656250001229032875, 4.330127018922192761, -2.499999999999997780 ) ) ;
#18584=CARTESIAN_POINT ( 'NONE',  ( 8.962500000000002132, -5.773502691896255534, -1.060575238724906372E-15 ) ) ;
#18586=CARTESIAN_POINT ( 'NONE',  ( 19.43437500061451573, -2.746126346562646425, 4.756430356249996549 ) ) ;
#18598=CARTESIAN_POINT ( 'NONE',  ( 10.28437500061451892, 5.492252693125287522, 3.363034840372157021E-16 ) ) ;
#18608=CARTESIAN_POINT ( 'NONE',  ( 28.20937500061451075, 2.746126346562645981, -4.756430356249997438 ) ) ;
#18611=CARTESIAN_POINT ( 'NONE',  ( 9.825000000000001066, -4.330127018922194537, 2.499999999999995559 ) ) ;
#18619=CARTESIAN_POINT ( 'NONE',  ( 29.37187500061451928, 2.746126346562643317, 4.756430356249998326 ) ) ;
#18621=CARTESIAN_POINT ( 'NONE',  ( 28.77187500061451431, 4.119189519843966529, 2.378215178124999607 ) ) ;
#18622=CARTESIAN_POINT ( 'NONE',  ( 10.47187500061451715, 2.746126346562643317, 4.756430356249998326 ) ) ;
#18638=CARTESIAN_POINT ( 'NONE',  ( 23.83125000122903359, -4.330127018922194537, 2.499999999999995559 ) ) ;
#18663=LINE ( 'NONE', #57474, #12330 ) ;
#18667=CARTESIAN_POINT ( 'NONE',  ( 23.88749999999999929, -2.886751345948153968, -4.999999999999952038 ) ) ;
#18678=CARTESIAN_POINT ( 'NONE',  ( 27.07499999999999929, 6.123233995736764310E-16, -4.999999999999998224 ) ) ;
#18681=ORIENTED_EDGE ( 'NONE', *, *, #59515, .F. ) ;
#18687=CARTESIAN_POINT ( 'NONE',  ( 15.57187500061451679, 5.824947211148865298E-16, -4.756430356249998326 ) ) ;
#18703=CARTESIAN_POINT ( 'NONE',  ( 27.13125000122903430, 6.123233995736764310E-16, -4.999999999999998224 ) ) ;
#18706=CARTESIAN_POINT ( 'NONE',  ( 20.63437500061451857, 5.824947211148865298E-16, -4.756430356249998326 ) ) ;
#18715=EDGE_CURVE ( 'NONE', #58973, #24462, #28593, .T. ) ;
#18718=DIRECTION ( 'NONE',  ( -1.000000000000000000, -0.000000000000000000, -0.000000000000000000 ) ) ;
#18719=ORIENTED_EDGE ( 'NONE', *, *, #45399, .T. ) ;
#18721=DIRECTION ( 'NONE',  ( 0.000000000000000000, 0.000000000000000000, 1.000000000000000000 ) ) ;
#18725=CARTESIAN_POINT ( 'NONE',  ( 45.00000000000000000, 0.000000000000000000, 4.999999999999998224 ) ) ;
#18727=CARTESIAN_POINT ( 'NONE',  ( 8.437500000000000000, -2.886751345948130876, 4.999999999999996447 ) ) ;
#18728=CARTESIAN_POINT ( 'NONE',  ( 45.00000000000000000, 6.123233995736764310E-16, -4.999999999999998224 ) ) ;
#18738=VERTEX_POINT ( 'NONE', #70113 ) ;
#18750=CARTESIAN_POINT ( 'NONE',  ( 29.73750000000000071, -2.886751345948125991, -5.000000000000000000 ) ) ;
#18768=CARTESIAN_POINT ( 'NONE',  ( 14.85937500061451999, 2.746126346562643317, 4.756430356249998326 ) ) ;
#18771=CARTESIAN_POINT ( 'NONE',  ( 26.59687500061451360, 0.000000000000000000, 4.756430356249998326 ) ) ;
#18778=ADVANCED_FACE ( 'NONE', ( #40594 ), #2165, .T. ) ;
#18779=CARTESIAN_POINT ( 'NONE',  ( 21.95625000122903003, 0.000000000000000000, 4.999999999999998224 ) ) ;
#18787=CARTESIAN_POINT ( 'NONE',  ( 28.17187500061451644, -5.492252693125287522, -1.008910452111647106E-15 ) ) ;
#18806=CARTESIAN_POINT ( 'NONE',  ( 11.14687500061451608, -2.746126346562641984, -4.756430356249999214 ) ) ;
#18812=ADVANCED_FACE ( 'NONE', ( #53121 ), #2519, .T. ) ;
#18837=CARTESIAN_POINT ( 'NONE',  ( 15.57187500061451679, -5.492252693125287522, -1.008910452111647106E-15 ) ) ;
#18845=CARTESIAN_POINT ( 'NONE',  ( 18.41250000000000142, -5.773502691896255534, -1.060575238724906372E-15 ) ) ;
#18849=CARTESIAN_POINT ( 'NONE',  ( 22.58437500061451786, -2.746126346562646425, 4.756430356249996549 ) ) ;
#18855=( BOUNDED_CURVE ( )  B_SPLINE_CURVE ( 2, ( #66213, #55865, #71768, #49961, #72485, #21871, #27796 ),
 .UNSPECIFIED., .F., .F. ) 
 B_SPLINE_CURVE_WITH_KNOTS ( ( 3, 2, 2, 3 ),
 ( 0.6700000000000000400, 0.6733333333333333393, 0.6766666666666667496, 0.6800000000000001599 ),
 .UNSPECIFIED. ) 
 CURVE ( )  GEOMETRIC_REPRESENTATION_ITEM ( )  RATIONAL_B_SPLINE_CURVE ( ( 1.000000000000000000, 0.8660254037844387076, 1.000000000000000000, 0.8660254037844387076, 1.000000000000000000, 0.8660254037844342667, 1.000000000000004441 ) ) 
 REPRESENTATION_ITEM ( '' )  );
#18857=CARTESIAN_POINT ( 'NONE',  ( 25.80937500061451217, -5.492252693125287522, -1.008910452111647106E-15 ) ) ;
#18859=CARTESIAN_POINT ( 'NONE',  ( 8.709375000614517859, -5.492252693125287522, -1.008910452111647106E-15 ) ) ;
#18867=CARTESIAN_POINT ( 'NONE',  ( 19.38750000000000284, -2.886751345948209480, -4.999999999999856115 ) ) ;
#18870=CARTESIAN_POINT ( 'NONE',  ( 11.97187500061451537, 5.824947211148865298E-16, -4.756430356249998326 ) ) ;
#18885=CARTESIAN_POINT ( 'NONE',  ( 29.88749999999999929, 5.773502691896255534, 3.535250795749688401E-16 ) ) ;
#18888=CARTESIAN_POINT ( 'NONE',  ( 18.98437500061451644, 4.119189519843966529, 2.378215178124999607 ) ) ;
#18910=LINE ( 'NONE', #57720, #33762 ) ;
#18911=ADVANCED_FACE ( 'NONE', ( #42047 ), #23949, .T. ) ;
#18924=CARTESIAN_POINT ( 'NONE',  ( 23.52187500061451786, 2.746126346562643317, 4.756430356249998326 ) ) ;
#18930=CARTESIAN_POINT ( 'NONE',  ( 23.77499999999999858, -4.330127018922194537, 2.499999999999995559 ) ) ;
#18935=CYLINDRICAL_SURFACE ( 'NONE', #29255, 4.999999999999998224 ) ;
#18940=CARTESIAN_POINT ( 'NONE',  ( 8.231250001229033941, 6.123233995736764310E-16, -4.999999999999998224 ) ) ;
#18943=CARTESIAN_POINT ( 'NONE',  ( 16.50937500061451502, 2.746126346562645981, -4.756430356249997438 ) ) ;
#18946=ORIENTED_EDGE ( 'NONE', *, *, #36053, .T. ) ;
#18955=CARTESIAN_POINT ( 'NONE',  ( 11.14687500061451608, 4.119189519843966529, -2.378215178124998275 ) ) ;
#18956=ORIENTED_EDGE ( 'NONE', *, *, #72743, .F. ) ;
#18962=CARTESIAN_POINT ( 'NONE',  ( 10.35000000000000142, -4.330127018922190985, -2.500000000000001332 ) ) ;
#18964=CARTESIAN_POINT ( 'NONE',  ( 8.981250001229033941, -4.330127018922194537, 2.499999999999995559 ) ) ;
#18966=CARTESIAN_POINT ( 'NONE',  ( 29.29687500061451644, 0.000000000000000000, 4.756430356249998326 ) ) ;
#18969=CARTESIAN_POINT ( 'NONE',  ( 9.074999999999999289, 6.123233995736764310E-16, -4.999999999999998224 ) ) ;
#18977=CARTESIAN_POINT ( 'NONE',  ( 28.02187500061451431, 2.746126346562643317, 4.756430356249998326 ) ) ;
#18979=CARTESIAN_POINT ( 'NONE',  ( 26.89687500061451431, 4.119189519843966529, -2.378215178124998275 ) ) ;
#18980=CARTESIAN_POINT ( 'NONE',  ( 11.55937500061451928, -4.119189519843965641, -2.378215178125001383 ) ) ;
#18994=CARTESIAN_POINT ( 'NONE',  ( 22.10625000122903216, -4.330127018922190985, -2.500000000000001332 ) ) ;
#18996=CARTESIAN_POINT ( 'NONE',  ( 45.00000000000000000, 6.123233995736764310E-16, -4.999999999999998224 ) ) ;
#19039=DIRECTION ( 'NONE',  ( 1.000000000000000000, -0.000000000000000000, -0.000000000000000000 ) ) ;
#19049=CARTESIAN_POINT ( 'NONE',  ( 15.98437500061451644, -2.746126346562642428, -4.756430356249999214 ) ) ;
#19069=CARTESIAN_POINT ( 'NONE',  ( 18.23437500061451999, -4.119189519843968306, 2.378215178124996054 ) ) ;
#19081=DIRECTION ( 'NONE',  ( 0.000000000000000000, 0.000000000000000000, 1.000000000000000000 ) ) ;
#19082=ORIENTED_EDGE ( 'NONE', *, *, #41965, .F. ) ;
#19088=CARTESIAN_POINT ( 'NONE',  ( 29.56875000122903074, 2.886751345948126879, 4.999999999999999112 ) ) ;
#19101=EDGE_LOOP ( 'NONE', ( #49490, #13262, #30473, #69462 ) ) ;
#19112=CARTESIAN_POINT ( 'NONE',  ( 45.00000000000000000, 0.000000000000000000, 0.000000000000000000 ) ) ;
#19113=CARTESIAN_POINT ( 'NONE',  ( 28.49999999999999645, 4.330127018922192761, -2.499999999999997780 ) ) ;
#19119=EDGE_CURVE ( 'NONE', #33154, #60311, #5940, .T. ) ;
#19120=CARTESIAN_POINT ( 'NONE',  ( 27.52500000000000213, 6.123233995736764310E-16, -4.999999999999998224 ) ) ;
#19132=CARTESIAN_POINT ( 'NONE',  ( 16.09687500061451715, 4.119189519843966529, -2.378215178124998275 ) ) ;
#19135=CARTESIAN_POINT ( 'NONE',  ( 22.80937500061451573, 2.746126346562645981, -4.756430356249997438 ) ) ;
#19143=CARTESIAN_POINT ( 'NONE',  ( 34.99999999999999289, 0.000000000000000000, 0.000000000000000000 ) ) ;
#19150=CARTESIAN_POINT ( 'NONE',  ( 24.19687500061451857, -2.746126346562642428, -4.756430356249999214 ) ) ;
#19169=CARTESIAN_POINT ( 'NONE',  ( 12.49687500061451573, -2.746126346562641984, -4.756430356249999214 ) ) ;
#19182=CARTESIAN_POINT ( 'NONE',  ( 23.45625000122903359, -4.330127018922190985, -2.500000000000001332 ) ) ;
#19183=ORIENTED_EDGE ( 'NONE', *, *, #72365, .F. ) ;
#19195=ORIENTED_EDGE ( 'NONE', *, *, #65590, .F. ) ;
#19198=CARTESIAN_POINT ( 'NONE',  ( 14.22187500061451537, -5.492252693125287522, -1.008910452111647106E-15 ) ) ;
#19205=CARTESIAN_POINT ( 'NONE',  ( 17.28750000000000142, 5.773502691896255534, 3.535250795749688894E-16 ) ) ;
#19209=CARTESIAN_POINT ( 'NONE',  ( 22.20937500061451786, -5.492252693125287522, -1.008910452111647106E-15 ) ) ;
#19210=VERTEX_POINT ( 'NONE', #50055 ) ;
#19218=CARTESIAN_POINT ( 'NONE',  ( 21.57187500061451146, 4.119189519843966529, 2.378215178124999607 ) ) ;
#19220=CARTESIAN_POINT ( 'NONE',  ( 8.184375000614515727, -2.746126346562646425, 4.756430356249996549 ) ) ;
#19230=CARTESIAN_POINT ( 'NONE',  ( 11.14687500061451608, 4.119189519843966529, -2.378215178124998275 ) ) ;
#19250=CARTESIAN_POINT ( 'NONE',  ( 19.09687500061451360, -2.746126346562646425, 4.756430356249996549 ) ) ;
#19288=CARTESIAN_POINT ( 'NONE',  ( 21.19687500061451502, 5.492252693125287522, 3.363034840372157021E-16 ) ) ;
#19294=CARTESIAN_POINT ( 'NONE',  ( 23.58749999999999858, 5.773502691896255534, 3.535250795749688894E-16 ) ) ;
#19300=FACE_OUTER_BOUND ( 'NONE', #34060, .T. ) ;
#19305=CARTESIAN_POINT ( 'NONE',  ( 29.18437500061451217, 5.492252693125287522, 3.363034840372157021E-16 ) ) ;
#19307=CARTESIAN_POINT ( 'NONE',  ( 16.02187500061451431, 5.824947211148865298E-16, -4.756430356249998326 ) ) ;
#19319=CARTESIAN_POINT ( 'NONE',  ( 10.73437500061451644, 5.492252693125287522, 3.363034840372157021E-16 ) ) ;
#19325=ORIENTED_EDGE ( 'NONE', *, *, #37028, .F. ) ;
#19326=CARTESIAN_POINT ( 'NONE',  ( 10.42500000000000071, 6.123233995736764310E-16, -4.999999999999998224 ) ) ;
#19330=CARTESIAN_POINT ( 'NONE',  ( 29.70937500061451431, 2.746126346562643317, 4.756430356249998326 ) ) ;
#19334=CARTESIAN_POINT ( 'NONE',  ( 7.912499999999999645, 2.886751345948126879, 4.999999999999999112 ) ) ;
#19342=CARTESIAN_POINT ( 'NONE',  ( 25.80937500061451928, 0.000000000000000000, 4.756430356249998326 ) ) ;
#19344=CARTESIAN_POINT ( 'NONE',  ( 9.421875000614519990, 2.746126346562645981, -4.756430356249997438 ) ) ;
#19355=FILL_AREA_STYLE ('',( #25274 ) ) ;
#19360=CARTESIAN_POINT ( 'NONE',  ( 21.39375000122903359, 5.773502691896255534, 3.535250795749688894E-16 ) ) ;
#19375=FACE_OUTER_BOUND ( 'NONE', #6414, .T. ) ;
#19384=CYLINDRICAL_SURFACE ( 'NONE', #54798, 4.999999999999998224 ) ;
#19394=CARTESIAN_POINT ( 'NONE',  ( 11.11875000122903323, 2.886751345948182834, 4.999999999999902300 ) ) ;
#19403=EDGE_CURVE ( 'NONE', #67375, #19923, #26224, .T. ) ;
#19407=VERTEX_POINT ( 'NONE', #55235 ) ;
#19414=CARTESIAN_POINT ( 'NONE',  ( 16.20937500061451431, 2.746126346562643317, 4.756430356249998326 ) ) ;
#19422=FACE_OUTER_BOUND ( 'NONE', #2144, .T. ) ;
#19431=FACE_OUTER_BOUND ( 'NONE', #46352, .T. ) ;
#19434=CARTESIAN_POINT ( 'NONE',  ( 17.10937500061451999, 4.119189519843966529, -2.378215178124998275 ) ) ;
#19444=CARTESIAN_POINT ( 'NONE',  ( 45.00000000000000000, 0.000000000000000000, 0.000000000000000000 ) ) ;
#19446=VECTOR ( 'NONE', #41636, 1000.000000000000000 ) ;
#19452=CARTESIAN_POINT ( 'NONE',  ( 27.31875000122903074, 2.886751345948126879, 4.999999999999999112 ) ) ;
#19467=ORIENTED_EDGE ( 'NONE', *, *, #15878, .F. ) ;
#19480=CARTESIAN_POINT ( 'NONE',  ( 29.06250000000000000, 2.886751345948126879, 4.999999999999999112 ) ) ;
#19486=CARTESIAN_POINT ( 'NONE',  ( 28.85625000122903216, -4.330127018922190985, -2.500000000000001332 ) ) ;
#19491=VECTOR ( 'NONE', #43108, 1000.000000000000227 ) ;
#19500=CARTESIAN_POINT ( 'NONE',  ( 16.17187500061451644, 4.119189519843966529, 2.378215178124999607 ) ) ;
#19503=CARTESIAN_POINT ( 'NONE',  ( 24.34687500061451715, 0.000000000000000000, 4.756430356249998326 ) ) ;
#19511=CARTESIAN_POINT ( 'NONE',  ( 23.75625000122903074, 0.000000000000000000, 4.999999999999998224 ) ) ;
#19519=CARTESIAN_POINT ( 'NONE',  ( 23.70937500061451786, -4.119189519843965641, -2.378215178125001383 ) ) ;
#19540=CARTESIAN_POINT ( 'NONE',  ( 12.87187500061451750, -5.492252693125287522, -1.008910452111647106E-15 ) ) ;
#19569=CARTESIAN_POINT ( 'NONE',  ( 13.65937500061451715, 0.000000000000000000, 4.756430356249998326 ) ) ;
#19575=CARTESIAN_POINT ( 'NONE',  ( 15.82499999999999929, 6.123233995736764310E-16, -4.999999999999998224 ) ) ;
#19579=CARTESIAN_POINT ( 'NONE',  ( 24.00937500061451502, -5.492252693125287522, -1.008910452111647106E-15 ) ) ;
#19580=CARTESIAN_POINT ( 'NONE',  ( 26.32499999999999929, 4.330127018922191873, 2.499999999999999556 ) ) ;
#19583=DIRECTION ( 'NONE',  ( -1.000000000000000000, -0.000000000000000000, -0.000000000000000000 ) ) ;
#19587=CARTESIAN_POINT ( 'NONE',  ( 22.73437500061451999, -2.746126346562642428, -4.756430356249999214 ) ) ;
#19589=CARTESIAN_POINT ( 'NONE',  ( 8.484375000614518214, 5.492252693125287522, 3.363034840372157021E-16 ) ) ;
#19600=CARTESIAN_POINT ( 'NONE',  ( 8.371875000614515727, 5.824947211148865298E-16, -4.756430356249998326 ) ) ;
#19611=ORIENTED_EDGE ( 'NONE', *, *, #43245, .T. ) ;
#19623=CARTESIAN_POINT ( 'NONE',  ( 19.58437500061451786, -4.119189519843968306, 2.378215178124996054 ) ) ;
#19655=VECTOR ( 'NONE', #12514, 1000.000000000000000 ) ;
#19658=CARTESIAN_POINT ( 'NONE',  ( 21.42187500061451644, -5.492252693125287522, -1.008910452111647106E-15 ) ) ;
#19665=CARTESIAN_POINT ( 'NONE',  ( 22.72499999999999787, 4.330127018922191873, 2.499999999999999556 ) ) ;
#19667=CARTESIAN_POINT ( 'NONE',  ( 9.112499999999998934, 2.886751345948073588, -5.000000000000094147 ) ) ;
#19676=CARTESIAN_POINT ( 'NONE',  ( 29.40937500061451360, -5.492252693125287522, -1.008910452111647106E-15 ) ) ;
#19678=CARTESIAN_POINT ( 'NONE',  ( 14.93437500061451573, -2.746126346562646425, 4.756430356249996549 ) ) ;
#19687=VECTOR ( 'NONE', #9430, 1000.000000000000000 ) ;
#19690=CARTESIAN_POINT ( 'NONE',  ( 7.284375000614517148, -2.746126346562646425, 4.756430356249996549 ) ) ;
#19691=ORIENTED_EDGE ( 'NONE', *, *, #7459, .T. ) ;
#19695=ORIENTED_EDGE ( 'NONE', *, *, #5795, .T. ) ;
#19696=CARTESIAN_POINT ( 'NONE',  ( 10.38750000000000107, -2.886751345948126435, -5.000000000000000000 ) ) ;
#19701=CARTESIAN_POINT ( 'NONE',  ( 28.80937500061451217, 2.746126346562643317, 4.756430356249998326 ) ) ;
#19705=CARTESIAN_POINT ( 'NONE',  ( 8.212500000000000355, 2.886751345948129099, -4.999999999999998224 ) ) ;
#19713=CARTESIAN_POINT ( 'NONE',  ( 25.58437500061451431, 5.824947211148865298E-16, -4.756430356249998326 ) ) ;
#19715=CARTESIAN_POINT ( 'NONE',  ( 11.07187500061451679, -5.492252693125287522, -1.008910452111647106E-15 ) ) ;
#19722=( BOUNDED_CURVE ( )  B_SPLINE_CURVE ( 2, ( #11084, #28088, #50616, #11452, #56512, #28439, #50974 ),
 .UNSPECIFIED., .F., .F. ) 
 B_SPLINE_CURVE_WITH_KNOTS ( ( 3, 2, 2, 3 ),
 ( 0.6100000000000002087, 0.6133333333333333970, 0.6166666666666668073, 0.6199999999999999956 ),
 .UNSPECIFIED. ) 
 CURVE ( )  GEOMETRIC_REPRESENTATION_ITEM ( )  RATIONAL_B_SPLINE_CURVE ( ( 0.9999999999999911182, 0.8660254037844475894, 1.000000000000000000, 0.8660254037844387076, 1.000000000000000000, 0.8660254037844387076, 1.000000000000000000 ) ) 
 REPRESENTATION_ITEM ( '' )  );
#19734=CARTESIAN_POINT ( 'NONE',  ( 20.34375000122903288, -2.886751345948125991, -5.000000000000000000 ) ) ;
#19736=CARTESIAN_POINT ( 'NONE',  ( 21.50625000122903074, 0.000000000000000000, 4.999999999999998224 ) ) ;
#19740=EDGE_CURVE ( 'NONE', #24417, #34969, #61180, .T. ) ;
#19750=CARTESIAN_POINT ( 'NONE',  ( 27.53437500061451360, 4.119189519843966529, 2.378215178124999607 ) ) ;
#19753=AXIS2_PLACEMENT_3D ( 'NONE', #57716, #7121, #24464 ) ;
#19767=CARTESIAN_POINT ( 'NONE',  ( 23.06250000000000000, 2.886751345948129099, -4.999999999999997335 ) ) ;
#19775=CARTESIAN_POINT ( 'NONE',  ( 28.19999999999999929, 0.000000000000000000, 4.999999999999998224 ) ) ;
#19780=ORIENTED_EDGE ( 'NONE', *, *, #37028, .T. ) ;
#19784=EDGE_LOOP ( 'NONE', ( #51968, #47410, #67170, #13521 ) ) ;
#19785=CARTESIAN_POINT ( 'NONE',  ( 25.72499999999999787, 6.123233995736764310E-16, -4.999999999999998224 ) ) ;
#19788=CARTESIAN_POINT ( 'NONE',  ( 16.50937500061451502, 2.746126346562645981, -4.756430356249997438 ) ) ;
#19804=LINE ( 'NONE', #41992, #52832 ) ;
#19807=CARTESIAN_POINT ( 'NONE',  ( 17.67187500061451644, 2.746126346562643317, 4.756430356249998326 ) ) ;
#19819=ORIENTED_EDGE ( 'NONE', *, *, #1067, .F. ) ;
#19826=CARTESIAN_POINT ( 'NONE',  ( 28.03125000122903288, 6.123233995736764310E-16, -4.999999999999998224 ) ) ;
#19838=ORIENTED_EDGE ( 'NONE', *, *, #5302, .F. ) ;
#19851=DIRECTION ( 'NONE',  ( -1.000000000000000000, -0.000000000000000000, -0.000000000000000000 ) ) ;
#19852=CARTESIAN_POINT ( 'NONE',  ( 29.25000000000000000, -4.330127018922190985, -2.500000000000001332 ) ) ;
#19858=CARTESIAN_POINT ( 'NONE',  ( 27.37500000000000000, -4.330127018922194537, 2.499999999999995559 ) ) ;
#19870=CARTESIAN_POINT ( 'NONE',  ( 15.19687500061451502, 4.119189519843966529, -2.378215178124998275 ) ) ;
#19873=CARTESIAN_POINT ( 'NONE',  ( 24.57187500061451502, 5.824947211148865298E-16, -4.756430356249998326 ) ) ;
#19882=CARTESIAN_POINT ( 'NONE',  ( 23.47499999999999787, 6.123233995736764310E-16, -4.999999999999998224 ) ) ;
#19883=CARTESIAN_POINT ( 'NONE',  ( 11.88749999999999751, 5.773502691896255534, 3.535250795749688894E-16 ) ) ;
#19890=CARTESIAN_POINT ( 'NONE',  ( 25.54687500061451644, -2.746126346562642428, -4.756430356249999214 ) ) ;
#19910=CARTESIAN_POINT ( 'NONE',  ( 12.30937500061451573, 0.000000000000000000, 4.756430356249998326 ) ) ;
#19922=VERTEX_POINT ( 'NONE', #34863 ) ;
#19923=VERTEX_POINT ( 'NONE', #57390 ) ;
#19938=CARTESIAN_POINT ( 'NONE',  ( 13.20937500061451786, 0.000000000000000000, 4.756430356249998326 ) ) ;
#19940=CARTESIAN_POINT ( 'NONE',  ( 13.51875000122903536, -5.773502691896255534, -1.060575238724906372E-15 ) ) ;
#19946=CARTESIAN_POINT ( 'NONE',  ( 15.71250000000000213, -5.773502691896255534, -1.060575238724906372E-15 ) ) ;
#19948=CARTESIAN_POINT ( 'NONE',  ( 45.00000000000000000, 0.000000000000000000, 0.000000000000000000 ) ) ;
#19952=CYLINDRICAL_SURFACE ( 'NONE', #22735, 4.999999999999998224 ) ;
#19957=CARTESIAN_POINT ( 'NONE',  ( 22.24687500061451573, -4.119189519843965641, -2.378215178125001383 ) ) ;
#19959=CARTESIAN_POINT ( 'NONE',  ( 9.571875000614515017, -4.119189519843968306, 2.378215178124996054 ) ) ;
#19966=CARTESIAN_POINT ( 'NONE',  ( 8.681250001229031454, 6.123233995736764310E-16, -4.999999999999998224 ) ) ;
#19968=CARTESIAN_POINT ( 'NONE',  ( 9.684375000614517504, -2.746126346562642428, -4.756430356249999214 ) ) ;
#19978=ORIENTED_EDGE ( 'NONE', *, *, #27431, .T. ) ;
#19990=CARTESIAN_POINT ( 'NONE',  ( 20.40937500061451715, 0.000000000000000000, 4.756430356249998326 ) ) ;
#20021=CARTESIAN_POINT ( 'NONE',  ( 21.68437500061451573, 4.119189519843966529, 2.378215178124999607 ) ) ;
#20027=CARTESIAN_POINT ( 'NONE',  ( 21.48750000000000071, -2.886751345948129988, 4.999999999999997335 ) ) ;
#20030=CARTESIAN_POINT ( 'NONE',  ( 45.00000000000000000, 6.123233995736764310E-16, -4.999999999999998224 ) ) ;
#20032=DIRECTION ( 'NONE',  ( 0.000000000000000000, 0.000000000000000000, 1.000000000000000000 ) ) ;
#20039=CARTESIAN_POINT ( 'NONE',  ( 29.25937500061451857, 2.746126346562643317, 4.756430356249998326 ) ) ;
#20041=CARTESIAN_POINT ( 'NONE',  ( 16.69687500061451502, 0.000000000000000000, 4.756430356249998326 ) ) ;
#20044=EDGE_LOOP ( 'NONE', ( #26348, #9822, #40193, #36051 ) ) ;
#20047=CARTESIAN_POINT ( 'NONE',  ( 17.15625000122903288, -4.330127018922190985, -2.500000000000001332 ) ) ;
#20050=CARTESIAN_POINT ( 'NONE',  ( 16.70625000122903359, -4.330127018922190985, -2.500000000000001332 ) ) ;
#20051=CARTESIAN_POINT ( 'NONE',  ( 8.371875000614515727, 5.824947211148865298E-16, -4.756430356249998326 ) ) ;
#20052=ORIENTED_EDGE ( 'NONE', *, *, #57093, .T. ) ;
#20057=CARTESIAN_POINT ( 'NONE',  ( 16.94999999999999929, 0.000000000000000000, 4.999999999999998224 ) ) ;
#20060=CARTESIAN_POINT ( 'NONE',  ( 19.93125000122903145, 6.123233995736764310E-16, -4.999999999999998224 ) ) ;
#20062=CARTESIAN_POINT ( 'NONE',  ( 29.03437500061451360, -2.746126346562642428, -4.756430356249999214 ) ) ;
#20073=CARTESIAN_POINT ( 'NONE',  ( 27.79687500061451644, -2.746126346562641984, -4.756430356249999214 ) ) ;
#20075=CARTESIAN_POINT ( 'NONE',  ( 11.29687500061451644, 5.492252693125287522, 3.363034840372157021E-16 ) ) ;
#20087=PRODUCT_CONTEXT ( 'NONE', #43151, 'mechanical' ) ;
#20092=CARTESIAN_POINT ( 'NONE',  ( 20.26875000122903003, -5.773502691896255534, -1.060575238724906372E-15 ) ) ;
#20110=CARTESIAN_POINT ( 'NONE',  ( 27.34687500061451360, -2.746126346562642428, -4.756430356249999214 ) ) ;
#20115=ADVANCED_FACE ( 'NONE', ( #32879 ), #44347, .T. ) ;
#20119=CARTESIAN_POINT ( 'NONE',  ( 7.518750001229031810, 2.886751345948126879, 4.999999999999998224 ) ) ;
#20133=DIRECTION ( 'NONE',  ( 0.000000000000000000, 0.000000000000000000, 1.000000000000000000 ) ) ;
#20136=CARTESIAN_POINT ( 'NONE',  ( 28.04999999999999716, 4.330127018922192761, -2.499999999999997780 ) ) ;
#20140=EDGE_LOOP ( 'NONE', ( #61509, #40122, #11990, #19183 ) ) ;
#20148=CARTESIAN_POINT ( 'NONE',  ( 16.24687500061451573, 0.000000000000000000, 4.756430356249998326 ) ) ;
#20157=EDGE_LOOP ( 'NONE', ( #42698, #38536, #46786 ) ) ;
#20163=CARTESIAN_POINT ( 'NONE',  ( 15.35625000122903216, -4.330127018922190985, -2.500000000000001332 ) ) ;
#20164=CARTESIAN_POINT ( 'NONE',  ( 9.731250001229033941, 4.330127018922191873, 2.499999999999999556 ) ) ;
#20168=CARTESIAN_POINT ( 'NONE',  ( 18.45937500061451431, 4.119189519843966529, -2.378215178124998275 ) ) ;
#20177=PRODUCT_DEFINITION_SHAPE ( 'NONE', 'NONE',  #2500 ) ;
#20186=CARTESIAN_POINT ( 'NONE',  ( 28.66875000122902861, 2.886751345948126879, 4.999999999999999112 ) ) ;
#20188=DIRECTION ( 'NONE',  ( 0.000000000000000000, 0.000000000000000000, 1.000000000000000000 ) ) ;
#20202=CARTESIAN_POINT ( 'NONE',  ( 15.88125000122903074, 6.123233995736764310E-16, -4.999999999999998224 ) ) ;
#20211=CARTESIAN_POINT ( 'NONE',  ( 17.45625000122903003, 0.000000000000000000, 4.999999999999998224 ) ) ;
#20212=CARTESIAN_POINT ( 'NONE',  ( 29.84999999999999787, 4.330127018922192761, -2.499999999999997780 ) ) ;
#20214=CYLINDRICAL_SURFACE ( 'NONE', #41762, 4.999999999999998224 ) ;
#20231=CARTESIAN_POINT ( 'NONE',  ( 15.30937500061451573, 2.746126346562643317, 4.756430356249998326 ) ) ;
#20232=ORIENTED_EDGE ( 'NONE', *, *, #52283, .F. ) ;
#20235=CARTESIAN_POINT ( 'NONE',  ( 24.04687500061451289, -4.119189519843965641, -2.378215178125001383 ) ) ;
#20245=CARTESIAN_POINT ( 'NONE',  ( 13.27500000000000213, 4.330127018922191873, 2.499999999999999556 ) ) ;
#20252=CARTESIAN_POINT ( 'NONE',  ( 24.53437500061451715, -4.119189519843968306, 2.378215178124996054 ) ) ;
#20256=CYLINDRICAL_SURFACE ( 'NONE', #62165, 4.999999999999998224 ) ;
#20272=CARTESIAN_POINT ( 'NONE',  ( 12.53437500061451537, 5.824947211148865298E-16, -4.756430356249998326 ) ) ;
#20285=ORIENTED_EDGE ( 'NONE', *, *, #18491, .T. ) ;
#20296=ORIENTED_EDGE ( 'NONE', *, *, #50099, .F. ) ;
#20300=CARTESIAN_POINT ( 'NONE',  ( 13.58437500061451786, 4.119189519843966529, 2.378215178124999607 ) ) ;
#20309=CARTESIAN_POINT ( 'NONE',  ( 14.32500000000000107, -4.330127018922194537, 2.499999999999995559 ) ) ;
#20321=CARTESIAN_POINT ( 'NONE',  ( 21.87187500061451573, 5.824947211148865298E-16, -4.756430356249998326 ) ) ;
#20323=CARTESIAN_POINT ( 'NONE',  ( 9.984375000614516438, -2.746126346562646425, 4.756430356249996549 ) ) ;
#20329=EDGE_CURVE ( 'NONE', #46244, #21751, #9256, .T. ) ;
#20335=CARTESIAN_POINT ( 'NONE',  ( 10.17187500061451644, 5.824947211148865298E-16, -4.756430356249998326 ) ) ;
#20358=( BOUNDED_CURVE ( )  B_SPLINE_CURVE ( 2, ( #41355, #63865, #53154, #47614, #70144, #64602, #59048 ),
 .UNSPECIFIED., .F., .F. ) 
 B_SPLINE_CURVE_WITH_KNOTS ( ( 3, 2, 2, 3 ),
 ( 0.2100000000000000477, 0.2133333333333333748, 0.2166666666666667018, 0.2200000000000000011 ),
 .UNSPECIFIED. ) 
 CURVE ( )  GEOMETRIC_REPRESENTATION_ITEM ( )  RATIONAL_B_SPLINE_CURVE ( ( 0.9999999999999977796, 0.8660254037844409281, 1.000000000000000000, 0.8660254037844387076, 1.000000000000000000, 0.8660254037844387076, 1.000000000000000000 ) ) 
 REPRESENTATION_ITEM ( '' )  );
#20360=CARTESIAN_POINT ( 'NONE',  ( 18.49687500061452283, 5.492252693125287522, 3.363034840372157021E-16 ) ) ;
#20364=EDGE_LOOP ( 'NONE', ( #43224, #52440, #69132, #50720 ) ) ;
#20393=CARTESIAN_POINT ( 'NONE',  ( 21.49687500061451573, -2.746126346562642428, -4.756430356249999214 ) ) ;
#20399=CARTESIAN_POINT ( 'NONE',  ( 22.57499999999999929, 6.123233995736764310E-16, -4.999999999999998224 ) ) ;
#20406=CARTESIAN_POINT ( 'NONE',  ( 11.98125000122903394, 4.330127018922191873, 2.499999999999999556 ) ) ;
#20410=CARTESIAN_POINT ( 'NONE',  ( 7.856250001229033053, 4.330127018922192761, -2.499999999999997780 ) ) ;
#20412=CARTESIAN_POINT ( 'NONE',  ( 15.90937500061451537, -5.492252693125287522, -1.008910452111647106E-15 ) ) ;
#20422=CARTESIAN_POINT ( 'NONE',  ( 8.746875000614515727, -4.119189519843965641, -2.378215178125001383 ) ) ;
#20431=CARTESIAN_POINT ( 'NONE',  ( 19.70625000122903359, 0.000000000000000000, 4.999999999999998224 ) ) ;
#20437=CARTESIAN_POINT ( 'NONE',  ( 8.887499999999999289, -2.886751345948129988, 4.999999999999997335 ) ) ;
#20438=CYLINDRICAL_SURFACE ( 'NONE', #36028, 4.999999999999998224 ) ;
#20444=CARTESIAN_POINT ( 'NONE',  ( 27.38437500061451857, 5.824947211148865298E-16, -4.756430356249998326 ) ) ;
#20461=CARTESIAN_POINT ( 'NONE',  ( 21.76875000122903359, 2.886751345948129099, -4.999999999999998224 ) ) ;
#20477=CARTESIAN_POINT ( 'NONE',  ( 29.03437500061451715, -4.119189519843968306, 2.378215178124996054 ) ) ;
#20493=CARTESIAN_POINT ( 'NONE',  ( 10.93125000122903501, 6.123233995736764310E-16, -4.999999999999998224 ) ) ;
#20512=CARTESIAN_POINT ( 'NONE',  ( 14.10937500061451644, -5.492252693125287522, -1.008910452111647106E-15 ) ) ;
#20520=EDGE_LOOP ( 'NONE', ( #69993, #70575, #41880, #11576 ) ) ;
#20526=CARTESIAN_POINT ( 'NONE',  ( 9.693750001229032520, 5.773502691896255534, 3.535250795749688401E-16 ) ) ;
#20529=CARTESIAN_POINT ( 'NONE',  ( 8.681250001229031454, 6.123233995736764310E-16, -4.999999999999998224 ) ) ;
#20530=CARTESIAN_POINT ( 'NONE',  ( 16.69687500061451502, 5.492252693125287522, 3.363034840372157021E-16 ) ) ;
#20533=( BOUNDED_CURVE ( )  B_SPLINE_CURVE ( 2, ( #63286, #7143, #29673, #24121, #25493, #18569, #46670 ),
 .UNSPECIFIED., .F., .F. ) 
 B_SPLINE_CURVE_WITH_KNOTS ( ( 3, 2, 2, 3 ),
 ( 0.02999999999999993991, 0.03333333333333331899, 0.03666666666666669461, 0.04000000000000007022 ),
 .UNSPECIFIED. ) 
 CURVE ( )  GEOMETRIC_REPRESENTATION_ITEM ( )  RATIONAL_B_SPLINE_CURVE ( ( 1.000000000000002442, 0.8660254037844364872, 1.000000000000000000, 0.8660254037844387076, 1.000000000000000000, 0.8660254037844359321, 1.000000000000002887 ) ) 
 REPRESENTATION_ITEM ( '' )  );
#20549=CARTESIAN_POINT ( 'NONE',  ( 29.04375000122903216, 5.773502691896255534, 3.535250795749688894E-16 ) ) ;
#20551=DIRECTION ( 'NONE',  ( -1.000000000000000000, -0.000000000000000000, -0.000000000000000000 ) ) ;
#20577=CARTESIAN_POINT ( 'NONE',  ( 26.92499999999999716, -4.330127018922194537, 2.499999999999995559 ) ) ;
#20582=( BOUNDED_CURVE ( )  B_SPLINE_CURVE ( 2, ( #21429, #38434, #61683, #67609, #16974, #39900, #12166 ),
 .UNSPECIFIED., .F., .F. ) 
 B_SPLINE_CURVE_WITH_KNOTS ( ( 3, 2, 2, 3 ),
 ( 0.3900000000000000133, 0.3933333333333333126, 0.3966666666666667229, 0.4000000000000000777 ),
 .UNSPECIFIED. ) 
 CURVE ( )  GEOMETRIC_REPRESENTATION_ITEM ( )  RATIONAL_B_SPLINE_CURVE ( ( 1.000000000000000000, 0.8660254037844387076, 1.000000000000000000, 0.8660254037844387076, 1.000000000000000000, 0.8660254037844364872, 1.000000000000002220 ) ) 
 REPRESENTATION_ITEM ( '' )  );
#20583=CARTESIAN_POINT ( 'NONE',  ( 12.59999999999999964, -4.330127018922190985, -2.500000000000001332 ) ) ;
#20596=ADVANCED_FACE ( 'NONE', ( #68322 ), #50602, .T. ) ;
#20597=CARTESIAN_POINT ( 'NONE',  ( 13.80937500061451395, 2.746126346562645981, -4.756430356249997438 ) ) ;
#20601=CARTESIAN_POINT ( 'NONE',  ( 24.00937500061451502, -5.492252693125287522, -1.008910452111647106E-15 ) ) ;
#20612=CARTESIAN_POINT ( 'NONE',  ( 12.82499999999999929, 4.330127018922191873, 2.499999999999999556 ) ) ;
#20620=CARTESIAN_POINT ( 'NONE',  ( 24.42187500061451999, 2.746126346562643317, 4.756430356249998326 ) ) ;
#20632=AXIS2_PLACEMENT_3D ( 'NONE', #65611, #64878, #53436 ) ;
#20641=CARTESIAN_POINT ( 'NONE',  ( 10.88437500061451679, 4.119189519843966529, 2.378215178124999607 ) ) ;
#20669=CARTESIAN_POINT ( 'NONE',  ( 14.67187500061451821, -5.492252693125287522, -1.008910452111647106E-15 ) ) ;
#20678=CARTESIAN_POINT ( 'NONE',  ( 15.37500000000000000, 6.123233995736764310E-16, -4.999999999999998224 ) ) ;
#20689=CARTESIAN_POINT ( 'NONE',  ( 23.22187500061451360, 5.824947211148865298E-16, -4.756430356249998326 ) ) ;
#20704=CARTESIAN_POINT ( 'NONE',  ( 9.346875000614517148, 4.119189519843966529, -2.378215178124998275 ) ) ;
#20727=CARTESIAN_POINT ( 'NONE',  ( 16.05937500061451573, -4.119189519843965641, -2.378215178125001383 ) ) ;
#20756=VERTEX_POINT ( 'NONE', #35051 ) ;
#20760=CARTESIAN_POINT ( 'NONE',  ( 21.53437500061451715, 5.824947211148865298E-16, -4.756430356249998326 ) ) ;
#20762=EDGE_CURVE ( 'NONE', #47145, #28470, #5172, .T. ) ;
#20767=CARTESIAN_POINT ( 'NONE',  ( 23.17500000000000071, 4.330127018922191873, 2.499999999999999556 ) ) ;
#20772=CARTESIAN_POINT ( 'NONE',  ( 18.95625000122903003, -4.330127018922190985, -2.500000000000001332 ) ) ;
#20778=CARTESIAN_POINT ( 'NONE',  ( 8.081250001229031810, -4.330127018922194537, 2.499999999999995559 ) ) ;
#20781=CARTESIAN_POINT ( 'NONE',  ( 13.28437500061451537, -2.746126346562641984, -4.756430356249999214 ) ) ;
#20792=CARTESIAN_POINT ( 'NONE',  ( 8.896875000614517859, 4.119189519843966529, -2.378215178124998275 ) ) ;
#20794=EDGE_CURVE ( 'NONE', #72010, #31518, #57579, .T. ) ;
#20808=AXIS2_PLACEMENT_3D ( 'NONE', #22983, #63866, #58684 ) ;
#20815=CARTESIAN_POINT ( 'NONE',  ( 23.74687500061451573, -2.746126346562641984, -4.756430356249999214 ) ) ;
#20817=DIRECTION ( 'NONE',  ( 0.000000000000000000, 0.000000000000000000, 1.000000000000000000 ) ) ;
#20825=( BOUNDED_CURVE ( )  B_SPLINE_CURVE ( 2, ( #48628, #71528, #65979, #15359, #60419, #52075, #2459 ),
 .UNSPECIFIED., .F., .F. ) 
 B_SPLINE_CURVE_WITH_KNOTS ( ( 3, 2, 2, 3 ),
 ( 0.8900000000000000133, 0.8933333333333333126, 0.8966666666666666119, 0.9000000000000000222 ),
 .UNSPECIFIED. ) 
 CURVE ( )  GEOMETRIC_REPRESENTATION_ITEM ( )  RATIONAL_B_SPLINE_CURVE ( ( 1.000000000000000000, 0.8660254037844387076, 1.000000000000000000, 0.8660254037844387076, 1.000000000000000000, 0.8660254037844387076, 1.000000000000000000 ) ) 
 REPRESENTATION_ITEM ( '' )  );
#20829=AXIS2_PLACEMENT_3D ( 'NONE', #55856, #51396, #5965 ) ;
#20836=CARTESIAN_POINT ( 'NONE',  ( 18.54375000122902861, -2.886751345948125991, -5.000000000000000000 ) ) ;
#20839=ORIENTED_EDGE ( 'NONE', *, *, #44780, .T. ) ;
#20844=CARTESIAN_POINT ( 'NONE',  ( 20.99999999999999645, 0.000000000000000000, 4.999999999999998224 ) ) ;
#20852=CARTESIAN_POINT ( 'NONE',  ( 29.25937500061451502, 4.119189519843966529, -2.378215178124998275 ) ) ;
#20860=CARTESIAN_POINT ( 'NONE',  ( 22.18125000122903145, 6.123233995736764310E-16, -4.999999999999998224 ) ) ;
#20878=CARTESIAN_POINT ( 'NONE',  ( 9.356250001229033941, 0.000000000000000000, 4.999999999999998224 ) ) ;
#20889=CARTESIAN_POINT ( 'NONE',  ( 13.24687500061451750, -4.119189519843965641, -2.378215178125001383 ) ) ;
#20897=ORIENTED_EDGE ( 'NONE', *, *, #9282, .T. ) ;
#20903=CARTESIAN_POINT ( 'NONE',  ( 15.28125000122903288, -4.330127018922194537, 2.499999999999995559 ) ) ;
#20908=CARTESIAN_POINT ( 'NONE',  ( 15.83437500061451608, 4.119189519843966529, 2.378215178124999607 ) ) ;
#20918=CARTESIAN_POINT ( 'NONE',  ( 12.95625000122903359, 0.000000000000000000, 4.999999999999998224 ) ) ;
#20921=CARTESIAN_POINT ( 'NONE',  ( 21.73125000122903216, 6.123233995736764310E-16, -4.999999999999998224 ) ) ;
#20925=CARTESIAN_POINT ( 'NONE',  ( 26.53125000122902932, -4.330127018922194537, 2.499999999999995559 ) ) ;
#20927=DIRECTION ( 'NONE',  ( -1.000000000000000000, -0.000000000000000000, -0.000000000000000000 ) ) ;
#20930=CARTESIAN_POINT ( 'NONE',  ( 8.175000000000002487, 6.123233995736764310E-16, -4.999999999999998224 ) ) ;
#20967=( BOUNDED_CURVE ( )  B_SPLINE_CURVE ( 2, ( #12927, #63894, #19182, #59815, #54650, #37292, #30651 ),
 .UNSPECIFIED., .F., .F. ) 
 B_SPLINE_CURVE_WITH_KNOTS ( ( 3, 2, 2, 3 ),
 ( 0.2700000000000000733, 0.2733333333333333726, 0.2766666666666666718, 0.2800000000000000266 ),
 .UNSPECIFIED. ) 
 CURVE ( )  GEOMETRIC_REPRESENTATION_ITEM ( )  RATIONAL_B_SPLINE_CURVE ( ( 0.9999999999999977796, 0.8660254037844409281, 1.000000000000000000, 0.8660254037844387076, 1.000000000000000000, 0.8660254037844387076, 1.000000000000000000 ) ) 
 REPRESENTATION_ITEM ( '' )  );
#20973=CARTESIAN_POINT ( 'NONE',  ( 21.12187500061451217, 4.119189519843966529, 2.378215178124999607 ) ) ;
#20977=CARTESIAN_POINT ( 'NONE',  ( 13.85625000122903216, 0.000000000000000000, 4.999999999999998224 ) ) ;
#20981=CARTESIAN_POINT ( 'NONE',  ( 23.36250000000000071, -5.773502691896255534, -1.060575238724906372E-15 ) ) ;
#20983=CARTESIAN_POINT ( 'NONE',  ( 14.10000000000000142, 4.330127018922192761, -2.499999999999997780 ) ) ;
#20990=CARTESIAN_POINT ( 'NONE',  ( 22.24687500061451217, -2.746126346562646425, 4.756430356249996549 ) ) ;
#21012=CARTESIAN_POINT ( 'NONE',  ( 9.834375000614517859, 5.824947211148865298E-16, -4.756430356249998326 ) ) ;
#21039=CARTESIAN_POINT ( 'NONE',  ( 11.97187500061451892, -5.492252693125287522, -1.008910452111647106E-15 ) ) ;
#21042=CARTESIAN_POINT ( 'NONE',  ( 13.48125000122903394, -4.330127018922194537, 2.499999999999995559 ) ) ;
#21059=CARTESIAN_POINT ( 'NONE',  ( 19.65937500061451360, 2.746126346562645981, -4.756430356249997438 ) ) ;
#21062=CARTESIAN_POINT ( 'NONE',  ( 14.34375000122903465, -2.886751345948129988, 4.999999999999997335 ) ) ;
#21064=CARTESIAN_POINT ( 'NONE',  ( 7.546875000614516438, 4.119189519843966529, -2.378215178124998275 ) ) ;
#21076=CARTESIAN_POINT ( 'NONE',  ( 9.384375000614516793, 5.492252693125287522, 3.363034840372157021E-16 ) ) ;
#21085=ORIENTED_EDGE ( 'NONE', *, *, #62697, .F. ) ;
#21097=CARTESIAN_POINT ( 'NONE',  ( 17.29687500061451999, -2.746126346562646425, 4.756430356249996549 ) ) ;
#21128=CARTESIAN_POINT ( 'NONE',  ( 19.39687500061451786, 5.492252693125287522, 3.363034840372157021E-16 ) ) ;
#21135=CARTESIAN_POINT ( 'NONE',  ( 21.89999999999999858, 0.000000000000000000, 4.999999999999998224 ) ) ;
#21137=CARTESIAN_POINT ( 'NONE',  ( 20.62499999999999645, -4.330127018922194537, 2.499999999999995559 ) ) ;
#21138=CARTESIAN_POINT ( 'NONE',  ( 18.58125000122903003, 6.123233995736764310E-16, -4.999999999999998224 ) ) ;
#21145=CARTESIAN_POINT ( 'NONE',  ( 27.72187500061451715, 5.824947211148865298E-16, -4.756430356249998326 ) ) ;
#21147=CARTESIAN_POINT ( 'NONE',  ( 13.20937500061451431, -5.492252693125287522, -1.008910452111647106E-15 ) ) ;
#21157=CARTESIAN_POINT ( 'NONE',  ( 16.74375000122903145, -2.886751345948181946, -4.999999999999904077 ) ) ;
#21158=CARTESIAN_POINT ( 'NONE',  ( 7.884375000614518569, -2.746126346562642428, -4.756430356249999214 ) ) ;
#21159=EDGE_LOOP ( 'NONE', ( #42976, #47050, #51122, #6538 ) ) ;
#21172=CARTESIAN_POINT ( 'NONE',  ( 25.59375000122903643, -2.886751345948157965, 4.999999999999948486 ) ) ;
#21180=CARTESIAN_POINT ( 'NONE',  ( 24.98437500061451644, -4.119189519843968306, 2.378215178124996054 ) ) ;
#21182=CARTESIAN_POINT ( 'NONE',  ( 8.596875000614518925, 5.492252693125287522, 3.363034840372157021E-16 ) ) ;
#21184=( BOUNDED_CURVE ( )  B_SPLINE_CURVE ( 2, ( #72632, #5033, #5396, #60801, #67102, #27570, #72994 ),
 .UNSPECIFIED., .F., .F. ) 
 B_SPLINE_CURVE_WITH_KNOTS ( ( 3, 2, 2, 3 ),
 ( 0.8600000000000002087, 0.8633333333333333970, 0.8666666666666668073, 0.8699999999999999956 ),
 .UNSPECIFIED. ) 
 CURVE ( )  GEOMETRIC_REPRESENTATION_ITEM ( )  RATIONAL_B_SPLINE_CURVE ( ( 0.9999999999999911182, 0.8660254037844475894, 1.000000000000000000, 0.8660254037844387076, 1.000000000000000000, 0.8660254037844387076, 1.000000000000000000 ) ) 
 REPRESENTATION_ITEM ( '' )  );
#21193=CARTESIAN_POINT ( 'NONE',  ( 8.231250001229033941, 6.123233995736764310E-16, -4.999999999999998224 ) ) ;
#21200=CARTESIAN_POINT ( 'NONE',  ( 17.83125000122903003, 4.330127018922191873, 2.499999999999999556 ) ) ;
#21216=CARTESIAN_POINT ( 'NONE',  ( 29.37187500061451928, 2.746126346562643317, 4.756430356249998326 ) ) ;
#21231=CARTESIAN_POINT ( 'NONE',  ( 11.00625000122903252, 4.330127018922192761, -2.499999999999997780 ) ) ;
#21235=CARTESIAN_POINT ( 'NONE',  ( 20.55937500061451217, 2.746126346562645981, -4.756430356249997438 ) ) ;
#21253=CARTESIAN_POINT ( 'NONE',  ( 11.06250000000000178, 2.886751345948126879, 4.999999999999998224 ) ) ;
#21254=CARTESIAN_POINT ( 'NONE',  ( 15.27187500061451608, 4.119189519843966529, 2.378215178124999607 ) ) ;
#21264=CARTESIAN_POINT ( 'NONE',  ( 16.85625000122903572, 4.330127018922192761, -2.499999999999997780 ) ) ;
#21268=CARTESIAN_POINT ( 'NONE',  ( 17.10000000000000142, -4.330127018922190985, -2.500000000000001332 ) ) ;
#21271=DIRECTION ( 'NONE',  ( -1.000000000000000000, -0.000000000000000000, -0.000000000000000000 ) ) ;
#21272=CARTESIAN_POINT ( 'NONE',  ( 14.25937500061451679, -4.119189519843965641, -2.378215178125001383 ) ) ;
#21282=CARTESIAN_POINT ( 'NONE',  ( 12.97499999999999964, -4.330127018922194537, 2.499999999999995559 ) ) ;
#21286=CARTESIAN_POINT ( 'NONE',  ( 21.58125000122903359, -4.330127018922194537, 2.499999999999995559 ) ) ;
#21290=CARTESIAN_POINT ( 'NONE',  ( 25.40625000122903288, 4.330127018922192761, -2.499999999999997780 ) ) ;
#21293=LINE ( 'NONE', #59344, #58458 ) ;
#21301=ORIENTED_EDGE ( 'NONE', *, *, #9426, .F. ) ;
#21303=CARTESIAN_POINT ( 'NONE',  ( 10.33125000122903359, -4.330127018922194537, 2.499999999999995559 ) ) ;
#21339=CARTESIAN_POINT ( 'NONE',  ( 21.98437500061451644, 5.492252693125287522, 3.363034840372157021E-16 ) ) ;
#21347=CARTESIAN_POINT ( 'NONE',  ( 12.15000000000000036, -4.330127018922190985, -2.500000000000001332 ) ) ;
#21354=CARTESIAN_POINT ( 'NONE',  ( 23.29687500061451644, -2.746126346562642428, -4.756430356249999214 ) ) ;
#21358=LINE ( 'NONE', #31358, #37227 ) ;
#21377=CARTESIAN_POINT ( 'NONE',  ( 10.69687500061451679, -2.746126346562641984, -4.756430356249999214 ) ) ;
#21386=ORIENTED_EDGE ( 'NONE', *, *, #33660, .F. ) ;
#21389=LINE ( 'NONE', #16214, #5529 ) ;
#21401=CARTESIAN_POINT ( 'NONE',  ( 10.65937500061451715, -4.119189519843965641, -2.378215178125001383 ) ) ;
#21410=CYLINDRICAL_SURFACE ( 'NONE', #24353, 4.999999999999998224 ) ;
#21420=CARTESIAN_POINT ( 'NONE',  ( 20.37187500061451217, -4.119189519843968306, 2.378215178124996054 ) ) ;
#21423=CARTESIAN_POINT ( 'NONE',  ( 13.96875000122903465, -5.773502691896255534, -1.060575238724906372E-15 ) ) ;
#21429=CARTESIAN_POINT ( 'NONE',  ( 21.22500000000000142, 6.123233995736764310E-16, -4.999999999999998224 ) ) ;
#21437=CARTESIAN_POINT ( 'NONE',  ( 8.071875000614515017, 4.119189519843966529, 2.378215178124999607 ) ) ;
#21460=CARTESIAN_POINT ( 'NONE',  ( 18.08437500061451431, 4.119189519843966529, 2.378215178124999607 ) ) ;
#21481=EDGE_CURVE ( 'NONE', #58840, #50518, #49318, .T. ) ;
#21495=CARTESIAN_POINT ( 'NONE',  ( 19.65937500061451360, -4.119189519843965641, -2.378215178125001383 ) ) ;
#21501=CARTESIAN_POINT ( 'NONE',  ( 20.40000000000000213, 4.330127018922192761, -2.499999999999997780 ) ) ;
#21504=CARTESIAN_POINT ( 'NONE',  ( 19.25625000122903430, 0.000000000000000000, 4.999999999999998224 ) ) ;
#21511=CARTESIAN_POINT ( 'NONE',  ( 26.93437500061451573, 5.492252693125287522, 3.363034840372157021E-16 ) ) ;
#21513=CARTESIAN_POINT ( 'NONE',  ( 13.80937500061451395, 2.746126346562645981, -4.756430356249997438 ) ) ;
#21523=ORIENTED_EDGE ( 'NONE', *, *, #51187, .T. ) ;
#21536=CARTESIAN_POINT ( 'NONE',  ( 16.25625000122903074, -4.330127018922190985, -2.500000000000001332 ) ) ;
#21537=ORIENTED_EDGE ( 'NONE', *, *, #23281, .F. ) ;
#21539=CARTESIAN_POINT ( 'NONE',  ( 29.32499999999999929, 6.123233995736764310E-16, -4.999999999999998224 ) ) ;
#21547=CARTESIAN_POINT ( 'NONE',  ( 25.43437500061451573, -4.119189519843968306, 2.378215178124996054 ) ) ;
#21552=ADVANCED_FACE ( 'NONE', ( #8975 ), #18935, .T. ) ;
#21557=CARTESIAN_POINT ( 'NONE',  ( 27.07499999999999929, 6.123233995736764310E-16, -4.999999999999998224 ) ) ;
#21568=CARTESIAN_POINT ( 'NONE',  ( 19.18125000122903501, 4.330127018922191873, 2.499999999999999556 ) ) ;
#21584=CARTESIAN_POINT ( 'NONE',  ( 25.62187500061451573, 2.746126346562645981, -4.756430356249997438 ) ) ;
#21599=CARTESIAN_POINT ( 'NONE',  ( 11.41875000122903394, 2.886751345948129099, -4.999999999999998224 ) ) ;
#21603=CARTESIAN_POINT ( 'NONE',  ( 21.19687500061451502, 0.000000000000000000, 4.756430356249998326 ) ) ;
#21616=( BOUNDED_CURVE ( )  B_SPLINE_CURVE ( 2, ( #20844, #60729, #59999, #71838, #72927, #38203, #37840 ),
 .UNSPECIFIED., .F., .F. ) 
 B_SPLINE_CURVE_WITH_KNOTS ( ( 3, 2, 2, 3 ),
 ( 0.4000000000000000777, 0.4033333333333333215, 0.4066666666666666763, 0.4099999999999999201 ),
 .UNSPECIFIED. ) 
 CURVE ( )  GEOMETRIC_REPRESENTATION_ITEM ( )  RATIONAL_B_SPLINE_CURVE ( ( 0.9999999999999977796, 0.8660254037844409281, 1.000000000000000000, 0.8660254037844387076, 1.000000000000000000, 0.8660254037844409281, 0.9999999999999977796 ) ) 
 REPRESENTATION_ITEM ( '' )  );
#21620=CARTESIAN_POINT ( 'NONE',  ( 13.02187500061451786, 4.119189519843966529, 2.378215178124999607 ) ) ;
#21637=CARTESIAN_POINT ( 'NONE',  ( 14.44687500061451679, 5.492252693125287522, 3.363034840372157021E-16 ) ) ;
#21655=CARTESIAN_POINT ( 'NONE',  ( 25.59375000122903288, -2.886751345948129988, 4.999999999999997335 ) ) ;
#21668=CARTESIAN_POINT ( 'NONE',  ( 10.25625000122903252, 0.000000000000000000, 4.999999999999998224 ) ) ;
#21677=( BOUNDED_CURVE ( )  B_SPLINE_CURVE ( 3, ( #37196, #60083, #14294, #3225 ),
 .UNSPECIFIED., .F., .F. ) 
 B_SPLINE_CURVE_WITH_KNOTS ( ( 4, 4 ),
 ( 3.141592653589793116, 4.712388980384689674 ),
 .UNSPECIFIED. ) 
 CURVE ( )  GEOMETRIC_REPRESENTATION_ITEM ( )  RATIONAL_B_SPLINE_CURVE ( ( 1.000000000000000000, 0.8047378541243649375, 0.8047378541243649375, 1.000000000000000000 ) ) 
 REPRESENTATION_ITEM ( '' )  );
#21683=EDGE_CURVE ( 'NONE', #38944, #3324, #24495, .T. ) ;
#21704=CARTESIAN_POINT ( 'NONE',  ( 22.09687500061451360, 0.000000000000000000, 4.756430356249998326 ) ) ;
#21713=CARTESIAN_POINT ( 'NONE',  ( 10.53750000000000320, 5.773502691896255534, 3.535250795749688894E-16 ) ) ;
#21720=CARTESIAN_POINT ( 'NONE',  ( 22.32187500061451502, -5.492252693125287522, -1.008910452111647106E-15 ) ) ;
#21723=CARTESIAN_POINT ( 'NONE',  ( 20.28749999999999787, -2.886751345948181946, -4.999999999999904077 ) ) ;
#21731=AXIS2_PLACEMENT_3D ( 'NONE', #67581, #16947, #39500 ) ;
#21742=CARTESIAN_POINT ( 'NONE',  ( 9.571875000614518569, 2.746126346562643317, 4.756430356249998326 ) ) ;
#21751=VERTEX_POINT ( 'NONE', #47398 ) ;
#21761=ORIENTED_EDGE ( 'NONE', *, *, #64577, .F. ) ;
#21764=CARTESIAN_POINT ( 'NONE',  ( 11.14687500061451608, -2.746126346562642428, -4.756430356249999214 ) ) ;
#21780=CARTESIAN_POINT ( 'NONE',  ( 45.00000000000000000, 0.000000000000000000, 4.999999999999998224 ) ) ;
#21784=ADVANCED_FACE ( 'NONE', ( #19300 ), #64381, .T. ) ;
#21785=CARTESIAN_POINT ( 'NONE',  ( 20.78437500061451360, -2.746126346562646425, 4.756430356249996549 ) ) ;
#21788=CARTESIAN_POINT ( 'NONE',  ( 14.49375000122903145, -2.886751345948125991, -5.000000000000000000 ) ) ;
#21804=CARTESIAN_POINT ( 'NONE',  ( 7.509375000614516793, 2.746126346562645981, -4.756430356249997438 ) ) ;
#21823=CARTESIAN_POINT ( 'NONE',  ( 17.45625000122903003, 0.000000000000000000, 4.999999999999998224 ) ) ;
#21826=CARTESIAN_POINT ( 'NONE',  ( 16.47187500061452070, -5.492252693125287522, -1.008910452111647106E-15 ) ) ;
#21831=ORIENTED_EDGE ( 'NONE', *, *, #70383, .T. ) ;
#21861=CARTESIAN_POINT ( 'NONE',  ( 19.92187500061451644, 2.746126346562643317, 4.756430356249998326 ) ) ;
#21867=CARTESIAN_POINT ( 'NONE',  ( 19.72499999999999787, -4.330127018922194537, 2.499999999999995559 ) ) ;
#21870=CARTESIAN_POINT ( 'NONE',  ( 24.68437500061451573, 5.492252693125287522, 3.363034840372157021E-16 ) ) ;
#21871=CARTESIAN_POINT ( 'NONE',  ( 14.34375000122903465, -2.886751345948074920, 5.000000000000092371 ) ) ;
#21877=CARTESIAN_POINT ( 'NONE',  ( 26.85937500061451644, 2.746126346562645981, -4.756430356249997438 ) ) ;
#21879=CARTESIAN_POINT ( 'NONE',  ( 14.78437500061451537, 5.492252693125287522, 3.363034840372157021E-16 ) ) ;
#21880=AXIS2_PLACEMENT_3D ( 'NONE', #65263, #20927, #20188 ) ;
#21883=VERTEX_POINT ( 'NONE', #55141 ) ;
#21889=VECTOR ( 'NONE', #3382, 1000.000000000000000 ) ;
#21892=DIRECTION ( 'NONE',  ( -1.000000000000000000, -0.000000000000000000, -0.000000000000000000 ) ) ;
#21907=DIRECTION ( 'NONE',  ( -1.000000000000000000, -0.000000000000000000, -0.000000000000000000 ) ) ;
#21918=CARTESIAN_POINT ( 'NONE',  ( 23.97187500061451715, 2.746126346562643317, 4.756430356249998326 ) ) ;
#21920=CARTESIAN_POINT ( 'NONE',  ( 7.434375000614519280, -4.119189519843968306, 2.378215178124996054 ) ) ;
#21937=CARTESIAN_POINT ( 'NONE',  ( 19.06875000122903430, 2.886751345948129099, -4.999999999999998224 ) ) ;
#21941=ORIENTED_EDGE ( 'NONE', *, *, #63349, .T. ) ;
#21952=CARTESIAN_POINT ( 'NONE',  ( 26.33437500061451431, -4.119189519843968306, 2.378215178124996054 ) ) ;
#21957=EDGE_CURVE ( 'NONE', #59877, #38481, #68729, .T. ) ;
#21959=CARTESIAN_POINT ( 'NONE',  ( 27.82499999999999929, -4.330127018922194537, 2.499999999999995559 ) ) ;
#21967=CARTESIAN_POINT ( 'NONE',  ( 11.75625000122903430, -4.330127018922190985, -2.500000000000001332 ) ) ;
#21970=CARTESIAN_POINT ( 'NONE',  ( 19.69687500061451502, 4.119189519843966529, -2.378215178124998275 ) ) ;
#21973=EDGE_LOOP ( 'NONE', ( #45718, #51877, #15257, #68837 ) ) ;
#21982=CARTESIAN_POINT ( 'NONE',  ( 12.79687500061451466, -4.119189519843965641, -2.378215178125001383 ) ) ;
#21988=CARTESIAN_POINT ( 'NONE',  ( 21.05625000122903145, 0.000000000000000000, 4.999999999999998224 ) ) ;
#21994=DIRECTION ( 'NONE',  ( -1.000000000000000000, -0.000000000000000000, -0.000000000000000000 ) ) ;
#22009=CARTESIAN_POINT ( 'NONE',  ( 29.33437500061451431, -2.746126346562646425, 4.756430356249996549 ) ) ;
#22010=CARTESIAN_POINT ( 'NONE',  ( 16.09687500061452070, -2.746126346562642428, -4.756430356249999214 ) ) ;
#22026=CARTESIAN_POINT ( 'NONE',  ( 25.55625000122903501, 0.000000000000000000, 4.999999999999998224 ) ) ;
#22054=( BOUNDED_CURVE ( )  B_SPLINE_CURVE ( 2, ( #25077, #14727, #13996, #30995, #54270, #47620, #59055 ),
 .UNSPECIFIED., .F., .F. ) 
 B_SPLINE_CURVE_WITH_KNOTS ( ( 3, 2, 2, 3 ),
 ( 0.1900000000000000855, 0.1933333333333333848, 0.1966666666666667118, 0.2000000000000000389 ),
 .UNSPECIFIED. ) 
 CURVE ( )  GEOMETRIC_REPRESENTATION_ITEM ( )  RATIONAL_B_SPLINE_CURVE ( ( 0.9999999999999966693, 0.8660254037844420383, 1.000000000000000000, 0.8660254037844387076, 1.000000000000000000, 0.8660254037844375974, 1.000000000000001110 ) ) 
 REPRESENTATION_ITEM ( '' )  );
#22066=CARTESIAN_POINT ( 'NONE',  ( 28.93125000122903145, 6.123233995736764310E-16, -4.999999999999998224 ) ) ;
#22074=CARTESIAN_POINT ( 'NONE',  ( 21.83437500061451786, -2.746126346562642428, -4.756430356249999214 ) ) ;
#22083=CARTESIAN_POINT ( 'NONE',  ( 11.32500000000000107, 6.123233995736764310E-16, -4.999999999999998224 ) ) ;
#22091=CARTESIAN_POINT ( 'NONE',  ( 22.95937500061451431, 4.119189519843966529, -2.378215178124998275 ) ) ;
#22094=CARTESIAN_POINT ( 'NONE',  ( 10.93125000122903501, 6.123233995736764310E-16, -4.999999999999998224 ) ) ;
#22108=CARTESIAN_POINT ( 'NONE',  ( 25.78125000122903288, 6.123233995736764310E-16, -4.999999999999998224 ) ) ;
#22114=CARTESIAN_POINT ( 'NONE',  ( 7.584375000614516082, 5.824947211148865298E-16, -4.756430356249998326 ) ) ;
#22137=CARTESIAN_POINT ( 'NONE',  ( 11.82187500061451679, 2.746126346562643317, 4.756430356249998326 ) ) ;
#22141=ADVANCED_FACE ( 'NONE', ( #68402 ), #12603, .F. ) ;
#22157=CARTESIAN_POINT ( 'NONE',  ( 19.73437500061451289, 5.492252693125287522, 3.363034840372157021E-16 ) ) ;
#22160=CARTESIAN_POINT ( 'NONE',  ( 15.05625000122903323, 4.330127018922192761, -2.499999999999997780 ) ) ;
#22164=CARTESIAN_POINT ( 'NONE',  ( 27.07499999999999929, 6.123233995736764310E-16, -4.999999999999998224 ) ) ;
#22175=CARTESIAN_POINT ( 'NONE',  ( 8.034375000614515372, 5.492252693125287522, 3.363034840372157021E-16 ) ) ;
#22181=FACE_OUTER_BOUND ( 'NONE', #4557, .T. ) ;
#22194=CARTESIAN_POINT ( 'NONE',  ( 34.99999999999999289, 2.500000000000000000, -3.500000000000000000 ) ) ;
#22197=CARTESIAN_POINT ( 'NONE',  ( 17.63437500061451502, 4.119189519843966529, 2.378215178124999607 ) ) ;
#22228=CARTESIAN_POINT ( 'NONE',  ( 18.68437500061451928, -4.119189519843968306, 2.378215178124996054 ) ) ;
#22229=FACE_OUTER_BOUND ( 'NONE', #36458, .T. ) ;
#22234=CARTESIAN_POINT ( 'NONE',  ( 19.20000000000000284, 0.000000000000000000, 4.999999999999998224 ) ) ;
#22237=CARTESIAN_POINT ( 'NONE',  ( 21.52499999999999858, -4.330127018922194537, 2.499999999999995559 ) ) ;
#22238=CARTESIAN_POINT ( 'NONE',  ( 24.98437500061451289, -2.746126346562641984, -4.756430356249999214 ) ) ;
#22246=CARTESIAN_POINT ( 'NONE',  ( 28.24687500061451217, 4.119189519843966529, -2.378215178124998275 ) ) ;
#22248=CARTESIAN_POINT ( 'NONE',  ( 12.57187500061451502, 4.119189519843966529, 2.378215178124999607 ) ) ;
#22251=EDGE_LOOP ( 'NONE', ( #13184, #46559, #62828, #59139 ) ) ;
#22257=CARTESIAN_POINT ( 'NONE',  ( 45.00000000000000000, 0.000000000000000000, 0.000000000000000000 ) ) ;
#22281=CARTESIAN_POINT ( 'NONE',  ( 24.19687500061451502, -2.746126346562641984, -4.756430356249999214 ) ) ;
#22288=ORIENTED_EDGE ( 'NONE', *, *, #47314, .T. ) ;
#22299=CARTESIAN_POINT ( 'NONE',  ( 18.28125000122903288, 4.330127018922191873, 2.499999999999999556 ) ) ;
#22309=LINE ( 'NONE', #37479, #13224 ) ;
#22315=CARTESIAN_POINT ( 'NONE',  ( 24.87187500061451573, 2.746126346562643317, 4.756430356249998326 ) ) ;
#22321=CARTESIAN_POINT ( 'NONE',  ( 25.91250000000000142, 2.886751345948126879, 4.999999999999999112 ) ) ;
#22330=CARTESIAN_POINT ( 'NONE',  ( 12.73125000122903394, 6.123233995736764310E-16, -4.999999999999998224 ) ) ;
#22334=CARTESIAN_POINT ( 'NONE',  ( 20.40937500061451360, -5.492252693125287522, -1.008910452111647106E-15 ) ) ;
#22340=CARTESIAN_POINT ( 'NONE',  ( 45.00000000000000000, 0.000000000000000000, 0.000000000000000000 ) ) ;
#22345=CARTESIAN_POINT ( 'NONE',  ( 13.73437500061451644, -2.746126346562642428, -4.756430356249999214 ) ) ;
#22346=ORIENTED_EDGE ( 'NONE', *, *, #32675, .F. ) ;
#22366=CARTESIAN_POINT ( 'NONE',  ( 13.46249999999999858, -5.773502691896255534, -1.060575238724906372E-15 ) ) ;
#22368=CARTESIAN_POINT ( 'NONE',  ( 23.75625000122903074, 0.000000000000000000, 4.999999999999998224 ) ) ;
#22369=CARTESIAN_POINT ( 'NONE',  ( 15.53437500061451715, -4.119189519843968306, 2.378215178124996054 ) ) ;
#22380=CARTESIAN_POINT ( 'NONE',  ( 11.60625000122903216, 0.000000000000000000, 4.999999999999998224 ) ) ;
#22388=CARTESIAN_POINT ( 'NONE',  ( 25.21875000122903288, -5.773502691896255534, -1.060575238724906372E-15 ) ) ;
#22395=EDGE_CURVE ( 'NONE', #2080, #39643, #18202, .T. ) ;
#22404=EDGE_CURVE ( 'NONE', #46196, #39643, #46957, .T. ) ;
#22426=LINE ( 'NONE', #55689, #17215 ) ;
#22434=CARTESIAN_POINT ( 'NONE',  ( 20.44687500061451502, -4.119189519843965641, -2.378215178125001383 ) ) ;
#22441=LINE ( 'NONE', #38723, #41879 ) ;
#22444=CARTESIAN_POINT ( 'NONE',  ( 10.87500000000000000, 6.123233995736764310E-16, -4.999999999999998224 ) ) ;
#22449=DIRECTION ( 'NONE',  ( -1.000000000000000000, -0.000000000000000000, -0.000000000000000000 ) ) ;
#22450=CARTESIAN_POINT ( 'NONE',  ( 21.90937500061451715, -4.119189519843965641, -2.378215178125001383 ) ) ;
#22453=CYLINDRICAL_SURFACE ( 'NONE', #38402, 4.999999999999998224 ) ;
#22460=LINE ( 'NONE', #12825, #54852 ) ;
#22467=CARTESIAN_POINT ( 'NONE',  ( 18.48750000000000071, -2.886751345948126435, -5.000000000000000000 ) ) ;
#22474=EDGE_CURVE ( 'NONE', #14695, #24785, #70578, .T. ) ;
#22495=CARTESIAN_POINT ( 'NONE',  ( 11.25937500061451679, 4.119189519843966529, -2.378215178124998275 ) ) ;
#22505=CARTESIAN_POINT ( 'NONE',  ( 14.53125000122903288, 6.123233995736764310E-16, -4.999999999999998224 ) ) ;
#22506=CARTESIAN_POINT ( 'NONE',  ( 24.28125000122903288, -4.330127018922194537, 2.499999999999995559 ) ) ;
#22516=CARTESIAN_POINT ( 'NONE',  ( 17.59687500061451360, 0.000000000000000000, 4.756430356249998326 ) ) ;
#22519=CARTESIAN_POINT ( 'NONE',  ( 14.26875000122903536, 2.886751345948126879, 4.999999999999999112 ) ) ;
#22533=CARTESIAN_POINT ( 'NONE',  ( 7.246875000614514839, 0.000000000000000000, 4.756430356249998326 ) ) ;
#22536=( BOUNDED_CURVE ( )  B_SPLINE_CURVE ( 2, ( #19882, #2541, #49079, #20981, #30977, #70870, #64590 ),
 .UNSPECIFIED., .F., .F. ) 
 B_SPLINE_CURVE_WITH_KNOTS ( ( 3, 2, 2, 3 ),
 ( 0.2900000000000000355, 0.2933333333333333903, 0.2966666666666666896, 0.2999999999999999889 ),
 .UNSPECIFIED. ) 
 CURVE ( )  GEOMETRIC_REPRESENTATION_ITEM ( )  RATIONAL_B_SPLINE_CURVE ( ( 0.9999999999999977796, 0.8660254037844409281, 1.000000000000000000, 0.8660254037844387076, 1.000000000000000000, 0.8660254037844387076, 1.000000000000000000 ) ) 
 REPRESENTATION_ITEM ( '' )  );
#22539=CARTESIAN_POINT ( 'NONE',  ( 24.76875000122903003, -5.773502691896255534, -1.060575238724906372E-15 ) ) ;
#22541=CARTESIAN_POINT ( 'NONE',  ( 11.34375000122903465, -2.886751345948126435, -5.000000000000000000 ) ) ;
#22554=CARTESIAN_POINT ( 'NONE',  ( 13.84687500061451537, -2.746126346562641984, -4.756430356249999214 ) ) ;
#22569=ORIENTED_EDGE ( 'NONE', *, *, #5952, .F. ) ;
#22582=ORIENTED_EDGE ( 'NONE', *, *, #65502, .F. ) ;
#22585=CARTESIAN_POINT ( 'NONE',  ( 17.74687500061451928, -2.746126346562646425, 4.756430356249996549 ) ) ;
#22590=CARTESIAN_POINT ( 'NONE',  ( 19.04999999999999716, 4.330127018922192761, -2.499999999999997780 ) ) ;
#22594=CARTESIAN_POINT ( 'NONE',  ( 25.09687500061451360, 4.119189519843966529, -2.378215178124998275 ) ) ;
#22601=CARTESIAN_POINT ( 'NONE',  ( 27.45937500061451431, 2.746126346562643317, 4.756430356249998326 ) ) ;
#22603=CARTESIAN_POINT ( 'NONE',  ( 12.08437500061451608, 5.492252693125287522, 3.363034840372157021E-16 ) ) ;
#22608=CARTESIAN_POINT ( 'NONE',  ( 8.006250001229034297, 0.000000000000000000, 4.999999999999998224 ) ) ;
#22612=FACE_OUTER_BOUND ( 'NONE', #21973, .T. ) ;
#22638=CARTESIAN_POINT ( 'NONE',  ( 21.08437500061451786, 5.824947211148865298E-16, -4.756430356249998326 ) ) ;
#22646=CARTESIAN_POINT ( 'NONE',  ( 27.26249999999999929, 2.886751345948168623, 4.999999999999926281 ) ) ;
#22657=CARTESIAN_POINT ( 'NONE',  ( 15.91875000122903216, 2.886751345948129099, -4.999999999999998224 ) ) ;
#22659=CARTESIAN_POINT ( 'NONE',  ( 29.49375000122903145, 5.773502691896255534, 3.535250795749688401E-16 ) ) ;
#22666=LINE ( 'NONE', #39681, #49796 ) ;
#22672=CARTESIAN_POINT ( 'NONE',  ( 26.48437500061451644, 5.824947211148865298E-16, -4.756430356249998326 ) ) ;
#22676=AXIS2_PLACEMENT_3D ( 'NONE', #52561, #58810, #24834 ) ;
#22678=CARTESIAN_POINT ( 'NONE',  ( 26.13749999999999929, -2.886751345948125991, -5.000000000000000000 ) ) ;
#22686=CARTESIAN_POINT ( 'NONE',  ( 10.78125000122903288, -4.330127018922194537, 2.499999999999995559 ) ) ;
#22690=CARTESIAN_POINT ( 'NONE',  ( 20.97187500061451715, 5.824947211148865298E-16, -4.756430356249998326 ) ) ;
#22701=CARTESIAN_POINT ( 'NONE',  ( 12.49687500061451573, 4.119189519843966529, -2.378215178124998275 ) ) ;
#22702=EDGE_LOOP ( 'NONE', ( #16159, #63518, #52925 ) ) ;
#22707=ORIENTED_EDGE ( 'NONE', *, *, #22854, .T. ) ;
#22722=CARTESIAN_POINT ( 'NONE',  ( 13.35000000000000142, 0.000000000000000000, 4.999999999999998224 ) ) ;
#22725=CARTESIAN_POINT ( 'NONE',  ( 11.85937500061451644, 0.000000000000000000, 4.756430356249998326 ) ) ;
#22735=AXIS2_PLACEMENT_3D ( 'NONE', #65028, #54681, #14419 ) ;
#22744=LINE ( 'NONE', #6489, #39876 ) ;
#22745=CARTESIAN_POINT ( 'NONE',  ( 22.70625000122903003, 4.330127018922192761, -2.499999999999997780 ) ) ;
#22749=( BOUNDED_CURVE ( )  B_SPLINE_CURVE ( 2, ( #30341, #69148, #18138, #18507, #47327, #12253, #45884 ),
 .UNSPECIFIED., .F., .F. ) 
 B_SPLINE_CURVE_WITH_KNOTS ( ( 3, 2, 2, 3 ),
 ( 0.1400000000000000133, 0.1433333333333333404, 0.1466666666666666674, 0.1499999999999999944 ),
 .UNSPECIFIED. ) 
 CURVE ( )  GEOMETRIC_REPRESENTATION_ITEM ( )  RATIONAL_B_SPLINE_CURVE ( ( 1.000000000000000000, 0.8660254037844387076, 1.000000000000000000, 0.8660254037844387076, 1.000000000000000000, 0.8660254037844387076, 1.000000000000000000 ) ) 
 REPRESENTATION_ITEM ( '' )  );
#22752=CARTESIAN_POINT ( 'NONE',  ( 25.48125000122903216, 4.330127018922191873, 2.499999999999999556 ) ) ;
#22777=CARTESIAN_POINT ( 'NONE',  ( 12.95625000122903359, 0.000000000000000000, 4.999999999999998224 ) ) ;
#22790=CARTESIAN_POINT ( 'NONE',  ( 18.79687500061451289, 4.119189519843966529, -2.378215178124998275 ) ) ;
#22798=EDGE_CURVE ( 'NONE', #55986, #39550, #40043, .T. ) ;
#22800=VERTEX_POINT ( 'NONE', #60206 ) ;
#22806=CARTESIAN_POINT ( 'NONE',  ( 18.18750000000000355, 5.773502691896255534, 3.535250795749688401E-16 ) ) ;
#22807=CARTESIAN_POINT ( 'NONE',  ( 21.19687500061451502, 5.492252693125287522, 3.363034840372157021E-16 ) ) ;
#22810=CARTESIAN_POINT ( 'NONE',  ( 28.48125000122902861, 6.123233995736764310E-16, -4.999999999999998224 ) ) ;
#22839=ORIENTED_EDGE ( 'NONE', *, *, #35798, .F. ) ;
#22848=CARTESIAN_POINT ( 'NONE',  ( 9.496875000614517504, 5.492252693125287522, 3.363034840372157021E-16 ) ) ;
#22854=EDGE_CURVE ( 'NONE', #1482, #4916, #66492, .T. ) ;
#22867=CARTESIAN_POINT ( 'NONE',  ( 18.15937500061451715, -5.492252693125287522, -1.008910452111647106E-15 ) ) ;
#22870=CARTESIAN_POINT ( 'NONE',  ( 25.77187500061451431, -4.119189519843968306, 2.378215178124996054 ) ) ;
#22879=DIRECTION ( 'NONE',  ( -1.000000000000000000, -0.000000000000000000, -0.000000000000000000 ) ) ;
#22885=CARTESIAN_POINT ( 'NONE',  ( 28.73437500061451644, 5.824947211148865298E-16, -4.756430356249998326 ) ) ;
#22891=LINE ( 'NONE', #6652, #12453 ) ;
#22895=EDGE_LOOP ( 'NONE', ( #45166, #71877, #31334, #60784 ) ) ;
#22907=CARTESIAN_POINT ( 'NONE',  ( 13.62187500061451750, 2.746126346562643317, 4.756430356249998326 ) ) ;
#22912=ORIENTED_EDGE ( 'NONE', *, *, #50906, .F. ) ;
#22939=CARTESIAN_POINT ( 'NONE',  ( 17.44687500061451857, -2.746126346562642428, -4.756430356249999214 ) ) ;
#22942=AXIS2_PLACEMENT_3D ( 'NONE', #5991, #68779, #1546 ) ;
#22946=CARTESIAN_POINT ( 'NONE',  ( 20.43749999999999645, 5.773502691896255534, 3.535250795749688894E-16 ) ) ;
#22951=CARTESIAN_POINT ( 'NONE',  ( 25.88437500061451502, -2.746126346562641984, -4.756430356249999214 ) ) ;
#22955=( BOUNDED_CURVE ( )  B_SPLINE_CURVE ( 2, ( #61950, #11354, #56415, #28337, #7254, #30145, #34964 ),
 .UNSPECIFIED., .F., .F. ) 
 B_SPLINE_CURVE_WITH_KNOTS ( ( 3, 2, 2, 3 ),
 ( 0.07999999999999998779, 0.08333333333333331483, 0.08666666666666664187, 0.08999999999999996891 ),
 .UNSPECIFIED. ) 
 CURVE ( )  GEOMETRIC_REPRESENTATION_ITEM ( )  RATIONAL_B_SPLINE_CURVE ( ( 1.000000000000000666, 0.8660254037844381525, 1.000000000000000000, 0.8660254037844387076, 1.000000000000000000, 0.8660254037844398178, 0.9999999999999988898 ) ) 
 REPRESENTATION_ITEM ( '' )  );
#22958=CARTESIAN_POINT ( 'NONE',  ( 24.75937500061451502, 2.746126346562643317, 4.756430356249998326 ) ) ;
#22960=CARTESIAN_POINT ( 'NONE',  ( 10.99687500061451573, -4.119189519843965641, -2.378215178125001383 ) ) ;
#22965=CARTESIAN_POINT ( 'NONE',  ( 8.231250001229033941, 6.123233995736764310E-16, -4.999999999999998224 ) ) ;
#22973=CARTESIAN_POINT ( 'NONE',  ( 13.65937500061451537, -5.492252693125287522, -1.008910452111647106E-15 ) ) ;
#22983=CARTESIAN_POINT ( 'NONE',  ( 45.00000000000000000, 0.000000000000000000, 0.000000000000000000 ) ) ;
#22985=ORIENTED_EDGE ( 'NONE', *, *, #7045, .F. ) ;
#22995=CARTESIAN_POINT ( 'NONE',  ( 20.97187500061451715, -5.492252693125287522, -1.008910452111647106E-15 ) ) ;
#23017=CARTESIAN_POINT ( 'NONE',  ( 16.85625000122903572, 4.330127018922192761, -2.499999999999997780 ) ) ;
#23034=CARTESIAN_POINT ( 'NONE',  ( 25.17187500061451644, 2.746126346562645981, -4.756430356249997438 ) ) ;
#23039=CARTESIAN_POINT ( 'NONE',  ( 27.48749999999999716, -2.886751345948125991, -5.000000000000000000 ) ) ;
#23042=CARTESIAN_POINT ( 'NONE',  ( 9.975000000000001421, 6.123233995736764310E-16, -4.999999999999998224 ) ) ;
#23045=EDGE_CURVE ( 'NONE', #64545, #61968, #32480, .T. ) ;
#23046=CARTESIAN_POINT ( 'NONE',  ( 29.77499999999999858, 6.123233995736764310E-16, -4.999999999999998224 ) ) ;
#23049=CARTESIAN_POINT ( 'NONE',  ( 9.806250001229033231, 0.000000000000000000, 4.999999999999998224 ) ) ;
#23053=CARTESIAN_POINT ( 'NONE',  ( 18.68437500061452283, -2.746126346562641984, -4.756430356249999214 ) ) ;
#23055=AXIS2_PLACEMENT_3D ( 'NONE', #63312, #29343, #51875 ) ;
#23060=CARTESIAN_POINT ( 'NONE',  ( 27.89999999999999858, -4.330127018922190985, -2.500000000000001332 ) ) ;
#23065=CARTESIAN_POINT ( 'NONE',  ( 13.20937500061451431, -5.492252693125287522, -1.008910452111647106E-15 ) ) ;
#23066=ORIENTED_EDGE ( 'NONE', *, *, #73012, .F. ) ;
#23071=ORIENTED_EDGE ( 'NONE', *, *, #53045, .F. ) ;
#23084=CARTESIAN_POINT ( 'NONE',  ( 28.09687500061451715, -2.746126346562646425, 4.756430356249996549 ) ) ;
#23088=CARTESIAN_POINT ( 'NONE',  ( 12.00937500061451857, -4.119189519843965641, -2.378215178125001383 ) ) ;
#23100=CARTESIAN_POINT ( 'NONE',  ( 0.000000000000000000, 0.000000000000000000, 0.000000000000000000 ) ) ;
#23105=CARTESIAN_POINT ( 'NONE',  ( 23.98125000122903216, 6.123233995736764310E-16, -4.999999999999998224 ) ) ;
#23113=CARTESIAN_POINT ( 'NONE',  ( 25.36875000122903145, 2.886751345948087355, -5.000000000000071054 ) ) ;
#23115=EDGE_CURVE ( 'NONE', #72906, #42612, #22426, .T. ) ;
#23126=( BOUNDED_CURVE ( )  B_SPLINE_CURVE ( 2, ( #34143, #51149, #23060, #45615, #50788, #17512, #33789 ),
 .UNSPECIFIED., .F., .F. ) 
 B_SPLINE_CURVE_WITH_KNOTS ( ( 3, 2, 2, 3 ),
 ( 0.08999999999999996891, 0.09333333333333329596, 0.09666666666666662300, 0.09999999999999995004 ),
 .UNSPECIFIED. ) 
 CURVE ( )  GEOMETRIC_REPRESENTATION_ITEM ( )  RATIONAL_B_SPLINE_CURVE ( ( 1.000000000000001110, 0.8660254037844374864, 1.000000000000000000, 0.8660254037844387076, 1.000000000000000000, 0.8660254037844409281, 0.9999999999999977796 ) ) 
 REPRESENTATION_ITEM ( '' )  );
#23147=CARTESIAN_POINT ( 'NONE',  ( 29.08125000122903003, 4.330127018922191873, 2.499999999999999556 ) ) ;
#23152=ORIENTED_EDGE ( 'NONE', *, *, #59010, .F. ) ;
#23155=CARTESIAN_POINT ( 'NONE',  ( 18.00937500061451502, 2.746126346562643317, 4.756430356249998326 ) ) ;
#23163=ORIENTED_EDGE ( 'NONE', *, *, #13474, .F. ) ;
#23171=CARTESIAN_POINT ( 'NONE',  ( 21.08437500061451786, 5.824947211148865298E-16, -4.756430356249998326 ) ) ;
#23182=ORIENTED_EDGE ( 'NONE', *, *, #15334, .T. ) ;
#23192=CARTESIAN_POINT ( 'NONE',  ( 7.846875000614518036, -2.746126346562646425, 4.756430356249996549 ) ) ;
#23196=( BOUNDED_CURVE ( )  B_SPLINE_CURVE ( 2, ( #35708, #13529, #7635, #41267, #24984, #30173, #13905 ),
 .UNSPECIFIED., .F., .F. ) 
 B_SPLINE_CURVE_WITH_KNOTS ( ( 3, 2, 2, 3 ),
 ( 0.9400000000000001688, 0.9433333333333335791, 0.9466666666666667673, 0.9500000000000000666 ),
 .UNSPECIFIED. ) 
 CURVE ( )  GEOMETRIC_REPRESENTATION_ITEM ( )  RATIONAL_B_SPLINE_CURVE ( ( 0.9999999999999911182, 0.8660254037844475894, 1.000000000000000000, 0.8660254037844387076, 1.000000000000000000, 0.8660254037844342667, 1.000000000000004441 ) ) 
 REPRESENTATION_ITEM ( '' )  );
#23215=CARTESIAN_POINT ( 'NONE',  ( 8.746875000614515727, -2.746126346562646425, 4.756430356249996549 ) ) ;
#23238=CARTESIAN_POINT ( 'NONE',  ( 17.82187500061451502, 5.824947211148865298E-16, -4.756430356249998326 ) ) ;
#23241=CARTESIAN_POINT ( 'NONE',  ( 26.14687500061451431, 0.000000000000000000, 4.756430356249998326 ) ) ;
#23249=DIRECTION ( 'NONE',  ( 1.000000000000000000, 0.000000000000000000, 0.000000000000000000 ) ) ;
#23255=CARTESIAN_POINT ( 'NONE',  ( 28.35937500061451289, 4.119189519843966529, -2.378215178124998275 ) ) ;
#23261=LINE ( 'NONE', #39914, #6554 ) ;
#23273=CARTESIAN_POINT ( 'NONE',  ( 14.89687500061451786, 5.492252693125287522, 3.363034840372157021E-16 ) ) ;
#23281=EDGE_CURVE ( 'NONE', #31980, #32613, #22955, .T. ) ;
#23305=CARTESIAN_POINT ( 'NONE',  ( 17.03437500061451715, 5.824947211148865298E-16, -4.756430356249998326 ) ) ;
#23312=CARTESIAN_POINT ( 'NONE',  ( 16.72500000000000142, 6.123233995736764310E-16, -4.999999999999998224 ) ) ;
#23316=CARTESIAN_POINT ( 'NONE',  ( 26.78437500061451360, -2.746126346562641984, -4.756430356249999214 ) ) ;
#23321=EDGE_CURVE ( 'NONE', #21751, #71509, #17954, .T. ) ;
#23324=CARTESIAN_POINT ( 'NONE',  ( 23.82187500061451502, 4.119189519843966529, 2.378215178124999607 ) ) ;
#23326=CARTESIAN_POINT ( 'NONE',  ( 10.28437500061451715, 5.492252693125287522, 3.363034840372157021E-16 ) ) ;
#23331=CARTESIAN_POINT ( 'NONE',  ( 21.73125000122903216, 6.123233995736764310E-16, -4.999999999999998224 ) ) ;
#23334=VECTOR ( 'NONE', #32395, 1000.000000000000000 ) ;
#23339=CARTESIAN_POINT ( 'NONE',  ( 11.63437500061451502, 5.492252693125287522, 3.363034840372157021E-16 ) ) ;
#23342=( BOUNDED_CURVE ( )  B_SPLINE_CURVE ( 2, ( #34371, #17734, #11852, #12570, #35104, #52462, #52823 ),
 .UNSPECIFIED., .F., .F. ) 
 B_SPLINE_CURVE_WITH_KNOTS ( ( 3, 2, 2, 3 ),
 ( 0.009999999999999979391, 0.01333333333333330643, 0.01666666666666663174, 0.01999999999999995878 ),
 .UNSPECIFIED. ) 
 CURVE ( )  GEOMETRIC_REPRESENTATION_ITEM ( )  RATIONAL_B_SPLINE_CURVE ( ( 1.000000000000000888, 0.8660254037844378194, 1.000000000000000000, 0.8660254037844387076, 1.000000000000000000, 0.8660254037844403729, 0.9999999999999983347 ) ) 
 REPRESENTATION_ITEM ( '' )  );
#23351=VERTEX_POINT ( 'NONE', #8339 ) ;
#23360=CARTESIAN_POINT ( 'NONE',  ( 22.54687500061451644, 5.492252693125287522, 3.363034840372157021E-16 ) ) ;
#23367=ORIENTED_EDGE ( 'NONE', *, *, #63206, .F. ) ;
#23380=CARTESIAN_POINT ( 'NONE',  ( 16.10625000122903216, 0.000000000000000000, 4.999999999999998224 ) ) ;
#23396=CARTESIAN_POINT ( 'NONE',  ( 24.08437500061451786, -4.119189519843968306, 2.378215178124996054 ) ) ;
#23402=CARTESIAN_POINT ( 'NONE',  ( 24.75000000000000000, -4.330127018922190985, -2.500000000000001332 ) ) ;
#23412=CARTESIAN_POINT ( 'NONE',  ( 9.618750001229031454, 2.886751345948129099, -4.999999999999998224 ) ) ;
#23416=CARTESIAN_POINT ( 'NONE',  ( 19.02187500061451431, -4.119189519843968306, 2.378215178124996054 ) ) ;
#23423=CARTESIAN_POINT ( 'NONE',  ( 20.32499999999999929, 6.123233995736764310E-16, -4.999999999999998224 ) ) ;
#23428=CARTESIAN_POINT ( 'NONE',  ( 10.02187500061451431, -4.119189519843968306, 2.378215178124996054 ) ) ;
#23449=CARTESIAN_POINT ( 'NONE',  ( 28.77187500061451431, 2.746126346562645981, -4.756430356249997438 ) ) ;
#23452=CARTESIAN_POINT ( 'NONE',  ( 28.20937500061451431, 2.746126346562645981, -4.756430356249997438 ) ) ;
#23454=CARTESIAN_POINT ( 'NONE',  ( 13.20937500061451786, 0.000000000000000000, 4.756430356249998326 ) ) ;
#23471=CARTESIAN_POINT ( 'NONE',  ( 22.81875000122903074, 2.886751345948126879, 4.999999999999999112 ) ) ;
#23495=CARTESIAN_POINT ( 'NONE',  ( 22.29375000122903216, 5.773502691896255534, 3.535250795749688401E-16 ) ) ;
#23509=CARTESIAN_POINT ( 'NONE',  ( 11.17500000000000071, -4.330127018922194537, 2.499999999999995559 ) ) ;
#23511=VERTEX_POINT ( 'NONE', #29426 ) ;
#23517=CARTESIAN_POINT ( 'NONE',  ( 19.73437500061451289, 5.492252693125287522, 3.363034840372157021E-16 ) ) ;
#23534=CARTESIAN_POINT ( 'NONE',  ( 20.37187500061451573, 2.746126346562643317, 4.756430356249998326 ) ) ;
#23551=DIRECTION ( 'NONE',  ( -1.000000000000000000, -0.000000000000000000, -0.000000000000000000 ) ) ;
#23553=DIRECTION ( 'NONE',  ( -0.000000000000000000, -0.000000000000000000, -1.000000000000000000 ) ) ;
#23556=EDGE_CURVE ( 'NONE', #18169, #9094, #56005, .T. ) ;
#23558=CARTESIAN_POINT ( 'NONE',  ( 7.696875000614516793, 5.492252693125287522, 3.363034840372157021E-16 ) ) ;
#23570=VERTEX_POINT ( 'NONE', #18678 ) ;
#23571=EDGE_LOOP ( 'NONE', ( #32221, #47998, #9586, #64772 ) ) ;
#23582=CARTESIAN_POINT ( 'NONE',  ( 8.784375000614518925, -4.119189519843968306, 2.378215178124996054 ) ) ;
#23583=CARTESIAN_POINT ( 'NONE',  ( 11.15625000122903288, 0.000000000000000000, 4.999999999999998224 ) ) ;
#23592=FACE_OUTER_BOUND ( 'NONE', #7733, .T. ) ;
#23602=CARTESIAN_POINT ( 'NONE',  ( 16.73437500061451644, -2.746126346562646425, 4.756430356249996549 ) ) ;
#23605=CARTESIAN_POINT ( 'NONE',  ( 27.23437500061450933, -2.746126346562642428, -4.756430356249999214 ) ) ;
#23609=CARTESIAN_POINT ( 'NONE',  ( 28.87499999999999645, 6.123233995736764310E-16, -4.999999999999998224 ) ) ;
#23611=CARTESIAN_POINT ( 'NONE',  ( 28.10625000122902861, 4.330127018922192761, -2.499999999999997780 ) ) ;
#23618=CARTESIAN_POINT ( 'NONE',  ( 26.59687500061451360, 5.492252693125287522, 3.363034840372157021E-16 ) ) ;
#23625=CARTESIAN_POINT ( 'NONE',  ( 45.00000000000000000, 0.000000000000000000, 0.000000000000000000 ) ) ;
#23637=CARTESIAN_POINT ( 'NONE',  ( 14.48437500061451821, 4.119189519843966529, 2.378215178124999607 ) ) ;
#23651=CARTESIAN_POINT ( 'NONE',  ( 11.38125000122903252, 6.123233995736764310E-16, -4.999999999999998224 ) ) ;
#23652=ORIENTED_EDGE ( 'NONE', *, *, #17853, .F. ) ;
#23668=CARTESIAN_POINT ( 'NONE',  ( 16.13437500061451502, 5.824947211148865298E-16, -4.756430356249998326 ) ) ;
#23674=CARTESIAN_POINT ( 'NONE',  ( 18.11250000000000071, 2.886751345948129099, -4.999999999999998224 ) ) ;
#23677=CARTESIAN_POINT ( 'NONE',  ( 45.00000000000000000, 0.000000000000000000, 0.000000000000000000 ) ) ;
#23678=CARTESIAN_POINT ( 'NONE',  ( 23.10937500061451644, -5.492252693125287522, -1.008910452111647106E-15 ) ) ;
#23684=CARTESIAN_POINT ( 'NONE',  ( 26.07187500061451146, 4.119189519843966529, 2.378215178124999607 ) ) ;
#23686=CARTESIAN_POINT ( 'NONE',  ( 10.02187500061451431, -4.119189519843968306, 2.378215178124996054 ) ) ;
#23689=ORIENTED_EDGE ( 'NONE', *, *, #49936, .F. ) ;
#23696=ORIENTED_EDGE ( 'NONE', *, *, #30226, .T. ) ;
#23698=CARTESIAN_POINT ( 'NONE',  ( 10.77187500061451608, 4.119189519843966529, 2.378215178124999607 ) ) ;
#23715=CARTESIAN_POINT ( 'NONE',  ( 12.28125000122903110, 6.123233995736764310E-16, -4.999999999999998224 ) ) ;
#23717=CARTESIAN_POINT ( 'NONE',  ( 21.57187500061451502, 2.746126346562645981, -4.756430356249997438 ) ) ;
#23734=CARTESIAN_POINT ( 'NONE',  ( 28.46249999999999858, 2.886751345948129099, -4.999999999999997335 ) ) ;
#23737=CARTESIAN_POINT ( 'NONE',  ( 15.76875000122903181, -5.773502691896255534, -1.060575238724906372E-15 ) ) ;
#23749=ORIENTED_EDGE ( 'NONE', *, *, #54007, .F. ) ;
#23753=CARTESIAN_POINT ( 'NONE',  ( 24.49687500061451573, -2.746126346562646425, 4.756430356249996549 ) ) ;
#23758=CARTESIAN_POINT ( 'NONE',  ( 24.67500000000000071, -4.330127018922194537, 2.499999999999995559 ) ) ;
#23760=CARTESIAN_POINT ( 'NONE',  ( 12.50625000122903430, 0.000000000000000000, 4.999999999999998224 ) ) ;
#23761=FACE_OUTER_BOUND ( 'NONE', #8853, .T. ) ;
#23765=AXIS2_PLACEMENT_3D ( 'NONE', #23100, #68190, #46012 ) ;
#23766=CARTESIAN_POINT ( 'NONE',  ( 23.04375000122903216, -2.886751345948153968, -4.999999999999952038 ) ) ;
#23769=CARTESIAN_POINT ( 'NONE',  ( 8.456250001229033586, 0.000000000000000000, 4.999999999999998224 ) ) ;
#23772=CARTESIAN_POINT ( 'NONE',  ( 17.59687500061451360, 0.000000000000000000, 4.756430356249998326 ) ) ;
#23784=CARTESIAN_POINT ( 'NONE',  ( 10.95937500061451431, -5.492252693125287522, -1.008910452111647106E-15 ) ) ;
#23785=ORIENTED_EDGE ( 'NONE', *, *, #14641, .T. ) ;
#23791=ORIENTED_EDGE ( 'NONE', *, *, #70383, .F. ) ;
#23792=CARTESIAN_POINT ( 'NONE',  ( 19.87500000000000000, 6.123233995736764310E-16, -4.999999999999998224 ) ) ;
#23798=CARTESIAN_POINT ( 'NONE',  ( 9.562500000000001776, 2.886751345948129099, -4.999999999999998224 ) ) ;
#23807=CARTESIAN_POINT ( 'NONE',  ( 28.73437500061451644, 5.824947211148865298E-16, -4.756430356249998326 ) ) ;
#23809=CARTESIAN_POINT ( 'NONE',  ( 27.87187500061451217, 4.119189519843966529, 2.378215178124999607 ) ) ;
#23810=CARTESIAN_POINT ( 'NONE',  ( 12.83437500061451786, -4.119189519843968306, 2.378215178124996054 ) ) ;
#23826=CARTESIAN_POINT ( 'NONE',  ( 24.58125000122903003, 4.330127018922191873, 2.499999999999999556 ) ) ;
#23829=ORIENTED_EDGE ( 'NONE', *, *, #55670, .F. ) ;
#23854=CARTESIAN_POINT ( 'NONE',  ( 22.36875000122903145, 2.886751345948098901, 5.000000000000047073 ) ) ;
#23862=CARTESIAN_POINT ( 'NONE',  ( 18.00000000000000355, -4.330127018922190985, -2.500000000000001332 ) ) ;
#23880=CARTESIAN_POINT ( 'NONE',  ( 20.10937500061451644, 2.746126346562645981, -4.756430356249997438 ) ) ;
#23896=CARTESIAN_POINT ( 'NONE',  ( 18.07499999999999929, 6.123233995736764310E-16, -4.999999999999998224 ) ) ;
#23897=CARTESIAN_POINT ( 'NONE',  ( 19.73437500061451644, 5.824947211148865298E-16, -4.756430356249998326 ) ) ;
#23915=CARTESIAN_POINT ( 'NONE',  ( 20.94375000122902719, 5.773502691896255534, 3.535250795749688401E-16 ) ) ;
#23940=CARTESIAN_POINT ( 'NONE',  ( 10.02187500061451964, 2.746126346562643317, 4.756430356249998326 ) ) ;
#23941=CARTESIAN_POINT ( 'NONE',  ( 26.90625000122902932, 0.000000000000000000, 4.999999999999998224 ) ) ;
#23942=DIRECTION ( 'NONE',  ( 0.000000000000000000, 0.000000000000000000, 1.000000000000000000 ) ) ;
#23949=CYLINDRICAL_SURFACE ( 'NONE', #58620, 4.999999999999998224 ) ;
#23951=CARTESIAN_POINT ( 'NONE',  ( 9.637499999999999289, 5.773502691896255534, 3.535250795749688401E-16 ) ) ;
#23961=CARTESIAN_POINT ( 'NONE',  ( 16.50937500061451502, 2.746126346562645981, -4.756430356249997438 ) ) ;
#23964=CARTESIAN_POINT ( 'NONE',  ( 26.78437500061451715, -2.746126346562642428, -4.756430356249999214 ) ) ;
#23971=CARTESIAN_POINT ( 'NONE',  ( 21.80625000122903145, 4.330127018922192761, -2.499999999999997780 ) ) ;
#23979=CARTESIAN_POINT ( 'NONE',  ( 27.23437500061451644, -4.119189519843968306, 2.378215178124996054 ) ) ;
#23998=CARTESIAN_POINT ( 'NONE',  ( 14.97187500061451892, 2.746126346562643317, 4.756430356249998326 ) ) ;
#24010=VERTEX_POINT ( 'NONE', #34055 ) ;
#24022=VERTEX_POINT ( 'NONE', #46239 ) ;
#24027=CARTESIAN_POINT ( 'NONE',  ( 15.53437500061451715, -4.119189519843968306, 2.378215178124996054 ) ) ;
#24035=CARTESIAN_POINT ( 'NONE',  ( 18.56250000000000000, 2.886751345948129099, -4.999999999999998224 ) ) ;
#24039=CARTESIAN_POINT ( 'NONE',  ( 23.63437500061451502, -2.746126346562641984, -4.756430356249999214 ) ) ;
#24042=CARTESIAN_POINT ( 'NONE',  ( 26.55000000000000071, -4.330127018922190985, -2.500000000000001332 ) ) ;
#24046=ADVANCED_FACE ( 'NONE', ( #56595 ), #12970, .T. ) ;
#24049=CARTESIAN_POINT ( 'NONE',  ( 24.23437500061451644, 5.492252693125287522, 3.363034840372157021E-16 ) ) ;
#24051=CARTESIAN_POINT ( 'NONE',  ( 11.93437500061451750, -2.746126346562641984, -4.756430356249999214 ) ) ;
#24056=CARTESIAN_POINT ( 'NONE',  ( 8.043750001229032165, -2.886751345948130876, 4.999999999999996447 ) ) ;
#24059=CARTESIAN_POINT ( 'NONE',  ( 29.73749999999999716, -2.886751345948115777, -5.000000000000017764 ) ) ;
#24060=CARTESIAN_POINT ( 'NONE',  ( 15.82499999999999929, 6.123233995736764310E-16, -4.999999999999998224 ) ) ;
#24063=CARTESIAN_POINT ( 'NONE',  ( 12.27187500061451608, -4.119189519843968306, 2.378215178124996054 ) ) ;
#24066=EDGE_CURVE ( 'NONE', #29126, #23351, #56245, .T. ) ;
#24071=CARTESIAN_POINT ( 'NONE',  ( 45.00000000000000000, 0.000000000000000000, 0.000000000000000000 ) ) ;
#24080=CARTESIAN_POINT ( 'NONE',  ( 7.500000000000000000, 0.000000000000000000, 4.999999999999998224 ) ) ;
#24082=CARTESIAN_POINT ( 'NONE',  ( 21.49687500061451573, -2.746126346562641984, -4.756430356249999214 ) ) ;
#24100=CARTESIAN_POINT ( 'NONE',  ( 21.33749999999999858, 5.773502691896255534, 3.535250795749688401E-16 ) ) ;
#24104=CARTESIAN_POINT ( 'NONE',  ( 10.03125000122903288, 6.123233995736764310E-16, -4.999999999999998224 ) ) ;
#24114=EDGE_LOOP ( 'NONE', ( #60862, #38345, #56700, #23689 ) ) ;
#24118=CARTESIAN_POINT ( 'NONE',  ( 23.67187500061451999, -5.492252693125287522, -1.008910452111647106E-15 ) ) ;
#24121=CARTESIAN_POINT ( 'NONE',  ( 29.21249999999999858, -5.773502691896255534, -1.060575238724906372E-15 ) ) ;
#24124=CARTESIAN_POINT ( 'NONE',  ( 25.38749999999999929, 5.773502691896255534, 3.535250795749688894E-16 ) ) ;
#24134=CARTESIAN_POINT ( 'NONE',  ( 8.343750001229034652, 5.773502691896255534, 3.535250795749688894E-16 ) ) ;
#24136=CARTESIAN_POINT ( 'NONE',  ( 17.25937500061451502, -5.492252693125287522, -1.008910452111647106E-15 ) ) ;
#24147=CARTESIAN_POINT ( 'NONE',  ( 10.69687500061451679, 4.119189519843966529, -2.378215178124998275 ) ) ;
#24161=CARTESIAN_POINT ( 'NONE',  ( 10.08749999999999858, 5.773502691896255534, 3.535250795749688894E-16 ) ) ;
#24165=ORIENTED_EDGE ( 'NONE', *, *, #56240, .F. ) ;
#24172=CARTESIAN_POINT ( 'NONE',  ( 28.62187500061451217, 5.824947211148865298E-16, -4.756430356249998326 ) ) ;
#24173=CARTESIAN_POINT ( 'NONE',  ( 11.97187500061451892, -5.492252693125287522, -1.008910452111647106E-15 ) ) ;
#24181=FACE_OUTER_BOUND ( 'NONE', #20140, .T. ) ;
#24188=CARTESIAN_POINT ( 'NONE',  ( 24.61875000122903501, 2.886751345948126879, 4.999999999999999112 ) ) ;
#24191=ORIENTED_EDGE ( 'NONE', *, *, #65091, .F. ) ;
#24198=EDGE_CURVE ( 'NONE', #65361, #25555, #25332, .T. ) ;
#24212=AXIS2_PLACEMENT_3D ( 'NONE', #42382, #32385, #13930 ) ;
#24214=VECTOR ( 'NONE', #14266, 1000.000000000000000 ) ;
#24216=CARTESIAN_POINT ( 'NONE',  ( 22.21875000122903288, 2.886751345948101122, -5.000000000000046185 ) ) ;
#24217=EDGE_CURVE ( 'NONE', #34631, #10555, #65473, .T. ) ;
#24221=CARTESIAN_POINT ( 'NONE',  ( 23.85000000000000142, -4.330127018922190985, -2.500000000000001332 ) ) ;
#24228=VERTEX_POINT ( 'NONE', #23331 ) ;
#24229=DIRECTION ( 'NONE',  ( -1.000000000000000000, -0.000000000000000000, -0.000000000000000000 ) ) ;
#24243=CARTESIAN_POINT ( 'NONE',  ( 18.42187500061451644, 4.119189519843966529, 2.378215178124999607 ) ) ;
#24262=CARTESIAN_POINT ( 'NONE',  ( 19.32187500061451857, 2.746126346562645981, -4.756430356249997438 ) ) ;
#24271=( BOUNDED_CURVE ( )  B_SPLINE_CURVE ( 2, ( #4627, #27157, #38971, #60381, #16055, #72219, #61129 ),
 .UNSPECIFIED., .F., .F. ) 
 B_SPLINE_CURVE_WITH_KNOTS ( ( 3, 2, 2, 3 ),
 ( 0.09999999999999995004, 0.1033333333333332771, 0.1066666666666666041, 0.1099999999999999312 ),
 .UNSPECIFIED. ) 
 CURVE ( )  GEOMETRIC_REPRESENTATION_ITEM ( )  RATIONAL_B_SPLINE_CURVE ( ( 1.000000000000002220, 0.8660254037844364872, 1.000000000000000000, 0.8660254037844387076, 1.000000000000000000, 0.8660254037844414832, 0.9999999999999972244 ) ) 
 REPRESENTATION_ITEM ( '' )  );
#24274=DIRECTION ( 'NONE',  ( 0.000000000000000000, 0.000000000000000000, 1.000000000000000000 ) ) ;
#24277=VECTOR ( 'NONE', #13989, 1000.000000000000000 ) ;
#24284=CARTESIAN_POINT ( 'NONE',  ( 8.474999999999999645, -4.330127018922194537, 2.499999999999995559 ) ) ;
#24286=CARTESIAN_POINT ( 'NONE',  ( 14.84999999999999964, -4.330127018922190985, -2.500000000000001332 ) ) ;
#24303=EDGE_CURVE ( 'NONE', #18738, #47145, #70211, .T. ) ;
#24307=CARTESIAN_POINT ( 'NONE',  ( 27.84375000122903288, -2.886751345948137093, 4.999999999999984901 ) ) ;
#24309=CARTESIAN_POINT ( 'NONE',  ( 9.796875000614519990, -2.746126346562642428, -4.756430356249999214 ) ) ;
#24316=CARTESIAN_POINT ( 'NONE',  ( 45.00000000000000000, 0.000000000000000000, 0.000000000000000000 ) ) ;
#24325=CARTESIAN_POINT ( 'NONE',  ( 14.40937500061451537, 2.746126346562643317, 4.756430356249998326 ) ) ;
#24328=CARTESIAN_POINT ( 'NONE',  ( 25.65937500061451360, 2.746126346562643317, 4.756430356249998326 ) ) ;
#24344=CARTESIAN_POINT ( 'NONE',  ( 27.87187500061451573, 2.746126346562645981, -4.756430356249997438 ) ) ;
#24348=CARTESIAN_POINT ( 'NONE',  ( 45.00000000000000000, 0.000000000000000000, 4.999999999999998224 ) ) ;
#24353=AXIS2_PLACEMENT_3D ( 'NONE', #66488, #15867, #38415 ) ;
#24363=CARTESIAN_POINT ( 'NONE',  ( 11.55937500061451928, -4.119189519843965641, -2.378215178125001383 ) ) ;
#24394=CARTESIAN_POINT ( 'NONE',  ( 16.17187500061451644, 2.746126346562645981, -4.756430356249997438 ) ) ;
#24400=CARTESIAN_POINT ( 'NONE',  ( 16.38749999999999929, 5.773502691896255534, 3.535250795749688894E-16 ) ) ;
#24404=CARTESIAN_POINT ( 'NONE',  ( 23.18437500061451573, -2.746126346562641984, -4.756430356249999214 ) ) ;
#24405=CARTESIAN_POINT ( 'NONE',  ( 26.17500000000000071, 6.123233995736764310E-16, -4.999999999999998224 ) ) ;
#24412=CARTESIAN_POINT ( 'NONE',  ( 25.99687500061451573, 4.119189519843966529, -2.378215178124998275 ) ) ;
#24414=CARTESIAN_POINT ( 'NONE',  ( 9.459375000614519635, 2.746126346562643317, 4.756430356249998326 ) ) ;
#24417=VERTEX_POINT ( 'NONE', #59121 ) ;
#24422=CARTESIAN_POINT ( 'NONE',  ( 19.20000000000000284, 0.000000000000000000, 4.999999999999998224 ) ) ;
#24426=CARTESIAN_POINT ( 'NONE',  ( 10.65937500061451892, 2.746126346562645981, -4.756430356249997438 ) ) ;
#24445=CARTESIAN_POINT ( 'NONE',  ( 19.28437500061451360, 5.824947211148865298E-16, -4.756430356249998326 ) ) ;
#24462=VERTEX_POINT ( 'NONE', #69504 ) ;
#24464=DIRECTION ( 'NONE',  ( 0.000000000000000000, 0.000000000000000000, 1.000000000000000000 ) ) ;
#24468=CARTESIAN_POINT ( 'NONE',  ( 45.00000000000000000, 0.000000000000000000, 4.999999999999998224 ) ) ;
#24473=( BOUNDED_CURVE ( )  B_SPLINE_CURVE ( 2, ( #54323, #70573, #14045, #2975, #8150, #31041, #30321 ),
 .UNSPECIFIED., .F., .F. ) 
 B_SPLINE_CURVE_WITH_KNOTS ( ( 3, 2, 2, 3 ),
 ( 0.2300000000000000100, 0.2333333333333333370, 0.2366666666666666363, 0.2399999999999999634 ),
 .UNSPECIFIED. ) 
 CURVE ( )  GEOMETRIC_REPRESENTATION_ITEM ( )  RATIONAL_B_SPLINE_CURVE ( ( 1.000000000000000000, 0.8660254037844387076, 1.000000000000000000, 0.8660254037844387076, 1.000000000000000000, 0.8660254037844398178, 0.9999999999999988898 ) ) 
 REPRESENTATION_ITEM ( '' )  );
#24484=CARTESIAN_POINT ( 'NONE',  ( 23.03437500061451715, 4.119189519843966529, 2.378215178124999607 ) ) ;
#24487=( BOUNDED_CURVE ( )  B_SPLINE_CURVE ( 2, ( #70023, #71121, #25317, #31228, #42319, #8696, #7968 ),
 .UNSPECIFIED., .F., .T. ) 
 B_SPLINE_CURVE_WITH_KNOTS ( ( 3, 2, 2, 3 ),
 ( 0.5800000000000000711, 0.5833333333333334814, 0.5866666666666666696, 0.5899999999999999689 ),
 .UNSPECIFIED. ) 
 CURVE ( )  GEOMETRIC_REPRESENTATION_ITEM ( )  RATIONAL_B_SPLINE_CURVE ( ( 0.9999999999999955591, 0.8660254037844431485, 1.000000000000000000, 0.8660254037844387076, 1.000000000000000000, 0.8660254037844387076, 1.000000000000000000 ) ) 
 REPRESENTATION_ITEM ( '' )  );
#24490=CARTESIAN_POINT ( 'NONE',  ( 24.14999999999999858, 0.000000000000000000, 4.999999999999998224 ) ) ;
#24493=CARTESIAN_POINT ( 'NONE',  ( 12.76875000122903536, 2.886751345948129099, -4.999999999999997335 ) ) ;
#24495=LINE ( 'NONE', #2335, #9229 ) ;
#24500=CARTESIAN_POINT ( 'NONE',  ( 8.831250001229033586, 4.330127018922191873, 2.499999999999999556 ) ) ;
#24503=CARTESIAN_POINT ( 'NONE',  ( 18.98437500061451289, -2.746126346562646425, 4.756430356249996549 ) ) ;
#24506=VERTEX_POINT ( 'NONE', #16253 ) ;
#24510=LINE ( 'NONE', #57035, #35690 ) ;
#24515=CARTESIAN_POINT ( 'NONE',  ( 9.646875000614514306, -4.119189519843965641, -2.378215178125001383 ) ) ;
#24516=ORIENTED_EDGE ( 'NONE', *, *, #48942, .F. ) ;
#24521=VERTEX_POINT ( 'NONE', #37694 ) ;
#24526=CARTESIAN_POINT ( 'NONE',  ( 27.42187500061451289, 4.119189519843966529, 2.378215178124999607 ) ) ;
#24529=CARTESIAN_POINT ( 'NONE',  ( 9.000000000000001776, -4.330127018922190985, -2.500000000000001332 ) ) ;
#24537=CARTESIAN_POINT ( 'NONE',  ( 29.70937500061451431, 4.119189519843966529, -2.378215178124998275 ) ) ;
#24539=CARTESIAN_POINT ( 'NONE',  ( 27.83437500061451075, 5.492252693125287522, 3.363034840372157021E-16 ) ) ;
#24540=CARTESIAN_POINT ( 'NONE',  ( 9.496875000614517504, 5.492252693125287522, 3.363034840372157021E-16 ) ) ;
#24554=CARTESIAN_POINT ( 'NONE',  ( 20.79375000122902861, -2.886751345948125991, -5.000000000000000000 ) ) ;
#24562=CARTESIAN_POINT ( 'NONE',  ( 23.30625000122903145, 0.000000000000000000, 4.999999999999998224 ) ) ;
#24577=CARTESIAN_POINT ( 'NONE',  ( 45.00000000000000000, 0.000000000000000000, 0.000000000000000000 ) ) ;
#24581=DIRECTION ( 'NONE',  ( -1.000000000000000000, -0.000000000000000000, -0.000000000000000000 ) ) ;
#24585=CARTESIAN_POINT ( 'NONE',  ( 7.762499999999999289, 2.886751345948018077, -5.000000000000190070 ) ) ;
#24604=CARTESIAN_POINT ( 'NONE',  ( 16.99687500061451573, 4.119189519843966529, -2.378215178124998275 ) ) ;
#24621=DIRECTION ( 'NONE',  ( -1.000000000000000000, -0.000000000000000000, -0.000000000000000000 ) ) ;
#24623=DIRECTION ( 'NONE',  ( -1.000000000000000000, -0.000000000000000000, -0.000000000000000000 ) ) ;
#24624=CARTESIAN_POINT ( 'NONE',  ( 17.89687500061451431, -2.746126346562642428, -4.756430356249999214 ) ) ;
#24638=CARTESIAN_POINT ( 'NONE',  ( 27.29999999999999716, 0.000000000000000000, 4.999999999999998224 ) ) ;
#24667=CARTESIAN_POINT ( 'NONE',  ( 28.53749999999999787, 5.773502691896255534, 3.535250795749688894E-16 ) ) ;
#24673=CARTESIAN_POINT ( 'NONE',  ( 28.81875000122903074, -5.773502691896255534, -1.060575238724906372E-15 ) ) ;
#24687=CARTESIAN_POINT ( 'NONE',  ( 15.75937500061451502, 2.746126346562643317, 4.756430356249998326 ) ) ;
#24690=CARTESIAN_POINT ( 'NONE',  ( 23.37187500061451573, 4.119189519843966529, 2.378215178124999607 ) ) ;
#24694=CARTESIAN_POINT ( 'NONE',  ( 28.83749999999999858, -2.886751345948149972, -4.999999999999956479 ) ) ;
#24706=CARTESIAN_POINT ( 'NONE',  ( 27.38437500061451857, 5.824947211148865298E-16, -4.756430356249998326 ) ) ;
#24709=EDGE_CURVE ( 'NONE', #52280, #34596, #20582, .T. ) ;
#24726=CARTESIAN_POINT ( 'NONE',  ( 11.25937500061451679, 4.119189519843966529, -2.378215178124998275 ) ) ;
#24738=CARTESIAN_POINT ( 'NONE',  ( 22.12500000000000000, 6.123233995736764310E-16, -4.999999999999998224 ) ) ;
#24752=ORIENTED_EDGE ( 'NONE', *, *, #49936, .T. ) ;
#24755=CARTESIAN_POINT ( 'NONE',  ( 15.08437500061451786, -4.119189519843968306, 2.378215178124996054 ) ) ;
#24762=CARTESIAN_POINT ( 'NONE',  ( 16.61250000000000426, -5.773502691896255534, -1.060575238724906372E-15 ) ) ;
#24766=CARTESIAN_POINT ( 'NONE',  ( 22.28437500061451360, -2.746126346562641984, -4.756430356249999214 ) ) ;
#24774=CARTESIAN_POINT ( 'NONE',  ( 22.58437500061451786, -2.746126346562646425, 4.756430356249996549 ) ) ;
#24776=CARTESIAN_POINT ( 'NONE',  ( 7.846875000614515372, -4.119189519843965641, -2.378215178125001383 ) ) ;
#24785=VERTEX_POINT ( 'NONE', #36426 ) ;
#24787=CARTESIAN_POINT ( 'NONE',  ( 11.07187500061451679, 5.824947211148865298E-16, -4.756430356249998326 ) ) ;
#24807=CARTESIAN_POINT ( 'NONE',  ( 20.52187500061451786, -5.492252693125287522, -1.008910452111647106E-15 ) ) ;
#24809=CARTESIAN_POINT ( 'NONE',  ( 28.59375000122903288, 5.773502691896255534, 3.535250795749688401E-16 ) ) ;
#24814=ORIENTED_EDGE ( 'NONE', *, *, #10750, .T. ) ;
#24834=DIRECTION ( 'NONE',  ( 0.000000000000000000, 0.000000000000000000, 1.000000000000000000 ) ) ;
#24841=CARTESIAN_POINT ( 'NONE',  ( 22.47187500061451715, 2.746126346562645981, -4.756430356249997438 ) ) ;
#24848=CARTESIAN_POINT ( 'NONE',  ( 24.93750000000000355, 5.773502691896255534, 3.535250795749688894E-16 ) ) ;
#24851=LINE ( 'NONE', #36672, #60717 ) ;
#24853=DIRECTION ( 'NONE',  ( -1.000000000000000000, -0.000000000000000000, -0.000000000000000000 ) ) ;
#24858=CARTESIAN_POINT ( 'NONE',  ( 7.668750001229033053, -5.773502691896255534, -1.060575238724906372E-15 ) ) ;
#24860=CARTESIAN_POINT ( 'NONE',  ( 15.68437500061451573, 5.492252693125287522, 3.363034840372157021E-16 ) ) ;
#24872=CARTESIAN_POINT ( 'NONE',  ( 10.80937500061451573, 2.746126346562643317, 4.756430356249998326 ) ) ;
#24873=ORIENTED_EDGE ( 'NONE', *, *, #15601, .T. ) ;
#24880=CARTESIAN_POINT ( 'NONE',  ( -5.000000000000004441, 6.123233995736764310E-16, -4.999999999999998224 ) ) ;
#24884=CARTESIAN_POINT ( 'NONE',  ( 29.63437500061451857, 5.492252693125287522, 3.363034840372157021E-16 ) ) ;
#24887=CARTESIAN_POINT ( 'NONE',  ( 9.299999999999998934, 0.000000000000000000, 4.999999999999998224 ) ) ;
#24895=CARTESIAN_POINT ( 'NONE',  ( 27.12187500061451573, 2.746126346562643317, 4.756430356249998326 ) ) ;
#24897=CARTESIAN_POINT ( 'NONE',  ( 9.721875000614517148, -5.492252693125287522, -1.008910452111647106E-15 ) ) ;
#24904=( BOUNDED_CURVE ( )  B_SPLINE_CURVE ( 2, ( #39361, #21253, #10183, #44906, #11643, #72242, #32718 ),
 .UNSPECIFIED., .F., .F. ) 
 B_SPLINE_CURVE_WITH_KNOTS ( ( 3, 2, 2, 3 ),
 ( 0.8399999999999999689, 0.8433333333333334902, 0.8466666666666667895, 0.8500000000000001998 ),
 .UNSPECIFIED. ) 
 CURVE ( )  GEOMETRIC_REPRESENTATION_ITEM ( )  RATIONAL_B_SPLINE_CURVE ( ( 1.000000000000000000, 0.8660254037844387076, 1.000000000000000000, 0.8660254037844387076, 1.000000000000000000, 0.8660254037844298258, 1.000000000000008882 ) ) 
 REPRESENTATION_ITEM ( '' )  );
#24909=( LENGTH_UNIT ( ) NAMED_UNIT ( * ) SI_UNIT ( .MILLI., .METRE. ) );
#24914=CARTESIAN_POINT ( 'NONE',  ( 22.21875000122903643, 2.886751345948129099, -4.999999999999998224 ) ) ;
#24959=ORIENTED_EDGE ( 'NONE', *, *, #67238, .T. ) ;
#24962=EDGE_CURVE ( 'NONE', #64001, #34347, #30092, .T. ) ;
#24964=CARTESIAN_POINT ( 'NONE',  ( 25.91250000000000142, 2.886751345948098901, 5.000000000000047073 ) ) ;
#24967=CARTESIAN_POINT ( 'NONE',  ( 15.64687500061451608, 4.119189519843966529, -2.378215178124998275 ) ) ;
#24984=CARTESIAN_POINT ( 'NONE',  ( 8.306250001229031454, 4.330127018922192761, -2.499999999999997780 ) ) ;
#24987=CARTESIAN_POINT ( 'NONE',  ( 18.75937500061451857, -4.119189519843965641, -2.378215178125001383 ) ) ;
#25002=CARTESIAN_POINT ( 'NONE',  ( 14.02499999999999858, 6.123233995736764310E-16, -4.999999999999998224 ) ) ;
#25006=CARTESIAN_POINT ( 'NONE',  ( 27.35625000122903216, 0.000000000000000000, 4.999999999999998224 ) ) ;
#25008=CARTESIAN_POINT ( 'NONE',  ( 26.45625000122903003, 0.000000000000000000, 4.999999999999998224 ) ) ;
#25009=FACE_OUTER_BOUND ( 'NONE', #64177, .T. ) ;
#25031=CARTESIAN_POINT ( 'NONE',  ( 29.81250000000000000, 2.886751345948129099, -4.999999999999998224 ) ) ;
#25040=DIRECTION ( 'NONE',  ( -1.000000000000000000, -0.000000000000000000, -0.000000000000000000 ) ) ;
#25048=DIRECTION ( 'NONE',  ( -1.000000000000000000, -0.000000000000000000, -0.000000000000000000 ) ) ;
#25050=CARTESIAN_POINT ( 'NONE',  ( 14.59687500061451537, -4.119189519843965641, -2.378215178125001383 ) ) ;
#25053=CARTESIAN_POINT ( 'NONE',  ( 24.75937500061451502, 2.746126346562643317, 4.756430356249998326 ) ) ;
#25060=LINE ( 'NONE', #65318, #37125 ) ;
#25061=CARTESIAN_POINT ( 'NONE',  ( 25.55625000122903501, 0.000000000000000000, 4.999999999999998224 ) ) ;
#25068=CARTESIAN_POINT ( 'NONE',  ( 23.97187500061451360, 2.746126346562643317, 4.756430356249998326 ) ) ;
#25071=FACE_OUTER_BOUND ( 'NONE', #10177, .T. ) ;
#25077=CARTESIAN_POINT ( 'NONE',  ( 25.33125000122903003, 6.123233995736764310E-16, -4.999999999999998224 ) ) ;
#25087=CARTESIAN_POINT ( 'NONE',  ( 13.43437500061451750, 5.824947211148865298E-16, -4.756430356249998326 ) ) ;
#25116=CARTESIAN_POINT ( 'NONE',  ( 14.33437500061451786, 5.824947211148865298E-16, -4.756430356249998326 ) ) ;
#25119=( BOUNDED_CURVE ( )  B_SPLINE_CURVE ( 2, ( #11912, #29895, #41708, #475, #64232, #68074, #40000 ),
 .UNSPECIFIED., .F., .F. ) 
 B_SPLINE_CURVE_WITH_KNOTS ( ( 3, 2, 2, 3 ),
 ( 0.4900000000000001021, 0.4933333333333334569, 0.4966666666666667562, 0.5000000000000001110 ),
 .UNSPECIFIED. ) 
 CURVE ( )  GEOMETRIC_REPRESENTATION_ITEM ( )  RATIONAL_B_SPLINE_CURVE ( ( 0.9999999999999955591, 0.8660254037844431485, 1.000000000000000000, 0.8660254037844387076, 1.000000000000000000, 0.8660254037844342667, 1.000000000000004441 ) ) 
 REPRESENTATION_ITEM ( '' )  );
#25123=CARTESIAN_POINT ( 'NONE',  ( 14.58750000000000036, 5.773502691896255534, 3.535250795749688894E-16 ) ) ;
#25127=EDGE_CURVE ( 'NONE', #9094, #66820, #24904, .T. ) ;
#25128=CARTESIAN_POINT ( 'NONE',  ( 22.09687500061451360, 0.000000000000000000, 4.756430356249998326 ) ) ;
#25129=CARTESIAN_POINT ( 'NONE',  ( 15.63749999999999929, -2.886751345948074920, 5.000000000000092371 ) ) ;
#25136=CARTESIAN_POINT ( 'NONE',  ( 22.88437500061451502, 5.492252693125287522, 3.363034840372157021E-16 ) ) ;
#25138=CARTESIAN_POINT ( 'NONE',  ( 7.921875000614517326, 5.824947211148865298E-16, -4.756430356249998326 ) ) ;
#25150=CARTESIAN_POINT ( 'NONE',  ( 9.946875000614516793, 0.000000000000000000, 4.756430356249998326 ) ) ;
#25171=CARTESIAN_POINT ( 'NONE',  ( 19.84687500061451360, 5.492252693125287522, 3.363034840372157021E-16 ) ) ;
#25173=CARTESIAN_POINT ( 'NONE',  ( 28.63125000122903074, 4.330127018922191873, 2.499999999999999556 ) ) ;
#25196=CARTESIAN_POINT ( 'NONE',  ( 45.00000000000000000, 0.000000000000000000, 0.000000000000000000 ) ) ;
#25203=CARTESIAN_POINT ( 'NONE',  ( 21.27187500061451786, 2.746126346562643317, 4.756430356249998326 ) ) ;
#25210=CARTESIAN_POINT ( 'NONE',  ( 22.87500000000000000, -4.330127018922194537, 2.499999999999995559 ) ) ;
#25214=DIRECTION ( 'NONE',  ( 0.000000000000000000, -8.673617379884037937E-17, -1.000000000000000000 ) ) ;
#25221=CARTESIAN_POINT ( 'NONE',  ( 28.73437500061451644, 5.492252693125287522, 3.363034840372157021E-16 ) ) ;
#25223=CARTESIAN_POINT ( 'NONE',  ( 15.00937500061451502, -5.492252693125287522, -1.008910452111647106E-15 ) ) ;
#25231=CARTESIAN_POINT ( 'NONE',  ( 24.20625000122903359, 0.000000000000000000, 4.999999999999998224 ) ) ;
#25235=CARTESIAN_POINT ( 'NONE',  ( 7.509375000614516793, 2.746126346562645981, -4.756430356249997438 ) ) ;
#25246=CARTESIAN_POINT ( 'NONE',  ( 29.14687500061451431, 4.119189519843966529, -2.378215178124998275 ) ) ;
#25251=CARTESIAN_POINT ( 'NONE',  ( 7.875000000000000000, 4.330127018922191873, 2.499999999999999556 ) ) ;
#25258=EDGE_CURVE ( 'NONE', #17653, #50451, #33803, .T. ) ;
#25260=CARTESIAN_POINT ( 'NONE',  ( 26.78437500061451360, -4.119189519843968306, 2.378215178124996054 ) ) ;
#25262=CARTESIAN_POINT ( 'NONE',  ( 11.40937500061451892, 0.000000000000000000, 4.756430356249998326 ) ) ;
#25274=FILL_AREA_STYLE_COLOUR ( '', #49755 ) ;
#25281=CARTESIAN_POINT ( 'NONE',  ( 22.14375000122903359, -2.886751345948125991, -5.000000000000000000 ) ) ;
#25283=FACE_OUTER_BOUND ( 'NONE', #35723, .T. ) ;
#25297=CARTESIAN_POINT ( 'NONE',  ( 28.69687500061451502, -2.746126346562642428, -4.756430356249999214 ) ) ;
#25304=AXIS2_PLACEMENT_3D ( 'NONE', #24577, #36031, #51587 ) ;
#25307=CARTESIAN_POINT ( 'NONE',  ( 14.75625000122903252, 0.000000000000000000, 4.999999999999998224 ) ) ;
#25316=CARTESIAN_POINT ( 'NONE',  ( 23.17500000000000071, 4.330127018922191873, 2.499999999999999556 ) ) ;
#25317=CARTESIAN_POINT ( 'NONE',  ( 16.48125000122903216, 4.330127018922191873, 2.499999999999999556 ) ) ;
#25320=AXIS2_PLACEMENT_3D ( 'NONE', #53956, #9249, #31784 ) ;
#25332=( BOUNDED_CURVE ( )  B_SPLINE_CURVE ( 2, ( #22965, #45526, #68056, #17425, #39984, #24056, #22608 ),
 .UNSPECIFIED., .F., .F. ) 
 B_SPLINE_CURVE_WITH_KNOTS ( ( 3, 2, 2, 3 ),
 ( 0.9500000000000000666, 0.9533333333333334769, 0.9566666666666666652, 0.9599999999999999645 ),
 .UNSPECIFIED. ) 
 CURVE ( )  GEOMETRIC_REPRESENTATION_ITEM ( )  RATIONAL_B_SPLINE_CURVE ( ( 0.9999999999999955591, 0.8660254037844431485, 1.000000000000000000, 0.8660254037844387076, 1.000000000000000000, 0.8660254037844387076, 1.000000000000000000 ) ) 
 REPRESENTATION_ITEM ( '' )  );
#25338=CARTESIAN_POINT ( 'NONE',  ( 16.73437500061451644, -2.746126346562646425, 4.756430356249996549 ) ) ;
#25353=CARTESIAN_POINT ( 'NONE',  ( 16.27499999999999858, 6.123233995736764310E-16, -4.999999999999998224 ) ) ;
#25357=CARTESIAN_POINT ( 'NONE',  ( 8.906250001229031099, 0.000000000000000000, 4.999999999999998224 ) ) ;
#25358=CARTESIAN_POINT ( 'NONE',  ( 17.59687500061451715, 5.492252693125287522, 3.363034840372157021E-16 ) ) ;
#25370=VERTEX_POINT ( 'NONE', #1649 ) ;
#25376=CARTESIAN_POINT ( 'NONE',  ( 28.48125000122902861, 6.123233995736764310E-16, -4.999999999999998224 ) ) ;
#25380=CARTESIAN_POINT ( 'NONE',  ( 7.537500000000002309, -2.886751345948130876, 4.999999999999996447 ) ) ;
#25381=CARTESIAN_POINT ( 'NONE',  ( 8.324999999999999289, 4.330127018922191873, 2.499999999999999556 ) ) ;
#25404=CARTESIAN_POINT ( 'NONE',  ( 28.91250000000000497, 2.886751345948129099, -4.999999999999998224 ) ) ;
#25406=CARTESIAN_POINT ( 'NONE',  ( 26.53125000122902932, -4.330127018922194537, 2.499999999999995559 ) ) ;
#25422=CARTESIAN_POINT ( 'NONE',  ( 15.64687500061451608, 4.119189519843966529, -2.378215178124998275 ) ) ;
#25425=CARTESIAN_POINT ( 'NONE',  ( 24.23437500061451644, 5.492252693125287522, 3.363034840372157021E-16 ) ) ;
#25436=CARTESIAN_POINT ( 'NONE',  ( 13.01249999999999929, -5.773502691896255534, -1.060575238724906372E-15 ) ) ;
#25443=CARTESIAN_POINT ( 'NONE',  ( 23.67187500061451999, -5.492252693125287522, -1.008910452111647106E-15 ) ) ;
#25454=ORIENTED_EDGE ( 'NONE', *, *, #46306, .F. ) ;
#25463=CARTESIAN_POINT ( 'NONE',  ( 12.00937500061451857, -4.119189519843965641, -2.378215178125001383 ) ) ;
#25487=ORIENTED_EDGE ( 'NONE', *, *, #26658, .F. ) ;
#25492=CARTESIAN_POINT ( 'NONE',  ( 13.24687500061451750, -2.746126346562646425, 4.756430356249996549 ) ) ;
#25493=CARTESIAN_POINT ( 'NONE',  ( 29.17500000000000071, -4.330127018922194537, 2.499999999999995559 ) ) ;
#25500=CARTESIAN_POINT ( 'NONE',  ( 14.81250000000000000, -5.773502691896255534, -1.060575238724906372E-15 ) ) ;
#25503=LINE ( 'NONE', #48048, #61880 ) ;
#25511=CARTESIAN_POINT ( 'NONE',  ( 22.80937500061451573, 2.746126346562645981, -4.756430356249997438 ) ) ;
#25513=CARTESIAN_POINT ( 'NONE',  ( 9.871875000614517504, 4.119189519843966529, 2.378215178124999607 ) ) ;
#25524=CARTESIAN_POINT ( 'NONE',  ( 10.39687500061451608, 0.000000000000000000, 4.756430356249998326 ) ) ;
#25549=CARTESIAN_POINT ( 'NONE',  ( 20.33437500061451786, 4.119189519843966529, 2.378215178124999607 ) ) ;
#25555=VERTEX_POINT ( 'NONE', #52607 ) ;
#25568=EDGE_CURVE ( 'NONE', #60311, #26800, #40889, .T. ) ;
#25584=CARTESIAN_POINT ( 'NONE',  ( 21.75937500061451502, 0.000000000000000000, 4.756430356249998326 ) ) ;
#25590=CARTESIAN_POINT ( 'NONE',  ( 21.71249999999999858, 2.886751345948129099, -4.999999999999998224 ) ) ;
#25593=CARTESIAN_POINT ( 'NONE',  ( 9.225000000000001421, 4.330127018922191873, 2.499999999999999556 ) ) ;
#25601=CARTESIAN_POINT ( 'NONE',  ( 8.193750001229034297, -2.886751345948125991, -5.000000000000000000 ) ) ;
#25603=CARTESIAN_POINT ( 'NONE',  ( 16.73437500061451644, -2.746126346562646425, 4.756430356249996549 ) ) ;
#25611=VECTOR ( 'NONE', #35367, 1000.000000000000000 ) ;
#25614=CARTESIAN_POINT ( 'NONE',  ( 7.621875000614515727, 4.119189519843966529, 2.378215178124999607 ) ) ;
#25625=CARTESIAN_POINT ( 'NONE',  ( 27.98437500061451644, -2.746126346562646425, 4.756430356249996549 ) ) ;
#25629=CARTESIAN_POINT ( 'NONE',  ( 8.250000000000000000, 4.330127018922192761, -2.499999999999997780 ) ) ;
#25636=CARTESIAN_POINT ( 'NONE',  ( 26.59687500061451360, 5.492252693125287522, 3.363034840372157021E-16 ) ) ;
#25638=CARTESIAN_POINT ( 'NONE',  ( 9.834375000614517859, 5.824947211148865298E-16, -4.756430356249998326 ) ) ;
#25648=DIRECTION ( 'NONE',  ( -1.000000000000000000, -0.000000000000000000, -0.000000000000000000 ) ) ;
#25658=CARTESIAN_POINT ( 'NONE',  ( 20.04375000122902861, 5.773502691896255534, 3.535250795749688894E-16 ) ) ;
#25666=CARTESIAN_POINT ( 'NONE',  ( 23.11875000122902790, 2.886751345948101122, -5.000000000000046185 ) ) ;
#25673=CARTESIAN_POINT ( 'NONE',  ( 27.45937500061451786, 4.119189519843966529, -2.378215178124998275 ) ) ;
#25676=EDGE_CURVE ( 'NONE', #31771, #32794, #26356, .T. ) ;
#25677=AXIS2_PLACEMENT_3D ( 'NONE', #45724, #56786, #56439 ) ;
#25700=DIRECTION ( 'NONE',  ( 0.000000000000000000, 0.000000000000000000, 1.000000000000000000 ) ) ;
#25711=CARTESIAN_POINT ( 'NONE',  ( 16.39687500061451431, -4.119189519843965641, -2.378215178125001383 ) ) ;
#25719=CARTESIAN_POINT ( 'NONE',  ( 8.681250001229031454, 6.123233995736764310E-16, -4.999999999999998224 ) ) ;
#25727=CARTESIAN_POINT ( 'NONE',  ( 45.00000000000000000, 6.123233995736764310E-16, -4.999999999999998224 ) ) ;
#25730=FACE_OUTER_BOUND ( 'NONE', #22702, .T. ) ;
#25731=CARTESIAN_POINT ( 'NONE',  ( 16.99687500061451573, -2.746126346562642428, -4.756430356249999214 ) ) ;
#25734=( BOUNDED_CURVE ( )  B_SPLINE_CURVE ( 2, ( #69664, #51953, #23862, #34587, #6527, #29059, #30860 ),
 .UNSPECIFIED., .F., .F. ) 
 B_SPLINE_CURVE_WITH_KNOTS ( ( 3, 2, 2, 3 ),
 ( 0.5300000000000000266, 0.5333333333333333259, 0.5366666666666667362, 0.5400000000000001465 ),
 .UNSPECIFIED. ) 
 CURVE ( )  GEOMETRIC_REPRESENTATION_ITEM ( )  RATIONAL_B_SPLINE_CURVE ( ( 1.000000000000000000, 0.8660254037844387076, 1.000000000000000000, 0.8660254037844387076, 1.000000000000000000, 0.8660254037844342667, 1.000000000000004441 ) ) 
 REPRESENTATION_ITEM ( '' )  );
#25746=CYLINDRICAL_SURFACE ( 'NONE', #7279, 4.999999999999998224 ) ;
#25750=CARTESIAN_POINT ( 'NONE',  ( 29.23125000122903216, -4.330127018922194537, 2.499999999999995559 ) ) ;
#25752=LINE ( 'NONE', #31661, #19491 ) ;
#25754=CYLINDRICAL_SURFACE ( 'NONE', #24212, 4.999999999999998224 ) ;
#25762=ORIENTED_EDGE ( 'NONE', *, *, #67527, .F. ) ;
#25766=DIRECTION ( 'NONE',  ( 0.000000000000000000, -1.000000000000000000, -0.000000000000000000 ) ) ;
#25775=CARTESIAN_POINT ( 'NONE',  ( 7.434375000614519280, -4.119189519843968306, 2.378215178124996054 ) ) ;
#25794=CARTESIAN_POINT ( 'NONE',  ( 15.68437500061451750, 5.492252693125287522, 3.363034840372157021E-16 ) ) ;
#25795=ORIENTED_EDGE ( 'NONE', *, *, #46306, .T. ) ;
#25798=CARTESIAN_POINT ( 'NONE',  ( 23.67187500061451289, 5.824947211148865298E-16, -4.756430356249998326 ) ) ;
#25807=CYLINDRICAL_SURFACE ( 'NONE', #2968, 4.999999999999998224 ) ;
#25808=CARTESIAN_POINT ( 'NONE',  ( 13.83749999999999858, -2.886751345948129988, 4.999999999999997335 ) ) ;
#25815=CARTESIAN_POINT ( 'NONE',  ( 24.90937500061451715, 0.000000000000000000, 4.756430356249998326 ) ) ;
#25819=CARTESIAN_POINT ( 'NONE',  ( 45.00000000000000000, 0.000000000000000000, 0.000000000000000000 ) ) ;
#25826=CARTESIAN_POINT ( 'NONE',  ( 7.143750001229036251, -2.886751345948130876, 4.999999999999996447 ) ) ;
#25836=CARTESIAN_POINT ( 'NONE',  ( 11.40937500061451892, 0.000000000000000000, 4.756430356249998326 ) ) ;
#25849=ORIENTED_EDGE ( 'NONE', *, *, #15556, .F. ) ;
#25864=CARTESIAN_POINT ( 'NONE',  ( 12.83437500061451786, -4.119189519843968306, 2.378215178124996054 ) ) ;
#25872=CARTESIAN_POINT ( 'NONE',  ( 15.03749999999999964, 5.773502691896255534, 3.535250795749688894E-16 ) ) ;
#25882=DIRECTION ( 'NONE',  ( 0.000000000000000000, 0.000000000000000000, 1.000000000000000000 ) ) ;
#25884=CARTESIAN_POINT ( 'NONE',  ( 21.72187500061451715, -4.119189519843968306, 2.378215178124996054 ) ) ;
#25886=CARTESIAN_POINT ( 'NONE',  ( 7.659375000614513596, 2.746126346562643317, 4.756430356249998326 ) ) ;
#25897=CARTESIAN_POINT ( 'NONE',  ( 8.634375000614515017, -2.746126346562646425, 4.756430356249996549 ) ) ;
#25902=EDGE_CURVE ( 'NONE', #39550, #14695, #48441, .T. ) ;
#25904=CARTESIAN_POINT ( 'NONE',  ( 23.55000000000000071, 4.330127018922192761, -2.499999999999997780 ) ) ;
#25917=CARTESIAN_POINT ( 'NONE',  ( 22.94999999999999929, -4.330127018922190985, -2.500000000000001332 ) ) ;
#25920=CARTESIAN_POINT ( 'NONE',  ( 18.53437500061451715, 4.119189519843966529, 2.378215178124999607 ) ) ;
#25924=ORIENTED_EDGE ( 'NONE', *, *, #23115, .T. ) ;
#25944=SHAPE_REPRESENTATION ( 'spindle', ( #23765 ), #1386 ) ;
#25947=ORIENTED_EDGE ( 'NONE', *, *, #33660, .T. ) ;
#25951=CARTESIAN_POINT ( 'NONE',  ( 22.32187500061451502, -5.492252693125287522, -1.008910452111647106E-15 ) ) ;
#25957=CARTESIAN_POINT ( 'NONE',  ( 21.33749999999999858, 5.773502691896255534, 3.535250795749688894E-16 ) ) ;
#25959=CARTESIAN_POINT ( 'NONE',  ( 9.074999999999999289, 6.123233995736764310E-16, -4.999999999999998224 ) ) ;
#25962=CARTESIAN_POINT ( 'NONE',  ( 12.01875000122903003, 2.886751345948182834, 4.999999999999902300 ) ) ;
#25967=CARTESIAN_POINT ( 'NONE',  ( 7.331250001229031810, 6.123233995736764310E-16, -4.999999999999998224 ) ) ;
#25969=CARTESIAN_POINT ( 'NONE',  ( 15.53437500061451537, -2.746126346562641984, -4.756430356249999214 ) ) ;
#25980=DIRECTION ( 'NONE',  ( -1.000000000000000000, -0.000000000000000000, -0.000000000000000000 ) ) ;
#25981=CARTESIAN_POINT ( 'NONE',  ( 8.184375000614515727, -2.746126346562646425, 4.756430356249996549 ) ) ;
#25992=CARTESIAN_POINT ( 'NONE',  ( 28.77187500061451431, 4.119189519843966529, 2.378215178124999607 ) ) ;
#25993=ORIENTED_EDGE ( 'NONE', *, *, #1055, .T. ) ;
#25996=CARTESIAN_POINT ( 'NONE',  ( 9.037499999999999645, -2.886751345948125991, -5.000000000000000000 ) ) ;
#26003=CARTESIAN_POINT ( 'NONE',  ( 25.99687500061451928, -2.746126346562641984, -4.756430356249999214 ) ) ;
#26005=CARTESIAN_POINT ( 'NONE',  ( 11.03437500061451715, -4.119189519843968306, 2.378215178124996054 ) ) ;
#26022=CARTESIAN_POINT ( 'NONE',  ( 19.96875000122903288, 2.886751345948129099, -4.999999999999998224 ) ) ;
#26038=CARTESIAN_POINT ( 'NONE',  ( 29.55937500061451573, -4.119189519843965641, -2.378215178125001383 ) ) ;
#26046=CARTESIAN_POINT ( 'NONE',  ( 21.99375000122903145, -2.886751345948102898, 5.000000000000044409 ) ) ;
#26060=ORIENTED_EDGE ( 'NONE', *, *, #20794, .T. ) ;
#26061=CARTESIAN_POINT ( 'NONE',  ( 17.00625000122903074, 0.000000000000000000, 4.999999999999998224 ) ) ;
#26075=CARTESIAN_POINT ( 'NONE',  ( 14.33437500061451431, 5.492252693125287522, 3.363034840372157021E-16 ) ) ;
#26090=CARTESIAN_POINT ( 'NONE',  ( 16.31249999999999645, 2.886751345948018077, -5.000000000000190070 ) ) ;
#26094=CARTESIAN_POINT ( 'NONE',  ( 45.00000000000000000, 0.000000000000000000, 4.999999999999998224 ) ) ;
#26095=CARTESIAN_POINT ( 'NONE',  ( 17.63437500061451502, 4.119189519843966529, 2.378215178124999607 ) ) ;
#26112=CARTESIAN_POINT ( 'NONE',  ( 28.29375000122902861, -2.886751345948129988, 4.999999999999997335 ) ) ;
#26114=FACE_OUTER_BOUND ( 'NONE', #9439, .T. ) ;
#26116=FACE_OUTER_BOUND ( 'NONE', #12074, .T. ) ;
#26123=ORIENTED_EDGE ( 'NONE', *, *, #35290, .F. ) ;
#26136=CARTESIAN_POINT ( 'NONE',  ( 28.64999999999999858, 0.000000000000000000, 4.999999999999998224 ) ) ;
#26141=ADVANCED_FACE ( 'NONE', ( #32908 ), #4482, .T. ) ;
#26145=CARTESIAN_POINT ( 'NONE',  ( 9.168750001229033941, 2.886751345948129099, -4.999999999999997335 ) ) ;
#26155=( BOUNDED_CURVE ( )  B_SPLINE_CURVE ( 2, ( #30955, #15055, #26890, #60114, #49416, #59379, #9157 ),
 .UNSPECIFIED., .F., .F. ) 
 B_SPLINE_CURVE_WITH_KNOTS ( ( 3, 2, 2, 3 ),
 ( 0.3300000000000000711, 0.3333333333333333703, 0.3366666666666667251, 0.3400000000000000799 ),
 .UNSPECIFIED. ) 
 CURVE ( )  GEOMETRIC_REPRESENTATION_ITEM ( )  RATIONAL_B_SPLINE_CURVE ( ( 0.9999999999999977796, 0.8660254037844409281, 1.000000000000000000, 0.8660254037844387076, 1.000000000000000000, 0.8660254037844364872, 1.000000000000002220 ) ) 
 REPRESENTATION_ITEM ( '' )  );
#26157=CARTESIAN_POINT ( 'NONE',  ( 11.93437500061451750, -2.746126346562642428, -4.756430356249999214 ) ) ;
#26161=CARTESIAN_POINT ( 'NONE',  ( 24.53437500061451715, -2.746126346562642428, -4.756430356249999214 ) ) ;
#26170=CARTESIAN_POINT ( 'NONE',  ( 12.22499999999999964, 6.123233995736764310E-16, -4.999999999999998224 ) ) ;
#26177=CARTESIAN_POINT ( 'NONE',  ( 25.28437500061451715, 4.119189519843966529, 2.378215178124999607 ) ) ;
#26181=CARTESIAN_POINT ( 'NONE',  ( 45.00000000000000000, 0.000000000000000000, 0.000000000000000000 ) ) ;
#26187=CARTESIAN_POINT ( 'NONE',  ( 7.181250001229034119, -4.330127018922194537, 2.499999999999995559 ) ) ;
#26195=EDGE_CURVE ( 'NONE', #6463, #4282, #50826, .T. ) ;
#26199=CARTESIAN_POINT ( 'NONE',  ( 10.84687500061451715, 5.492252693125287522, 3.363034840372157021E-16 ) ) ;
#26216=CARTESIAN_POINT ( 'NONE',  ( 16.19999999999999929, -4.330127018922190985, -2.500000000000001332 ) ) ;
#26224=( BOUNDED_CURVE ( )  B_SPLINE_CURVE ( 2, ( #38226, #16780, #72222, #50779, #182, #10887, #39338 ),
 .UNSPECIFIED., .F., .F. ) 
 B_SPLINE_CURVE_WITH_KNOTS ( ( 3, 2, 2, 3 ),
 ( 0.7399999999999999911, 0.7433333333333332904, 0.7466666666666667007, 0.7500000000000000000 ),
 .UNSPECIFIED. ) 
 CURVE ( )  GEOMETRIC_REPRESENTATION_ITEM ( )  RATIONAL_B_SPLINE_CURVE ( ( 1.000000000000000000, 0.8660254037844387076, 1.000000000000000000, 0.8660254037844387076, 1.000000000000000000, 0.8660254037844387076, 1.000000000000000000 ) ) 
 REPRESENTATION_ITEM ( '' )  );
#26225=ORIENTED_EDGE ( 'NONE', *, *, #63349, .F. ) ;
#26229=CARTESIAN_POINT ( 'NONE',  ( 12.87187500061451750, -5.492252693125287522, -1.008910452111647106E-15 ) ) ;
#26238=CARTESIAN_POINT ( 'NONE',  ( 15.75000000000000000, -4.330127018922190985, -2.500000000000001332 ) ) ;
#26246=CARTESIAN_POINT ( 'NONE',  ( 20.15625000122903288, 0.000000000000000000, 4.999999999999998224 ) ) ;
#26250=CARTESIAN_POINT ( 'NONE',  ( 23.03437500061451360, -2.746126346562646425, 4.756430356249996549 ) ) ;
#26263=CARTESIAN_POINT ( 'NONE',  ( 10.20937500061451608, 2.746126346562645981, -4.756430356249997438 ) ) ;
#26285=CARTESIAN_POINT ( 'NONE',  ( 17.52187500061451431, 2.746126346562645981, -4.756430356249997438 ) ) ;
#26317=CARTESIAN_POINT ( 'NONE',  ( 22.35937500061451644, -4.119189519843965641, -2.378215178125001383 ) ) ;
#26320=EDGE_CURVE ( 'NONE', #51781, #56470, #27733, .T. ) ;
#26322=ADVANCED_FACE ( 'NONE', ( #57871 ), #16990, .T. ) ;
#26325=CARTESIAN_POINT ( 'NONE',  ( 22.31250000000000000, 2.886751345948126879, 4.999999999999999112 ) ) ;
#26328=CARTESIAN_POINT ( 'NONE',  ( 20.38125000122903430, 6.123233995736764310E-16, -4.999999999999998224 ) ) ;
#26335=CARTESIAN_POINT ( 'NONE',  ( 7.556250001229035007, 0.000000000000000000, 4.999999999999998224 ) ) ;
#26337=CARTESIAN_POINT ( 'NONE',  ( 15.60937500061451644, 2.746126346562645981, -4.756430356249997438 ) ) ;
#26340=VERTEX_POINT ( 'NONE', #47170 ) ;
#26347=CARTESIAN_POINT ( 'NONE',  ( 8.296875000614518214, -4.119189519843965641, -2.378215178125001383 ) ) ;
#26348=ORIENTED_EDGE ( 'NONE', *, *, #66600, .T. ) ;
#26356=LINE ( 'NONE', #15261, #41837 ) ;
#26369=CARTESIAN_POINT ( 'NONE',  ( 27.53437500061451360, 4.119189519843966529, 2.378215178124999607 ) ) ;
#26371=CARTESIAN_POINT ( 'NONE',  ( 45.00000000000000000, 0.000000000000000000, 0.000000000000000000 ) ) ;
#26389=CARTESIAN_POINT ( 'NONE',  ( 19.51875000122903359, 2.886751345948129099, -4.999999999999998224 ) ) ;
#26392=ORIENTED_EDGE ( 'NONE', *, *, #59010, .T. ) ;
#26404=CARTESIAN_POINT ( 'NONE',  ( 28.17187500061451644, -5.492252693125287522, -1.008910452111647106E-15 ) ) ;
#26414=( BOUNDED_CURVE ( )  B_SPLINE_CURVE ( 2, ( #50104, #34181, #38655, #62270, #10574, #10933, #50825 ),
 .UNSPECIFIED., .F., .F. ) 
 B_SPLINE_CURVE_WITH_KNOTS ( ( 3, 2, 2, 3 ),
 ( 0.9699999999999999734, 0.9733333333333333837, 0.9766666666666666829, 0.9799999999999999822 ),
 .UNSPECIFIED. ) 
 CURVE ( )  GEOMETRIC_REPRESENTATION_ITEM ( )  RATIONAL_B_SPLINE_CURVE ( ( 1.000000000000000000, 0.8660254037844387076, 1.000000000000000000, 0.8660254037844387076, 1.000000000000000000, 0.8660254037844387076, 1.000000000000000000 ) ) 
 REPRESENTATION_ITEM ( '' )  );
#26418=LINE ( 'NONE', #2421, #19687 ) ;
#26425=AXIS2_PLACEMENT_3D ( 'NONE', #67141, #16499, #10969 ) ;
#26428=ORIENTED_EDGE ( 'NONE', *, *, #57573, .T. ) ;
#26436=EDGE_LOOP ( 'NONE', ( #35002, #41040, #69143, #10915 ) ) ;
#26439=( BOUNDED_CURVE ( )  B_SPLINE_CURVE ( 2, ( #9811, #61874, #11281, #5735, #48981, #71510, #32343 ),
 .UNSPECIFIED., .F., .F. ) 
 B_SPLINE_CURVE_WITH_KNOTS ( ( 3, 2, 2, 3 ),
 ( 0.4799999999999999267, 0.4833333333333333370, 0.4866666666666667473, 0.4900000000000001021 ),
 .UNSPECIFIED. ) 
 CURVE ( )  GEOMETRIC_REPRESENTATION_ITEM ( )  RATIONAL_B_SPLINE_CURVE ( ( 1.000000000000002220, 0.8660254037844364872, 1.000000000000000000, 0.8660254037844387076, 1.000000000000000000, 0.8660254037844342667, 1.000000000000004441 ) ) 
 REPRESENTATION_ITEM ( '' )  );
#26444=CARTESIAN_POINT ( 'NONE',  ( 14.85937500061451999, 2.746126346562643317, 4.756430356249998326 ) ) ;
#26455=CARTESIAN_POINT ( 'NONE',  ( 16.81875000122903074, 2.886751345948073588, -5.000000000000094147 ) ) ;
#26463=CARTESIAN_POINT ( 'NONE',  ( 15.23437500061451644, 5.824947211148865298E-16, -4.756430356249998326 ) ) ;
#26480=CARTESIAN_POINT ( 'NONE',  ( 28.21875000122903288, 2.886751345948126879, 4.999999999999999112 ) ) ;
#26491=VERTEX_POINT ( 'NONE', #11466 ) ;
#26508=CARTESIAN_POINT ( 'NONE',  ( 26.28749999999999432, 5.773502691896255534, 3.535250795749688894E-16 ) ) ;
#26510=FACE_OUTER_BOUND ( 'NONE', #34959, .T. ) ;
#26514=CARTESIAN_POINT ( 'NONE',  ( 12.48750000000000249, -2.886751345948074920, 5.000000000000092371 ) ) ;
#26527=VERTEX_POINT ( 'NONE', #53068 ) ;
#26530=CARTESIAN_POINT ( 'NONE',  ( 21.60937500061451644, 2.746126346562643317, 4.756430356249998326 ) ) ;
#26535=CARTESIAN_POINT ( 'NONE',  ( 15.95625000122903181, 4.330127018922192761, -2.499999999999997780 ) ) ;
#26540=CARTESIAN_POINT ( 'NONE',  ( 13.91249999999999964, -5.773502691896255534, -1.060575238724906372E-15 ) ) ;
#26548=CARTESIAN_POINT ( 'NONE',  ( 25.50937500061451502, -4.119189519843965641, -2.378215178125001383 ) ) ;
#26558=CARTESIAN_POINT ( 'NONE',  ( 0.000000000000000000, -4.999999999999999112, 0.000000000000000000 ) ) ;
#26559=VERTEX_POINT ( 'NONE', #2463 ) ;
#26569=CARTESIAN_POINT ( 'NONE',  ( 10.58437500061451964, -4.119189519843968306, 2.378215178124996054 ) ) ;
#26596=CARTESIAN_POINT ( 'NONE',  ( 12.45937500061451786, -4.119189519843965641, -2.378215178125001383 ) ) ;
#26607=CARTESIAN_POINT ( 'NONE',  ( 16.87500000000000000, 4.330127018922191873, 2.499999999999999556 ) ) ;
#26619=CARTESIAN_POINT ( 'NONE',  ( 19.39687500061451786, 0.000000000000000000, 4.756430356249998326 ) ) ;
#26622=CARTESIAN_POINT ( 'NONE',  ( 14.19375000122903074, 5.773502691896255534, 3.535250795749688894E-16 ) ) ;
#26635=ADVANCED_FACE ( 'NONE', ( #25730 ), #54901, .T. ) ;
#26637=CARTESIAN_POINT ( 'NONE',  ( 8.934375000614515727, 5.492252693125287522, 3.363034840372157021E-16 ) ) ;
#26647=ORIENTED_EDGE ( 'NONE', *, *, #43096, .F. ) ;
#26658=EDGE_CURVE ( 'NONE', #54979, #8125, #9104, .T. ) ;
#26660=CARTESIAN_POINT ( 'NONE',  ( 16.77187500061451786, 2.746126346562643317, 4.756430356249998326 ) ) ;
#26692=CARTESIAN_POINT ( 'NONE',  ( 20.44687500061451857, -2.746126346562646425, 4.756430356249996549 ) ) ;
#26698=CARTESIAN_POINT ( 'NONE',  ( 23.02499999999999858, 6.123233995736764310E-16, -4.999999999999998224 ) ) ;
#26701=CARTESIAN_POINT ( 'NONE',  ( 21.48750000000000071, -2.886751345948130876, 4.999999999999996447 ) ) ;
#26702=FACE_OUTER_BOUND ( 'NONE', #20520, .T. ) ;
#26708=CARTESIAN_POINT ( 'NONE',  ( 26.70937500061451431, -5.492252693125287522, -1.008910452111647106E-15 ) ) ;
#26710=CARTESIAN_POINT ( 'NONE',  ( 14.07187500061451679, -4.119189519843968306, 2.378215178124996054 ) ) ;
#26721=CARTESIAN_POINT ( 'NONE',  ( 8.671875000614518214, -4.119189519843968306, 2.378215178124996054 ) ) ;
#26722=ORIENTED_EDGE ( 'NONE', *, *, #24962, .T. ) ;
#26744=CARTESIAN_POINT ( 'NONE',  ( 23.25937500061451857, -4.119189519843965641, -2.378215178125001383 ) ) ;
#26746=CARTESIAN_POINT ( 'NONE',  ( 7.809375000614519280, 0.000000000000000000, 4.756430356249998326 ) ) ;
#26754=EDGE_CURVE ( 'NONE', #8302, #56819, #60731, .T. ) ;
#26764=CARTESIAN_POINT ( 'NONE',  ( 19.63125000122903430, 4.330127018922191873, 2.499999999999999556 ) ) ;
#26779=CARTESIAN_POINT ( 'NONE',  ( 28.32187500061451502, 2.746126346562645981, -4.756430356249997438 ) ) ;
#26786=CARTESIAN_POINT ( 'NONE',  ( 24.93750000000000000, 5.773502691896255534, 3.535250795749688401E-16 ) ) ;
#26797=CARTESIAN_POINT ( 'NONE',  ( 20.67187500061451289, 4.119189519843966529, 2.378215178124999607 ) ) ;
#26800=VERTEX_POINT ( 'NONE', #25357 ) ;
#26812=EDGE_LOOP ( 'NONE', ( #47655, #12826, #5214, #65209 ) ) ;
#26816=CARTESIAN_POINT ( 'NONE',  ( 13.73437500061451644, -2.746126346562642428, -4.756430356249999214 ) ) ;
#26834=CARTESIAN_POINT ( 'NONE',  ( 26.98125000122903216, -4.330127018922194537, 2.499999999999995559 ) ) ;
#26835=CARTESIAN_POINT ( 'NONE',  ( 15.72187500061451892, 2.746126346562645981, -4.756430356249997438 ) ) ;
#26849=CARTESIAN_POINT ( 'NONE',  ( 24.58125000122903003, 4.330127018922191873, 2.499999999999999556 ) ) ;
#26853=CARTESIAN_POINT ( 'NONE',  ( 25.14375000122903003, -2.886751345948129988, 4.999999999999997335 ) ) ;
#26855=CARTESIAN_POINT ( 'NONE',  ( 26.79375000122903216, 5.773502691896255534, 3.535250795749688401E-16 ) ) ;
#26857=VECTOR ( 'NONE', #10161, 1000.000000000000000 ) ;
#26858=CARTESIAN_POINT ( 'NONE',  ( 8.287499999999999645, 5.773502691896255534, 3.535250795749688401E-16 ) ) ;
#26864=ORIENTED_EDGE ( 'NONE', *, *, #48137, .T. ) ;
#26866=CARTESIAN_POINT ( 'NONE',  ( 23.75625000122903074, 0.000000000000000000, 4.999999999999998224 ) ) ;
#26876=( BOUNDED_CURVE ( )  B_SPLINE_CURVE ( 2, ( #12838, #35372, #46106, #58254, #57895, #7303, #29834 ),
 .UNSPECIFIED., .F., .F. ) 
 B_SPLINE_CURVE_WITH_KNOTS ( ( 3, 2, 2, 3 ),
 ( 0.2999999999999999889, 0.3033333333333333437, 0.3066666666666666430, 0.3099999999999999978 ),
 .UNSPECIFIED. ) 
 CURVE ( )  GEOMETRIC_REPRESENTATION_ITEM ( )  RATIONAL_B_SPLINE_CURVE ( ( 1.000000000000000000, 0.8660254037844387076, 1.000000000000000000, 0.8660254037844387076, 1.000000000000000000, 0.8660254037844387076, 1.000000000000000000 ) ) 
 REPRESENTATION_ITEM ( '' )  );
#26886=( BOUNDED_CURVE ( )  B_SPLINE_CURVE ( 2, ( #36254, #7451, #13712, #52519, #25904, #63956, #18519 ),
 .UNSPECIFIED., .F., .F. ) 
 B_SPLINE_CURVE_WITH_KNOTS ( ( 3, 2, 2, 3 ),
 ( 0.2800000000000000266, 0.2833333333333333259, 0.2866666666666667362, 0.2900000000000000355 ),
 .UNSPECIFIED. ) 
 CURVE ( )  GEOMETRIC_REPRESENTATION_ITEM ( )  RATIONAL_B_SPLINE_CURVE ( ( 1.000000000000000000, 0.8660254037844387076, 1.000000000000000000, 0.8660254037844387076, 1.000000000000000000, 0.8660254037844364872, 1.000000000000002220 ) ) 
 REPRESENTATION_ITEM ( '' )  );
#26890=CARTESIAN_POINT ( 'NONE',  ( 22.50000000000000000, -4.330127018922190985, -2.500000000000001332 ) ) ;
#26905=CARTESIAN_POINT ( 'NONE',  ( 22.54687500061451644, 0.000000000000000000, 4.756430356249998326 ) ) ;
#26912=EDGE_CURVE ( 'NONE', #4778, #71509, #38266, .T. ) ;
#26915=CARTESIAN_POINT ( 'NONE',  ( 13.72500000000000142, 4.330127018922191873, 2.499999999999999556 ) ) ;
#26922=CARTESIAN_POINT ( 'NONE',  ( 21.27187500061451786, 2.746126346562643317, 4.756430356249998326 ) ) ;
#26925=CARTESIAN_POINT ( 'NONE',  ( 13.29375000122903394, 5.773502691896255534, 3.535250795749688401E-16 ) ) ;
#26932=LINE ( 'NONE', #60519, #15929 ) ;
#26944=CARTESIAN_POINT ( 'NONE',  ( 9.721875000614517148, -5.492252693125287522, -1.008910452111647106E-15 ) ) ;
#26966=CARTESIAN_POINT ( 'NONE',  ( 10.77187500061451786, 2.746126346562645981, -4.756430356249997438 ) ) ;
#26976=CARTESIAN_POINT ( 'NONE',  ( 25.72499999999999787, 6.123233995736764310E-16, -4.999999999999998224 ) ) ;
#26979=EDGE_CURVE ( 'NONE', #29126, #27766, #70650, .T. ) ;
#26988=CARTESIAN_POINT ( 'NONE',  ( 20.82187500061451502, -4.119189519843968306, 2.378215178124996054 ) ) ;
#26991=CARTESIAN_POINT ( 'NONE',  ( 13.85625000122903216, 0.000000000000000000, 4.999999999999998224 ) ) ;
#27004=CARTESIAN_POINT ( 'NONE',  ( 28.58437500061451786, -4.119189519843968306, 2.378215178124996054 ) ) ;
#27013=VERTEX_POINT ( 'NONE', #22368 ) ;
#27022=LINE ( 'NONE', #22194, #62701 ) ;
#27026=CARTESIAN_POINT ( 'NONE',  ( 17.93437500061451928, 5.824947211148865298E-16, -4.756430356249998326 ) ) ;
#27057=CARTESIAN_POINT ( 'NONE',  ( 19.77187500061451786, 2.746126346562645981, -4.756430356249997438 ) ) ;
#27063=CARTESIAN_POINT ( 'NONE',  ( 19.87500000000000000, 6.123233995736764310E-16, -4.999999999999998224 ) ) ;
#27065=CARTESIAN_POINT ( 'NONE',  ( 20.69999999999999929, -4.330127018922190985, -2.500000000000001332 ) ) ;
#27068=DIRECTION ( 'NONE',  ( -1.000000000000000000, -0.000000000000000000, -0.000000000000000000 ) ) ;
#27073=CARTESIAN_POINT ( 'NONE',  ( 27.23437500061450933, -2.746126346562642428, -4.756430356249999214 ) ) ;
#27075=CARTESIAN_POINT ( 'NONE',  ( 12.79687500061451466, -4.119189519843965641, -2.378215178125001383 ) ) ;
#27084=CARTESIAN_POINT ( 'NONE',  ( 16.78125000122903288, 6.123233995736764310E-16, -4.999999999999998224 ) ) ;
#27093=CYLINDRICAL_SURFACE ( 'NONE', #48956, 4.999999999999998224 ) ;
#27099=ORIENTED_EDGE ( 'NONE', *, *, #57008, .T. ) ;
#27101=CARTESIAN_POINT ( 'NONE',  ( 29.36250000000000782, 2.886751345948158409, -4.999999999999947597 ) ) ;
#27108=CARTESIAN_POINT ( 'NONE',  ( 24.38437500061451502, 4.119189519843966529, 2.378215178124999607 ) ) ;
#27110=CARTESIAN_POINT ( 'NONE',  ( 8.859375000614518214, -4.119189519843965641, -2.378215178125001383 ) ) ;
#27127=CARTESIAN_POINT ( 'NONE',  ( 19.03125000122902932, 6.123233995736764310E-16, -4.999999999999998224 ) ) ;
#27130=ORIENTED_EDGE ( 'NONE', *, *, #65502, .T. ) ;
#27131=EDGE_CURVE ( 'NONE', #1724, #45117, #60282, .T. ) ;
#27144=CARTESIAN_POINT ( 'NONE',  ( 25.65937500061451715, 4.119189519843966529, -2.378215178124998275 ) ) ;
#27156=EDGE_CURVE ( 'NONE', #64487, #46244, #15410, .T. ) ;
#27157=CARTESIAN_POINT ( 'NONE',  ( 27.71250000000000213, 2.886751345948098901, 5.000000000000047073 ) ) ;
#27159=CARTESIAN_POINT ( 'NONE',  ( 10.85625000122903216, -4.330127018922190985, -2.500000000000001332 ) ) ;
#27163=CARTESIAN_POINT ( 'NONE',  ( 21.68437500061451573, -2.746126346562646425, 4.756430356249996549 ) ) ;
#27167=CARTESIAN_POINT ( 'NONE',  ( 10.55625000122903323, 4.330127018922192761, -2.499999999999997780 ) ) ;
#27169=DIRECTION ( 'NONE',  ( -1.000000000000000000, -0.000000000000000000, -0.000000000000000000 ) ) ;
#27177=ORIENTED_EDGE ( 'NONE', *, *, #51676, .T. ) ;
#27181=CARTESIAN_POINT ( 'NONE',  ( 14.82187500061451502, 4.119189519843966529, 2.378215178124999607 ) ) ;
#27187=ORIENTED_EDGE ( 'NONE', *, *, #5393, .T. ) ;
#27197=CARTESIAN_POINT ( 'NONE',  ( 29.07187500061451502, 5.824947211148865298E-16, -4.756430356249998326 ) ) ;
#27198=CARTESIAN_POINT ( 'NONE',  ( 14.85937500061451644, 4.119189519843966529, -2.378215178124998275 ) ) ;
#27211=CARTESIAN_POINT ( 'NONE',  ( 25.61250000000000071, -5.773502691896255534, -1.060575238724906372E-15 ) ) ;
#27215=CARTESIAN_POINT ( 'NONE',  ( 26.75625000122903430, 4.330127018922192761, -2.499999999999997780 ) ) ;
#27225=ORIENTED_EDGE ( 'NONE', *, *, #17040, .F. ) ;
#27227=CARTESIAN_POINT ( 'NONE',  ( 23.79375000122903216, -2.886751345948102898, 5.000000000000044409 ) ) ;
#27230=PLANE ( 'NONE',  #59836 ) ;
#27247=CARTESIAN_POINT ( 'NONE',  ( 12.44999999999999929, 0.000000000000000000, 4.999999999999998224 ) ) ;
#27266=CARTESIAN_POINT ( 'NONE',  ( 22.39687500061451431, 4.119189519843966529, -2.378215178124998275 ) ) ;
#27269=CARTESIAN_POINT ( 'NONE',  ( 45.00000000000000000, 6.123233995736764310E-16, -4.999999999999998224 ) ) ;
#27273=CARTESIAN_POINT ( 'NONE',  ( 26.62500000000000000, 6.123233995736764310E-16, -4.999999999999998224 ) ) ;
#27274=ORIENTED_EDGE ( 'NONE', *, *, #20762, .T. ) ;
#27275=CARTESIAN_POINT ( 'NONE',  ( 10.57500000000000107, 4.330127018922191873, 2.499999999999999556 ) ) ;
#27282=CARTESIAN_POINT ( 'NONE',  ( 21.68437500061451573, 4.119189519843966529, 2.378215178124999607 ) ) ;
#27303=CARTESIAN_POINT ( 'NONE',  ( 10.92187500061451644, 2.746126346562643317, 4.756430356249998326 ) ) ;
#27315=CYLINDRICAL_SURFACE ( 'NONE', #60937, 4.999999999999998224 ) ;
#27326=CARTESIAN_POINT ( 'NONE',  ( 10.54687500061451644, -2.746126346562646425, 4.756430356249996549 ) ) ;
#27338=CYLINDRICAL_SURFACE ( 'NONE', #70155, 4.999999999999998224 ) ;
#27347=CARTESIAN_POINT ( 'NONE',  ( 19.05937500061451217, -5.492252693125287522, -1.008910452111647106E-15 ) ) ;
#27350=CARTESIAN_POINT ( 'NONE',  ( 13.14375000122903536, -2.886751345948125991, -5.000000000000000000 ) ) ;
#27365=CARTESIAN_POINT ( 'NONE',  ( 7.996875000614515727, 4.119189519843966529, -2.378215178124998275 ) ) ;
#27386=CARTESIAN_POINT ( 'NONE',  ( 16.84687500061452070, -2.746126346562646425, 4.756430356249996549 ) ) ;
#27419=CARTESIAN_POINT ( 'NONE',  ( 17.70937500061451431, 0.000000000000000000, 4.756430356249998326 ) ) ;
#27421=EDGE_CURVE ( 'NONE', #52965, #24228, #38073, .T. ) ;
#27426=CARTESIAN_POINT ( 'NONE',  ( 19.91250000000000142, 2.886751345948129099, -4.999999999999998224 ) ) ;
#27428=CARTESIAN_POINT ( 'NONE',  ( 26.44687500061451502, 4.119189519843966529, -2.378215178124998275 ) ) ;
#27431=EDGE_CURVE ( 'NONE', #675, #26527, #50404, .T. ) ;
#27438=CARTESIAN_POINT ( 'NONE',  ( 27.75937500061451502, 2.746126346562645981, -4.756430356249997438 ) ) ;
#27440=CARTESIAN_POINT ( 'NONE',  ( 14.48437500061451644, -2.746126346562646425, 4.756430356249996549 ) ) ;
#27446=CARTESIAN_POINT ( 'NONE',  ( 26.17500000000000071, 6.123233995736764310E-16, -4.999999999999998224 ) ) ;
#27456=ORIENTED_EDGE ( 'NONE', *, *, #14038, .T. ) ;
#27473=CARTESIAN_POINT ( 'NONE',  ( 24.30937500061451573, 4.119189519843966529, -2.378215178124998275 ) ) ;
#27475=CARTESIAN_POINT ( 'NONE',  ( 8.934375000614517504, 5.824947211148865298E-16, -4.756430356249998326 ) ) ;
#27491=CARTESIAN_POINT ( 'NONE',  ( 18.88125000122903430, -4.330127018922194537, 2.499999999999995559 ) ) ;
#27493=DIRECTION ( 'NONE',  ( 0.4999999999999975575, 0.000000000000000000, -0.8660254037844400399 ) ) ;
#27507=CARTESIAN_POINT ( 'NONE',  ( 26.07187500061451857, 2.746126346562645981, -4.756430356249997438 ) ) ;
#27518=( BOUNDED_CURVE ( )  B_SPLINE_CURVE ( 2, ( #52870, #40338, #7082, #6722, #40706, #29611, #24060 ),
 .UNSPECIFIED., .F., .F. ) 
 B_SPLINE_CURVE_WITH_KNOTS ( ( 3, 2, 2, 3 ),
 ( 0.6199999999999999956, 0.6233333333333332948, 0.6266666666666668162, 0.6300000000000001155 ),
 .UNSPECIFIED. ) 
 CURVE ( )  GEOMETRIC_REPRESENTATION_ITEM ( )  RATIONAL_B_SPLINE_CURVE ( ( 1.000000000000000000, 0.8660254037844387076, 1.000000000000000000, 0.8660254037844387076, 1.000000000000000000, 0.8660254037844342667, 1.000000000000004441 ) ) 
 REPRESENTATION_ITEM ( '' )  );
#27520=CARTESIAN_POINT ( 'NONE',  ( 12.50625000122903430, 0.000000000000000000, 4.999999999999998224 ) ) ;
#27524=CARTESIAN_POINT ( 'NONE',  ( 21.00937500061451857, 2.746126346562645981, -4.756430356249997438 ) ) ;
#27537=CARTESIAN_POINT ( 'NONE',  ( 13.32187500061451502, 5.824947211148865298E-16, -4.756430356249998326 ) ) ;
#27546=CARTESIAN_POINT ( 'NONE',  ( 14.67187500061451644, 5.824947211148865298E-16, -4.756430356249998326 ) ) ;
#27564=CARTESIAN_POINT ( 'NONE',  ( 16.13437500061451502, 5.824947211148865298E-16, -4.756430356249998326 ) ) ;
#27570=CARTESIAN_POINT ( 'NONE',  ( 10.46250000000000036, 2.886751345948129099, -4.999999999999997335 ) ) ;
#27574=DIRECTION ( 'NONE',  ( -1.000000000000000000, -0.000000000000000000, -0.000000000000000000 ) ) ;
#27582=CARTESIAN_POINT ( 'NONE',  ( 25.66875000122903216, -5.773502691896255534, -1.060575238724906372E-15 ) ) ;
#27595=CARTESIAN_POINT ( 'NONE',  ( 45.00000000000000000, 0.000000000000000000, 0.000000000000000000 ) ) ;
#27616=CARTESIAN_POINT ( 'NONE',  ( 45.00000000000000000, 0.000000000000000000, 4.999999999999998224 ) ) ;
#27629=CARTESIAN_POINT ( 'NONE',  ( 22.47187500061451360, 4.119189519843966529, 2.378215178124999607 ) ) ;
#27637=CARTESIAN_POINT ( 'NONE',  ( 11.81250000000000000, 2.886751345948129099, -4.999999999999998224 ) ) ;
#27644=CARTESIAN_POINT ( 'NONE',  ( 22.05937500061451573, 4.119189519843966529, -2.378215178124998275 ) ) ;
#27647=CARTESIAN_POINT ( 'NONE',  ( 28.25625000122903074, 0.000000000000000000, 4.999999999999998224 ) ) ;
#27659=CARTESIAN_POINT ( 'NONE',  ( 27.28125000122902932, 4.330127018922191873, 2.499999999999999556 ) ) ;
#27666=CARTESIAN_POINT ( 'NONE',  ( 9.009375000614518569, 4.119189519843966529, -2.378215178124998275 ) ) ;
#27670=EDGE_CURVE ( 'NONE', #38854, #58120, #22536, .T. ) ;
#27689=CARTESIAN_POINT ( 'NONE',  ( 11.78437500061451892, 4.119189519843966529, 2.378215178124999607 ) ) ;
#27709=VECTOR ( 'NONE', #21271, 1000.000000000000000 ) ;
#27710=CARTESIAN_POINT ( 'NONE',  ( 20.40937500061451360, -5.492252693125287522, -1.008910452111647106E-15 ) ) ;
#27713=CARTESIAN_POINT ( 'NONE',  ( 13.21875000122903288, 2.886751345948129099, -4.999999999999998224 ) ) ;
#27729=CARTESIAN_POINT ( 'NONE',  ( 29.44687500061451857, -2.746126346562646425, 4.756430356249996549 ) ) ;
#27733=( BOUNDED_CURVE ( )  B_SPLINE_CURVE ( 2, ( #386, #22541, #67624, #40913, #63426, #28453, #12813 ),
 .UNSPECIFIED., .F., .F. ) 
 B_SPLINE_CURVE_WITH_KNOTS ( ( 3, 2, 2, 3 ),
 ( 0.8100000000000000533, 0.8133333333333333526, 0.8166666666666667629, 0.8200000000000000622 ),
 .UNSPECIFIED. ) 
 CURVE ( )  GEOMETRIC_REPRESENTATION_ITEM ( )  RATIONAL_B_SPLINE_CURVE ( ( 1.000000000000000000, 0.8660254037844387076, 1.000000000000000000, 0.8660254037844387076, 1.000000000000000000, 0.8660254037844342667, 1.000000000000004441 ) ) 
 REPRESENTATION_ITEM ( '' )  );
#27737=CARTESIAN_POINT ( 'NONE',  ( 14.92500000000000071, 6.123233995736764310E-16, -4.999999999999998224 ) ) ;
#27751=CARTESIAN_POINT ( 'NONE',  ( 16.28437500061452070, 4.119189519843966529, 2.378215178124999607 ) ) ;
#27755=EDGE_LOOP ( 'NONE', ( #7214, #66012, #21831, #4946 ) ) ;
#27766=VERTEX_POINT ( 'NONE', #42796 ) ;
#27786=CARTESIAN_POINT ( 'NONE',  ( 19.32187500061451857, 2.746126346562645981, -4.756430356249997438 ) ) ;
#27787=CARTESIAN_POINT ( 'NONE',  ( 14.56875000122903252, 2.886751345948129099, -4.999999999999997335 ) ) ;
#27791=CARTESIAN_POINT ( 'NONE',  ( 19.31250000000000000, -5.773502691896255534, -1.060575238724906372E-15 ) ) ;
#27795=CARTESIAN_POINT ( 'NONE',  ( 26.33437500061451431, -2.746126346562641984, -4.756430356249999214 ) ) ;
#27796=CARTESIAN_POINT ( 'NONE',  ( 14.30625000122903145, 0.000000000000000000, 4.999999999999998224 ) ) ;
#27801=EDGE_CURVE ( 'NONE', #5961, #40656, #25060, .T. ) ;
#27803=CARTESIAN_POINT ( 'NONE',  ( 27.49687500061451573, 0.000000000000000000, 4.756430356249998326 ) ) ;
#27805=CARTESIAN_POINT ( 'NONE',  ( 12.53437500061451537, 5.492252693125287522, 3.363034840372157021E-16 ) ) ;
#27806=ADVANCED_FACE ( 'NONE', ( #59773 ), #25807, .T. ) ;
#27816=CARTESIAN_POINT ( 'NONE',  ( 18.01875000122903003, -5.773502691896255534, -1.060575238724906372E-15 ) ) ;
#27831=CARTESIAN_POINT ( 'NONE',  ( 16.18125000122903145, -4.330127018922194537, 2.499999999999995559 ) ) ;
#27832=VERTEX_POINT ( 'NONE', #59038 ) ;
#27835=VECTOR ( 'NONE', #7440, 1000.000000000000000 ) ;
#27843=CARTESIAN_POINT ( 'NONE',  ( 25.39687500061451431, -2.746126346562646425, 4.756430356249996549 ) ) ;
#27845=CARTESIAN_POINT ( 'NONE',  ( 8.671875000614518214, 2.746126346562643317, 4.756430356249998326 ) ) ;
#27850=ORIENTED_EDGE ( 'NONE', *, *, #16519, .F. ) ;
#27861=CARTESIAN_POINT ( 'NONE',  ( 18.91875000122903216, -5.773502691896255534, -1.060575238724906372E-15 ) ) ;
#27876=CARTESIAN_POINT ( 'NONE',  ( 26.29687500061451644, -2.746126346562646425, 4.756430356249996549 ) ) ;
#27881=CARTESIAN_POINT ( 'NONE',  ( 28.04999999999999716, 4.330127018922192761, -2.499999999999997780 ) ) ;
#27886=( BOUNDED_CURVE ( )  B_SPLINE_CURVE ( 2, ( #47709, #31457, #43282, #36991, #8191, #70248, #64702 ),
 .UNSPECIFIED., .F., .F. ) 
 B_SPLINE_CURVE_WITH_KNOTS ( ( 3, 2, 2, 3 ),
 ( 0.6800000000000001599, 0.6833333333333334592, 0.6866666666666667584, 0.6900000000000000577 ),
 .UNSPECIFIED. ) 
 CURVE ( )  GEOMETRIC_REPRESENTATION_ITEM ( )  RATIONAL_B_SPLINE_CURVE ( ( 0.9999999999999955591, 0.8660254037844431485, 1.000000000000000000, 0.8660254037844387076, 1.000000000000000000, 0.8660254037844342667, 1.000000000000004441 ) ) 
 REPRESENTATION_ITEM ( '' )  );
#27887=CARTESIAN_POINT ( 'NONE',  ( 8.737500000000002487, 5.773502691896255534, 3.535250795749688401E-16 ) ) ;
#27889=CARTESIAN_POINT ( 'NONE',  ( 10.66875000122903216, 2.886751345948126879, 4.999999999999999112 ) ) ;
#27892=CARTESIAN_POINT ( 'NONE',  ( 21.34687500061451715, -4.119189519843965641, -2.378215178125001383 ) ) ;
#27903=CARTESIAN_POINT ( 'NONE',  ( 13.88437500061451502, 5.492252693125287522, 3.363034840372157021E-16 ) ) ;
#27906=EDGE_CURVE ( 'NONE', #27013, #65422, #2257, .T. ) ;
#27917=VERTEX_POINT ( 'NONE', #33521 ) ;
#27927=CARTESIAN_POINT ( 'NONE',  ( 14.63437500061451679, -4.119189519843968306, 2.378215178124996054 ) ) ;
#27945=CARTESIAN_POINT ( 'NONE',  ( 26.19375000122903785, -2.886751345948125991, -5.000000000000000000 ) ) ;
#27975=CARTESIAN_POINT ( 'NONE',  ( 24.48749999999999716, 5.773502691896255534, 3.535250795749688401E-16 ) ) ;
#27978=( BOUNDED_CURVE ( )  B_SPLINE_CURVE ( 2, ( #10795, #55142, #10435, #55502, #4175, #4898, #33330 ),
 .UNSPECIFIED., .F., .F. ) 
 B_SPLINE_CURVE_WITH_KNOTS ( ( 3, 2, 2, 3 ),
 ( 0.2499999999999999722, 0.2533333333333333548, 0.2566666666666667096, 0.2600000000000000644 ),
 .UNSPECIFIED. ) 
 CURVE ( )  GEOMETRIC_REPRESENTATION_ITEM ( )  RATIONAL_B_SPLINE_CURVE ( ( 1.000000000000001110, 0.8660254037844374864, 1.000000000000000000, 0.8660254037844387076, 1.000000000000000000, 0.8660254037844364872, 1.000000000000002220 ) ) 
 REPRESENTATION_ITEM ( '' )  );
#27988=ORIENTED_EDGE ( 'NONE', *, *, #57093, .F. ) ;
#27995=CARTESIAN_POINT ( 'NONE',  ( 21.08437500061451786, 5.492252693125287522, 3.363034840372157021E-16 ) ) ;
#28006=CARTESIAN_POINT ( 'NONE',  ( 10.42500000000000071, 6.123233995736764310E-16, -4.999999999999998224 ) ) ;
#28012=CARTESIAN_POINT ( 'NONE',  ( 22.34999999999999787, 0.000000000000000000, 4.999999999999998224 ) ) ;
#28013=CARTESIAN_POINT ( 'NONE',  ( 23.10937500061451644, 0.000000000000000000, 4.756430356249998326 ) ) ;
#28016=DIRECTION ( 'NONE',  ( -1.000000000000000000, -0.000000000000000000, -0.000000000000000000 ) ) ;
#28035=CARTESIAN_POINT ( 'NONE',  ( 8.484375000614518214, 5.824947211148865298E-16, -4.756430356249998326 ) ) ;
#28057=CARTESIAN_POINT ( 'NONE',  ( 12.23437500061451821, 4.119189519843966529, 2.378215178124999607 ) ) ;
#28066=LINE ( 'NONE', #5164, #40877 ) ;
#28067=CARTESIAN_POINT ( 'NONE',  ( 12.54375000122903572, -2.886751345948130876, 4.999999999999996447 ) ) ;
#28074=DIRECTION ( 'NONE',  ( 0.000000000000000000, 0.000000000000000000, 1.000000000000000000 ) ) ;
#28075=EDGE_CURVE ( 'NONE', #35566, #2080, #42400, .T. ) ;
#28077=CARTESIAN_POINT ( 'NONE',  ( 20.22187500061451715, 4.119189519843966529, 2.378215178124999607 ) ) ;
#28080=CARTESIAN_POINT ( 'NONE',  ( 14.64375000122903181, 5.773502691896255534, 3.535250795749688894E-16 ) ) ;
#28088=CARTESIAN_POINT ( 'NONE',  ( 15.84375000122903643, -2.886751345948237457, -4.999999999999807265 ) ) ;
#28094=CARTESIAN_POINT ( 'NONE',  ( 7.921875000614517326, 5.824947211148865298E-16, -4.756430356249998326 ) ) ;
#28116=CARTESIAN_POINT ( 'NONE',  ( 15.34687500061451892, 5.492252693125287522, 3.363034840372157021E-16 ) ) ;
#28145=VERTEX_POINT ( 'NONE', #72331 ) ;
#28148=CARTESIAN_POINT ( 'NONE',  ( 17.89687500061451431, -2.746126346562642428, -4.756430356249999214 ) ) ;
#28154=CARTESIAN_POINT ( 'NONE',  ( 20.51249999999999929, 2.886751345948126879, 4.999999999999999112 ) ) ;
#28158=CARTESIAN_POINT ( 'NONE',  ( 25.62187500061451573, 4.119189519843966529, 2.378215178124999607 ) ) ;
#28159=CARTESIAN_POINT ( 'NONE',  ( 18.35625000122903216, 0.000000000000000000, 4.999999999999998224 ) ) ;
#28164=EDGE_CURVE ( 'NONE', #71509, #40722, #22441, .T. ) ;
#28166=CARTESIAN_POINT ( 'NONE',  ( 28.09687500061451715, -4.119189519843965641, -2.378215178125001383 ) ) ;
#28168=CARTESIAN_POINT ( 'NONE',  ( 10.95937500061451608, -5.492252693125287522, -1.008910452111647106E-15 ) ) ;
#28171=ORIENTED_EDGE ( 'NONE', *, *, #17037, .T. ) ;
#28177=DIRECTION ( 'NONE',  ( -1.000000000000000000, -0.000000000000000000, -0.000000000000000000 ) ) ;
#28191=VERTEX_POINT ( 'NONE', #55706 ) ;
#28201=CARTESIAN_POINT ( 'NONE',  ( 24.72187500061451360, 2.746126346562645981, -4.756430356249997438 ) ) ;
#28219=CARTESIAN_POINT ( 'NONE',  ( 16.21875000122903288, -5.773502691896255534, -1.060575238724906372E-15 ) ) ;
#28227=DIRECTION ( 'NONE',  ( -1.000000000000000000, -0.000000000000000000, -0.000000000000000000 ) ) ;
#28233=CARTESIAN_POINT ( 'NONE',  ( 26.70937500061451431, 0.000000000000000000, 4.756430356249998326 ) ) ;
#28238=CARTESIAN_POINT ( 'NONE',  ( 26.32499999999999929, 4.330127018922191873, 2.499999999999999556 ) ) ;
#28247=CARTESIAN_POINT ( 'NONE',  ( 11.53125000122903465, 4.330127018922191873, 2.499999999999999556 ) ) ;
#28251=CARTESIAN_POINT ( 'NONE',  ( 21.75937500061451146, -5.492252693125287522, -1.008910452111647106E-15 ) ) ;
#28254=ORIENTED_EDGE ( 'NONE', *, *, #34819, .T. ) ;
#28262=CARTESIAN_POINT ( 'NONE',  ( 12.75937500061451502, -5.492252693125287522, -1.008910452111647106E-15 ) ) ;
#28285=CARTESIAN_POINT ( 'NONE',  ( 29.37187500061451573, -4.119189519843968306, 2.378215178124996054 ) ) ;
#28286=CARTESIAN_POINT ( 'NONE',  ( 12.57187500061451857, 2.746126346562645981, -4.756430356249997438 ) ) ;
#28295=CARTESIAN_POINT ( 'NONE',  ( 11.75625000122903430, -4.330127018922190985, -2.500000000000001332 ) ) ;
#28302=CARTESIAN_POINT ( 'NONE',  ( 25.89375000122903003, 5.773502691896255534, 3.535250795749688894E-16 ) ) ;
#28337=CARTESIAN_POINT ( 'NONE',  ( 27.69375000122903074, 5.773502691896255534, 3.535250795749688401E-16 ) ) ;
#28345=CARTESIAN_POINT ( 'NONE',  ( 19.32187500061451857, 4.119189519843966529, 2.378215178124999607 ) ) ;
#28349=CARTESIAN_POINT ( 'NONE',  ( 34.99999999999999289, -2.499999999999999556, -3.499999999999999556 ) ) ;
#28361=CARTESIAN_POINT ( 'NONE',  ( 18.30000000000000071, 0.000000000000000000, 4.999999999999998224 ) ) ;
#28362=CARTESIAN_POINT ( 'NONE',  ( 20.70937500061451786, 4.119189519843966529, -2.378215178124998275 ) ) ;
#28365=( NAMED_UNIT ( * ) SI_UNIT ( $, .STERADIAN. ) SOLID_ANGLE_UNIT ( ) );
#28395=ORIENTED_EDGE ( 'NONE', *, *, #15666, .F. ) ;
#28397=CARTESIAN_POINT ( 'NONE',  ( 17.68125000122903501, 6.123233995736764310E-16, -4.999999999999998224 ) ) ;
#28405=CARTESIAN_POINT ( 'NONE',  ( 17.83125000122903003, 4.330127018922191873, 2.499999999999999556 ) ) ;
#28407=CARTESIAN_POINT ( 'NONE',  ( 9.646875000614516082, -2.746126346562646425, 4.756430356249996549 ) ) ;
#28417=CARTESIAN_POINT ( 'NONE',  ( 12.22499999999999964, 6.123233995736764310E-16, -4.999999999999998224 ) ) ;
#28421=CARTESIAN_POINT ( 'NONE',  ( 25.10625000122903216, 0.000000000000000000, 4.999999999999998224 ) ) ;
#28427=CARTESIAN_POINT ( 'NONE',  ( 17.29687500061451644, -4.119189519843965641, -2.378215178125001383 ) ) ;
#28430=CARTESIAN_POINT ( 'NONE',  ( 26.44687500061451502, 4.119189519843966529, -2.378215178124998275 ) ) ;
#28439=CARTESIAN_POINT ( 'NONE',  ( 15.69375000122903074, -2.886751345948130876, 4.999999999999996447 ) ) ;
#28445=CARTESIAN_POINT ( 'NONE',  ( 28.77187500061451431, 2.746126346562645981, -4.756430356249997438 ) ) ;
#28451=LINE ( 'NONE', #16988, #44330 ) ;
#28453=CARTESIAN_POINT ( 'NONE',  ( 11.19375000122903074, -2.886751345948074920, 5.000000000000092371 ) ) ;
#28466=CARTESIAN_POINT ( 'NONE',  ( 14.44687500061451679, 5.492252693125287522, 3.363034840372157021E-16 ) ) ;
#28470=VERTEX_POINT ( 'NONE', #63048 ) ;
#28480=ORIENTED_EDGE ( 'NONE', *, *, #60445, .T. ) ;
#28498=CARTESIAN_POINT ( 'NONE',  ( 16.62187500061451573, 2.746126346562645981, -4.756430356249997438 ) ) ;
#28503=CARTESIAN_POINT ( 'NONE',  ( 20.24999999999999645, -4.330127018922190985, -2.500000000000001332 ) ) ;
#28507=CARTESIAN_POINT ( 'NONE',  ( 25.43437500061451573, -2.746126346562641984, -4.756430356249999214 ) ) ;
#28514=CARTESIAN_POINT ( 'NONE',  ( 23.93437500061451573, -2.746126346562646425, 4.756430356249996549 ) ) ;
#28516=CARTESIAN_POINT ( 'NONE',  ( 11.33437500061451608, -2.746126346562646425, 4.756430356249996549 ) ) ;
#28528=ORIENTED_EDGE ( 'NONE', *, *, #64115, .F. ) ;
#28533=EDGE_CURVE ( 'NONE', #43273, #51781, #67437, .T. ) ;
#28554=CARTESIAN_POINT ( 'NONE',  ( 22.65937500061451715, 0.000000000000000000, 4.756430356249998326 ) ) ;
#28562=CARTESIAN_POINT ( 'NONE',  ( 27.29999999999999716, 0.000000000000000000, 4.999999999999998224 ) ) ;
#28573=CARTESIAN_POINT ( 'NONE',  ( 16.33125000122903359, 6.123233995736764310E-16, -4.999999999999998224 ) ) ;
#28589=CARTESIAN_POINT ( 'NONE',  ( 25.80937500061451928, 0.000000000000000000, 4.756430356249998326 ) ) ;
#28593=( BOUNDED_CURVE ( )  B_SPLINE_CURVE ( 2, ( #46137, #47223, #6974, #36134, #8060, #41324, #69754 ),
 .UNSPECIFIED., .F., .F. ) 
 B_SPLINE_CURVE_WITH_KNOTS ( ( 3, 2, 2, 3 ),
 ( 0.6199999999999999956, 0.6233333333333332948, 0.6266666666666667052, 0.6300000000000000044 ),
 .UNSPECIFIED. ) 
 CURVE ( )  GEOMETRIC_REPRESENTATION_ITEM ( )  RATIONAL_B_SPLINE_CURVE ( ( 1.000000000000000000, 0.8660254037844387076, 1.000000000000000000, 0.8660254037844387076, 1.000000000000000000, 0.8660254037844387076, 1.000000000000000000 ) ) 
 REPRESENTATION_ITEM ( '' )  );
#28595=CARTESIAN_POINT ( 'NONE',  ( 27.67499999999999716, 4.330127018922191873, 2.499999999999999556 ) ) ;
#28603=CARTESIAN_POINT ( 'NONE',  ( 11.60625000122903216, 0.000000000000000000, 4.999999999999998224 ) ) ;
#28607=CARTESIAN_POINT ( 'NONE',  ( 17.78437500061451360, -2.746126346562641984, -4.756430356249999214 ) ) ;
#28617=CARTESIAN_POINT ( 'NONE',  ( 13.47187500061451715, 4.119189519843966529, 2.378215178124999607 ) ) ;
#28624=CARTESIAN_POINT ( 'NONE',  ( 13.79999999999999893, 0.000000000000000000, 4.999999999999998224 ) ) ;
#28626=CARTESIAN_POINT ( 'NONE',  ( 12.22499999999999964, 6.123233995736764310E-16, -4.999999999999998224 ) ) ;
#28640=CARTESIAN_POINT ( 'NONE',  ( 22.48125000122903216, -4.330127018922194537, 2.499999999999995559 ) ) ;
#28641=CARTESIAN_POINT ( 'NONE',  ( 12.94687500061451857, -2.746126346562642428, -4.756430356249999214 ) ) ;
#28658=CARTESIAN_POINT ( 'NONE',  ( 22.44375000122903074, -2.886751345948129988, 4.999999999999997335 ) ) ;
#28701=ADVANCED_FACE ( 'NONE', ( #40532 ), #34981, .T. ) ;
#28705=CARTESIAN_POINT ( 'NONE',  ( 18.60937500061451289, -5.492252693125287522, -1.008910452111647106E-15 ) ) ;
#28720=CARTESIAN_POINT ( 'NONE',  ( 20.10937500061451289, -4.119189519843965641, -2.378215178125001383 ) ) ;
#28723=CARTESIAN_POINT ( 'NONE',  ( 28.40625000122903288, -4.330127018922190985, -2.500000000000001332 ) ) ;
#28738=CARTESIAN_POINT ( 'NONE',  ( 45.00000000000000000, 6.123233995736764310E-16, -4.999999999999998224 ) ) ;
#28765=CARTESIAN_POINT ( 'NONE',  ( 9.421875000614519990, 2.746126346562645981, -4.756430356249997438 ) ) ;
#28786=CARTESIAN_POINT ( 'NONE',  ( 18.53437500061451360, -2.746126346562646425, 4.756430356249996549 ) ) ;
#28789=CARTESIAN_POINT ( 'NONE',  ( 26.63437500061451146, -2.746126346562646425, 4.756430356249996549 ) ) ;
#28797=LINE ( 'NONE', #16976, #38410 ) ;
#28803=CARTESIAN_POINT ( 'NONE',  ( 26.25937500061451857, 0.000000000000000000, 4.756430356249998326 ) ) ;
#28814=ORIENTED_EDGE ( 'NONE', *, *, #15629, .F. ) ;
#28824=CARTESIAN_POINT ( 'NONE',  ( 14.93437500061451750, 4.119189519843966529, 2.378215178124999607 ) ) ;
#28828=ORIENTED_EDGE ( 'NONE', *, *, #1636, .T. ) ;
#28838=CARTESIAN_POINT ( 'NONE',  ( 21.97500000000000142, -4.330127018922194537, 2.499999999999995559 ) ) ;
#28855=CARTESIAN_POINT ( 'NONE',  ( 15.38437500061451679, 4.119189519843966529, 2.378215178124999607 ) ) ;
#28859=AXIS2_PLACEMENT_3D ( 'NONE', #7281, #24623, #7637 ) ;
#28863=CARTESIAN_POINT ( 'NONE',  ( 16.46249999999999503, 2.886751345948126879, 4.999999999999999112 ) ) ;
#28867=CARTESIAN_POINT ( 'NONE',  ( 25.32187500061451502, -4.119189519843968306, 2.378215178124996054 ) ) ;
#28875=CARTESIAN_POINT ( 'NONE',  ( 25.13437500061451857, 5.492252693125287522, 3.363034840372157021E-16 ) ) ;
#28877=CARTESIAN_POINT ( 'NONE',  ( 12.19687500061451502, 0.000000000000000000, 4.756430356249998326 ) ) ;
#28884=ADVANCED_FACE ( 'NONE', ( #19422 ), #2452, .T. ) ;
#28886=CARTESIAN_POINT ( 'NONE',  ( 45.00000000000000000, 6.123233995736764310E-16, -4.999999999999998224 ) ) ;
#28887=CARTESIAN_POINT ( 'NONE',  ( 17.69999999999999929, 4.330127018922192761, -2.499999999999997780 ) ) ;
#28890=CARTESIAN_POINT ( 'NONE',  ( 12.34687500061451537, -4.119189519843965641, -2.378215178125001383 ) ) ;
#28902=EDGE_LOOP ( 'NONE', ( #5516, #33510, #19325, #2947 ) ) ;
#28910=AXIS2_PLACEMENT_3D ( 'NONE', #48611, #36786, #8712 ) ;
#28912=CARTESIAN_POINT ( 'NONE',  ( 22.84687500061451715, -2.746126346562641984, -4.756430356249999214 ) ) ;
#28919=VERTEX_POINT ( 'NONE', #70420 ) ;
#28925=LINE ( 'NONE', #6032, #60433 ) ;
#28934=CARTESIAN_POINT ( 'NONE',  ( 16.89375000122903359, 5.773502691896255534, 3.535250795749688894E-16 ) ) ;
#28946=ORIENTED_EDGE ( 'NONE', *, *, #31978, .F. ) ;
#28950=CARTESIAN_POINT ( 'NONE',  ( 23.89687500061451786, 5.492252693125287522, 3.363034840372157021E-16 ) ) ;
#28955=CARTESIAN_POINT ( 'NONE',  ( 28.16249999999999787, 2.886751345948126879, 4.999999999999999112 ) ) ;
#28966=CARTESIAN_POINT ( 'NONE',  ( 8.981250001229033941, -4.330127018922194537, 2.499999999999995559 ) ) ;
#28970=CARTESIAN_POINT ( 'NONE',  ( 18.64687500061451431, -4.119189519843965641, -2.378215178125001383 ) ) ;
#28982=CARTESIAN_POINT ( 'NONE',  ( 10.54687500061451644, -4.119189519843965641, -2.378215178125001383 ) ) ;
#29004=CARTESIAN_POINT ( 'NONE',  ( 28.35937500061451289, 4.119189519843966529, -2.378215178124998275 ) ) ;
#29007=CARTESIAN_POINT ( 'NONE',  ( 27.72187500061451715, 5.824947211148865298E-16, -4.756430356249998326 ) ) ;
#29008=CARTESIAN_POINT ( 'NONE',  ( 13.13437500061451857, 4.119189519843966529, 2.378215178124999607 ) ) ;
#29024=DIRECTION ( 'NONE',  ( -1.000000000000000000, -0.000000000000000000, -0.000000000000000000 ) ) ;
#29025=CARTESIAN_POINT ( 'NONE',  ( 22.96875000122903643, -5.773502691896255534, -1.060575238724906372E-15 ) ) ;
#29027=CARTESIAN_POINT ( 'NONE',  ( 45.00000000000000000, 6.123233995736764310E-16, -4.999999999999998224 ) ) ;
#29059=CARTESIAN_POINT ( 'NONE',  ( 17.88749999999999929, -2.886751345948074920, 5.000000000000092371 ) ) ;
#29075=CARTESIAN_POINT ( 'NONE',  ( 19.35937500061451644, 2.746126346562643317, 4.756430356249998326 ) ) ;
#29092=CARTESIAN_POINT ( 'NONE',  ( 20.82187500061451857, 2.746126346562643317, 4.756430356249998326 ) ) ;
#29107=AXIS2_PLACEMENT_3D ( 'NONE', #14663, #70465, #37206 ) ;
#29108=CARTESIAN_POINT ( 'NONE',  ( 21.44999999999999929, 0.000000000000000000, 4.999999999999998224 ) ) ;
#29114=CARTESIAN_POINT ( 'NONE',  ( 8.334375000614516082, -4.119189519843968306, 2.378215178124996054 ) ) ;
#29115=CARTESIAN_POINT ( 'NONE',  ( 14.88749999999999929, -2.886751345948126435, -5.000000000000000000 ) ) ;
#29125=ORIENTED_EDGE ( 'NONE', *, *, #31318, .T. ) ;
#29126=VERTEX_POINT ( 'NONE', #25719 ) ;
#29135=CARTESIAN_POINT ( 'NONE',  ( 17.71875000122903288, 2.886751345948129099, -4.999999999999997335 ) ) ;
#29136=CARTESIAN_POINT ( 'NONE',  ( 8.859375000614518214, -4.119189519843965641, -2.378215178125001383 ) ) ;
#29158=CARTESIAN_POINT ( 'NONE',  ( 16.88437500061451857, -2.746126346562642428, -4.756430356249999214 ) ) ;
#29161=CARTESIAN_POINT ( 'NONE',  ( 26.18437500061451573, -2.746126346562646425, 4.756430356249996549 ) ) ;
#29174=CARTESIAN_POINT ( 'NONE',  ( 28.02187500061451431, 2.746126346562643317, 4.756430356249998326 ) ) ;
#29181=CARTESIAN_POINT ( 'NONE',  ( 14.58750000000000036, 5.773502691896255534, 3.535250795749688401E-16 ) ) ;
#29193=CARTESIAN_POINT ( 'NONE',  ( 14.37187500061451750, 2.746126346562645981, -4.756430356249997438 ) ) ;
#29205=DIRECTION ( 'NONE',  ( -1.000000000000000000, -0.000000000000000000, -0.000000000000000000 ) ) ;
#29223=CARTESIAN_POINT ( 'NONE',  ( 16.20937500061451786, 4.119189519843966529, -2.378215178124998275 ) ) ;
#29233=CARTESIAN_POINT ( 'NONE',  ( 17.69999999999999929, 4.330127018922192761, -2.499999999999997780 ) ) ;
#29236=DIRECTION ( 'NONE',  ( -1.000000000000000000, 0.000000000000000000, 0.000000000000000000 ) ) ;
#29237=CARTESIAN_POINT ( 'NONE',  ( 24.04687500061451289, -4.119189519843965641, -2.378215178125001383 ) ) ;
#29238=CARTESIAN_POINT ( 'NONE',  ( 34.99999999999999289, 2.500000000000000000, -3.500000000000000000 ) ) ;
#29244=CARTESIAN_POINT ( 'NONE',  ( 25.95937500061451431, 2.746126346562645981, -4.756430356249997438 ) ) ;
#29246=CARTESIAN_POINT ( 'NONE',  ( 11.85937500061451644, -5.492252693125287522, -1.008910452111647106E-15 ) ) ;
#29249=ORIENTED_EDGE ( 'NONE', *, *, #22798, .F. ) ;
#29254=EDGE_CURVE ( 'NONE', #40553, #49807, #33960, .T. ) ;
#29255=AXIS2_PLACEMENT_3D ( 'NONE', #7874, #70658, #20032 ) ;
#29256=CARTESIAN_POINT ( 'NONE',  ( 45.00000000000000000, 6.123233995736764310E-16, -4.999999999999998224 ) ) ;
#29259=CARTESIAN_POINT ( 'NONE',  ( 12.08437500061451608, 5.492252693125287522, 3.363034840372157021E-16 ) ) ;
#29276=FACE_OUTER_BOUND ( 'NONE', #51031, .T. ) ;
#29278=CARTESIAN_POINT ( 'NONE',  ( 21.79687500061451644, -2.746126346562646425, 4.756430356249996549 ) ) ;
#29280=CARTESIAN_POINT ( 'NONE',  ( 25.06875000122902719, 2.886751345948140646, 4.999999999999974243 ) ) ;
#29295=FACE_OUTER_BOUND ( 'NONE', #52672, .T. ) ;
#29298=CARTESIAN_POINT ( 'NONE',  ( 16.29375000122903216, -2.886751345948125991, -5.000000000000000000 ) ) ;
#29307=CARTESIAN_POINT ( 'NONE',  ( 10.65000000000000036, 0.000000000000000000, 4.999999999999998224 ) ) ;
#29314=CARTESIAN_POINT ( 'NONE',  ( 23.07187500061451857, 2.746126346562643317, 4.756430356249998326 ) ) ;
#29321=CARTESIAN_POINT ( 'NONE',  ( 25.61250000000000071, -5.773502691896255534, -1.060575238724906372E-15 ) ) ;
#29330=CARTESIAN_POINT ( 'NONE',  ( 8.568750001229034297, -5.773502691896255534, -1.060575238724906372E-15 ) ) ;
#29333=CARTESIAN_POINT ( 'NONE',  ( 17.22187500061451360, -4.119189519843968306, 2.378215178124996054 ) ) ;
#29343=DIRECTION ( 'NONE',  ( -1.000000000000000000, -0.000000000000000000, -0.000000000000000000 ) ) ;
#29344=CARTESIAN_POINT ( 'NONE',  ( 10.13437500061451502, -2.746126346562642428, -4.756430356249999214 ) ) ;
#29351=CARTESIAN_POINT ( 'NONE',  ( 13.57500000000000107, 6.123233995736764310E-16, -4.999999999999998224 ) ) ;
#29357=CARTESIAN_POINT ( 'NONE',  ( 9.787499999999999645, -2.886751345948129988, 4.999999999999997335 ) ) ;
#29369=CARTESIAN_POINT ( 'NONE',  ( 27.00937500061451502, 2.746126346562643317, 4.756430356249998326 ) ) ;
#29370=CARTESIAN_POINT ( 'NONE',  ( 12.27187500061451786, 2.746126346562643317, 4.756430356249998326 ) ) ;
#29385=CYLINDRICAL_SURFACE ( 'NONE', #33944, 4.999999999999998224 ) ;
#29386=CARTESIAN_POINT ( 'NONE',  ( 23.00625000122903430, -4.330127018922190985, -2.500000000000001332 ) ) ;
#29412=CARTESIAN_POINT ( 'NONE',  ( -5.000000000000004441, 6.123233995736764310E-16, -4.999999999999998224 ) ) ;
#29416=CARTESIAN_POINT ( 'NONE',  ( 23.92499999999999716, 6.123233995736764310E-16, -4.999999999999998224 ) ) ;
#29422=VERTEX_POINT ( 'NONE', #60960 ) ;
#29426=CARTESIAN_POINT ( 'NONE',  ( 30.00000000000000000, 0.000000000000000000, 4.999999999999998224 ) ) ;
#29434=CARTESIAN_POINT ( 'NONE',  ( 19.77187500061451786, 4.119189519843966529, 2.378215178124999607 ) ) ;
#29449=CARTESIAN_POINT ( 'NONE',  ( 45.00000000000000000, 0.000000000000000000, 4.999999999999998224 ) ) ;
#29450=CARTESIAN_POINT ( 'NONE',  ( 19.88437500061451857, 4.119189519843966529, 2.378215178124999607 ) ) ;
#29473=CARTESIAN_POINT ( 'NONE',  ( 7.659375000614518036, 4.119189519843966529, -2.378215178124998275 ) ) ;
#29474=CYLINDRICAL_SURFACE ( 'NONE', #38362, 4.999999999999998224 ) ;
#29483=ORIENTED_EDGE ( 'NONE', *, *, #71543, .F. ) ;
#29495=CARTESIAN_POINT ( 'NONE',  ( 8.146875000614516082, 5.492252693125287522, 3.363034840372157021E-16 ) ) ;
#29497=CYLINDRICAL_SURFACE ( 'NONE', #61854, 4.999999999999998224 ) ;
#29507=CARTESIAN_POINT ( 'NONE',  ( 12.65625000122903110, -4.330127018922190985, -2.500000000000001332 ) ) ;
#29516=CARTESIAN_POINT ( 'NONE',  ( 17.25937500061451502, -5.492252693125287522, -1.008910452111647106E-15 ) ) ;
#29519=CARTESIAN_POINT ( 'NONE',  ( 26.70937500061451431, -5.492252693125287522, -1.008910452111647106E-15 ) ) ;
#29523=CARTESIAN_POINT ( 'NONE',  ( 45.00000000000000000, 2.500000000000000444, 3.499999999999999112 ) ) ;
#29533=CARTESIAN_POINT ( 'NONE',  ( 27.64687500061452141, -2.746126346562646425, 4.756430356249996549 ) ) ;
#29551=CARTESIAN_POINT ( 'NONE',  ( 14.10937500061451644, 0.000000000000000000, 4.756430356249998326 ) ) ;
#29582=CARTESIAN_POINT ( 'NONE',  ( 16.09687500061452070, -2.746126346562642428, -4.756430356249999214 ) ) ;
#29588=CARTESIAN_POINT ( 'NONE',  ( 18.22499999999999787, 4.330127018922191873, 2.499999999999999556 ) ) ;
#29592=CARTESIAN_POINT ( 'NONE',  ( 23.67187500061451289, 5.824947211148865298E-16, -4.756430356249998326 ) ) ;
#29600=CARTESIAN_POINT ( 'NONE',  ( 25.62187500061451573, 4.119189519843966529, 2.378215178124999607 ) ) ;
#29602=CARTESIAN_POINT ( 'NONE',  ( 10.77187500061451608, 4.119189519843966529, 2.378215178124999607 ) ) ;
#29611=CARTESIAN_POINT ( 'NONE',  ( 15.86250000000000071, 2.886751345948073588, -5.000000000000094147 ) ) ;
#29614=CARTESIAN_POINT ( 'NONE',  ( 12.64687500061451786, 0.000000000000000000, 4.756430356249998326 ) ) ;
#29633=CARTESIAN_POINT ( 'NONE',  ( 23.03437500061451715, 4.119189519843966529, 2.378215178124999607 ) ) ;
#29650=CARTESIAN_POINT ( 'NONE',  ( 28.57499999999999929, 4.330127018922191873, 2.499999999999999556 ) ) ;
#29655=CARTESIAN_POINT ( 'NONE',  ( 10.21875000122902932, 2.886751345948238789, 4.999999999999807265 ) ) ;
#29666=ORIENTED_EDGE ( 'NONE', *, *, #1611, .F. ) ;
#29670=CARTESIAN_POINT ( 'NONE',  ( 23.85937500061451644, 4.119189519843966529, -2.378215178124998275 ) ) ;
#29673=CARTESIAN_POINT ( 'NONE',  ( 29.25000000000000000, -4.330127018922190985, -2.500000000000001332 ) ) ;
#29676=CARTESIAN_POINT ( 'NONE',  ( 24.29999999999999716, -4.330127018922190985, -2.500000000000001332 ) ) ;
#29683=CARTESIAN_POINT ( 'NONE',  ( 15.26249999999999929, -5.773502691896255534, -1.060575238724906372E-15 ) ) ;
#29685=CARTESIAN_POINT ( 'NONE',  ( 8.793750001229033941, 5.773502691896255534, 3.535250795749688894E-16 ) ) ;
#29688=CARTESIAN_POINT ( 'NONE',  ( 18.53437500061451360, -2.746126346562646425, 4.756430356249996549 ) ) ;
#29699=CARTESIAN_POINT ( 'NONE',  ( 9.721875000614517148, 5.824947211148865298E-16, -4.756430356249998326 ) ) ;
#29712=CARTESIAN_POINT ( 'NONE',  ( 10.46249999999999858, 2.886751345948129099, -4.999999999999998224 ) ) ;
#29720=CARTESIAN_POINT ( 'NONE',  ( 29.14687500061451431, -2.746126346562641984, -4.756430356249999214 ) ) ;
#29722=CARTESIAN_POINT ( 'NONE',  ( 27.12187500061451573, -4.119189519843968306, 2.378215178124996054 ) ) ;
#29723=CARTESIAN_POINT ( 'NONE',  ( 13.54687500061451999, 5.492252693125287522, 3.363034840372157021E-16 ) ) ;
#29725=EDGE_CURVE ( 'NONE', #4282, #59530, #51880, .T. ) ;
#29730=DIRECTION ( 'NONE',  ( -1.000000000000000000, -0.000000000000000000, -0.000000000000000000 ) ) ;
#29732=CARTESIAN_POINT ( 'NONE',  ( 29.74687500061451573, 0.000000000000000000, 4.756430356249998326 ) ) ;
#29740=CARTESIAN_POINT ( 'NONE',  ( 24.46875000122903288, 2.886751345948129099, -4.999999999999998224 ) ) ;
#29748=CARTESIAN_POINT ( 'NONE',  ( 29.02499999999999858, 4.330127018922191873, 2.499999999999999556 ) ) ;
#29751=VECTOR ( 'NONE', #70777, 1000.000000000000000 ) ;
#29764=CARTESIAN_POINT ( 'NONE',  ( 22.18125000122903145, 6.123233995736764310E-16, -4.999999999999998224 ) ) ;
#29765=ADVANCED_FACE ( 'NONE', ( #35734 ), #29474, .T. ) ;
#29770=CARTESIAN_POINT ( 'NONE',  ( 23.73749999999999716, -2.886751345948130876, 4.999999999999996447 ) ) ;
#29774=CARTESIAN_POINT ( 'NONE',  ( 16.33125000122903359, 6.123233995736764310E-16, -4.999999999999998224 ) ) ;
#29788=EDGE_LOOP ( 'NONE', ( #14515, #30380, #18332, #4563 ) ) ;
#29792=CARTESIAN_POINT ( 'NONE',  ( 17.78437500061451360, -2.746126346562642428, -4.756430356249999214 ) ) ;
#29800=CARTESIAN_POINT ( 'NONE',  ( 45.00000000000000000, 0.000000000000000000, 0.000000000000000000 ) ) ;
#29811=CARTESIAN_POINT ( 'NONE',  ( 21.04687500061451644, -2.746126346562642428, -4.756430356249999214 ) ) ;
#29831=LINE ( 'NONE', #69370, #51375 ) ;
#29834=CARTESIAN_POINT ( 'NONE',  ( 22.63125000122903430, 6.123233995736764310E-16, -4.999999999999998224 ) ) ;
#29855=CARTESIAN_POINT ( 'NONE',  ( 9.159375000614515372, 0.000000000000000000, 4.756430356249998326 ) ) ;
#29861=CARTESIAN_POINT ( 'NONE',  ( 28.78125000122903288, -4.330127018922194537, 2.499999999999995559 ) ) ;
#29864=LINE ( 'NONE', #18400, #19655 ) ;
#29874=CARTESIAN_POINT ( 'NONE',  ( 17.67187500061451644, -4.119189519843968306, 2.378215178124996054 ) ) ;
#29877=CARTESIAN_POINT ( 'NONE',  ( 25.39687500061451431, -4.119189519843965641, -2.378215178125001383 ) ) ;
#29891=CARTESIAN_POINT ( 'NONE',  ( 27.15937500061451360, 0.000000000000000000, 4.756430356249998326 ) ) ;
#29895=CARTESIAN_POINT ( 'NONE',  ( 18.93749999999999645, -2.886751345948181946, -4.999999999999904077 ) ) ;
#29910=CARTESIAN_POINT ( 'NONE',  ( 13.35937500061451821, -4.119189519843965641, -2.378215178125001383 ) ) ;
#29912=CARTESIAN_POINT ( 'NONE',  ( 16.72500000000000142, 6.123233995736764310E-16, -4.999999999999998224 ) ) ;
#29923=ORIENTED_EDGE ( 'NONE', *, *, #25902, .F. ) ;
#29939=CARTESIAN_POINT ( 'NONE',  ( 16.69687500061451502, 5.492252693125287522, 3.363034840372157021E-16 ) ) ;
#29945=CARTESIAN_POINT ( 'NONE',  ( 18.45000000000000284, -4.330127018922190985, -2.500000000000001332 ) ) ;
#29949=CARTESIAN_POINT ( 'NONE',  ( 23.74687500061451573, 4.119189519843966529, -2.378215178124998275 ) ) ;
#29950=CARTESIAN_POINT ( 'NONE',  ( 26.36249999999999716, 2.886751345948113556, 5.000000000000023093 ) ) ;
#29956=CARTESIAN_POINT ( 'NONE',  ( 24.42187500061451289, -4.119189519843968306, 2.378215178124996054 ) ) ;
#29958=CARTESIAN_POINT ( 'NONE',  ( 9.121875000614517504, -4.119189519843968306, 2.378215178124996054 ) ) ;
#29968=ORIENTED_EDGE ( 'NONE', *, *, #39854, .F. ) ;
#29970=CARTESIAN_POINT ( 'NONE',  ( 10.69687500061451679, 4.119189519843966529, -2.378215178124998275 ) ) ;
#29976=EDGE_CURVE ( 'NONE', #20756, #1724, #26876, .T. ) ;
#29989=CARTESIAN_POINT ( 'NONE',  ( 22.32187500061451857, -5.492252693125287522, -1.008910452111647106E-15 ) ) ;
#29996=ORIENTED_EDGE ( 'NONE', *, *, #34066, .T. ) ;
#30020=ORIENTED_EDGE ( 'NONE', *, *, #65744, .T. ) ;
#30025=CARTESIAN_POINT ( 'NONE',  ( 23.93437500061451573, 4.119189519843966529, 2.378215178124999607 ) ) ;
#30033=CARTESIAN_POINT ( 'NONE',  ( 25.53750000000000142, -2.886751345948129988, 4.999999999999997335 ) ) ;
#30034=EDGE_CURVE ( 'NONE', #67801, #46954, #21677, .T. ) ;
#30041=CARTESIAN_POINT ( 'NONE',  ( 18.35625000122903216, 0.000000000000000000, 4.999999999999998224 ) ) ;
#30043=CARTESIAN_POINT ( 'NONE',  ( 9.768750001229035362, 2.886751345948126879, 4.999999999999999112 ) ) ;
#30046=CARTESIAN_POINT ( 'NONE',  ( 17.29687500061451644, -4.119189519843965641, -2.378215178125001383 ) ) ;
#30056=AXIS2_PLACEMENT_3D ( 'NONE', #32233, #48866, #38880 ) ;
#30060=CARTESIAN_POINT ( 'NONE',  ( 11.52187500061451608, 5.824947211148865298E-16, -4.756430356249998326 ) ) ;
#30061=ORIENTED_EDGE ( 'NONE', *, *, #66541, .T. ) ;
#30070=CARTESIAN_POINT ( 'NONE',  ( 27.53437500061451715, -2.746126346562646425, 4.756430356249996549 ) ) ;
#30073=CARTESIAN_POINT ( 'NONE',  ( 8.625000000000000000, 6.123233995736764310E-16, -4.999999999999998224 ) ) ;
#30082=CARTESIAN_POINT ( 'NONE',  ( 28.17187500061451644, -5.492252693125287522, -1.008910452111647106E-15 ) ) ;
#30084=CARTESIAN_POINT ( 'NONE',  ( 28.09687500061451715, -4.119189519843965641, -2.378215178125001383 ) ) ;
#30085=CARTESIAN_POINT ( 'NONE',  ( 9.684375000614517504, -4.119189519843968306, 2.378215178124996054 ) ) ;
#30092=( BOUNDED_CURVE ( )  B_SPLINE_CURVE ( 2, ( #62246, #56695, #16805, #60776, #38247, #43806, #28626 ),
 .UNSPECIFIED., .F., .F. ) 
 B_SPLINE_CURVE_WITH_KNOTS ( ( 3, 2, 2, 3 ),
 ( 0.7800000000000001377, 0.7833333333333334370, 0.7866666666666667362, 0.7900000000000001465 ),
 .UNSPECIFIED. ) 
 CURVE ( )  GEOMETRIC_REPRESENTATION_ITEM ( )  RATIONAL_B_SPLINE_CURVE ( ( 0.9999999999999955591, 0.8660254037844431485, 1.000000000000000000, 0.8660254037844387076, 1.000000000000000000, 0.8660254037844342667, 1.000000000000004441 ) ) 
 REPRESENTATION_ITEM ( '' )  );
#30094=CARTESIAN_POINT ( 'NONE',  ( 34.99999999999999289, 2.500000000000000444, 3.499999999999999112 ) ) ;
#30097=( NAMED_UNIT ( * ) SI_UNIT ( $, .STERADIAN. ) SOLID_ANGLE_UNIT ( ) );
#30102=CARTESIAN_POINT ( 'NONE',  ( 23.45625000122903359, -4.330127018922190985, -2.500000000000001332 ) ) ;
#30105=ORIENTED_EDGE ( 'NONE', *, *, #26979, .F. ) ;
#30110=CARTESIAN_POINT ( 'NONE',  ( 23.15625000122903288, 4.330127018922192761, -2.499999999999997780 ) ) ;
#30118=CARTESIAN_POINT ( 'NONE',  ( 29.78437500061451715, 4.119189519843966529, 2.378215178124999607 ) ) ;
#30121=VECTOR ( 'NONE', #33268, 1000.000000000000000 ) ;
#30128=CARTESIAN_POINT ( 'NONE',  ( 25.46249999999999858, 2.886751345948140646, 4.999999999999974243 ) ) ;
#30138=CARTESIAN_POINT ( 'NONE',  ( 19.40625000122902932, -4.330127018922190985, -2.500000000000001332 ) ) ;
#30141=ORIENTED_EDGE ( 'NONE', *, *, #11564, .T. ) ;
#30145=CARTESIAN_POINT ( 'NONE',  ( 27.61875000122903145, 2.886751345948142866, -4.999999999999973355 ) ) ;
#30154=CARTESIAN_POINT ( 'NONE',  ( 15.49687500061451573, -4.119189519843965641, -2.378215178125001383 ) ) ;
#30157=VECTOR ( 'NONE', #44585, 1000.000000000000000 ) ;
#30163=CARTESIAN_POINT ( 'NONE',  ( 11.60625000122903216, 0.000000000000000000, 4.999999999999998224 ) ) ;
#30164=ORIENTED_EDGE ( 'NONE', *, *, #46331, .F. ) ;
#30169=ADVANCED_FACE ( 'NONE', ( #26116 ), #25754, .T. ) ;
#30173=CARTESIAN_POINT ( 'NONE',  ( 8.268750001229030033, 2.886751345948073588, -5.000000000000094147 ) ) ;
#30176=CARTESIAN_POINT ( 'NONE',  ( 18.34687500061451715, -2.746126346562642428, -4.756430356249999214 ) ) ;
#30185=AXIS2_PLACEMENT_3D ( 'NONE', #4910, #9354, #48882 ) ;
#30187=CARTESIAN_POINT ( 'NONE',  ( 45.00000000000000000, 0.000000000000000000, 0.000000000000000000 ) ) ;
#30195=CARTESIAN_POINT ( 'NONE',  ( 19.70625000122903359, 0.000000000000000000, 4.999999999999998224 ) ) ;
#30197=CARTESIAN_POINT ( 'NONE',  ( 8.512499999999999289, -5.773502691896255534, -1.060575238724906372E-15 ) ) ;
#30198=CARTESIAN_POINT ( 'NONE',  ( 7.575000000000001954, -4.330127018922194537, 2.499999999999995559 ) ) ;
#30220=CARTESIAN_POINT ( 'NONE',  ( 28.57499999999999929, 4.330127018922191873, 2.499999999999999556 ) ) ;
#30226=EDGE_CURVE ( 'NONE', #829, #57985, #72603, .T. ) ;
#30237=CARTESIAN_POINT ( 'NONE',  ( 45.00000000000000000, 0.000000000000000000, 4.999999999999998224 ) ) ;
#30239=CARTESIAN_POINT ( 'NONE',  ( 14.33437500061451431, 5.492252693125287522, 3.363034840372157021E-16 ) ) ;
#30242=CARTESIAN_POINT ( 'NONE',  ( 23.82187500061451502, 4.119189519843966529, 2.378215178124999607 ) ) ;
#30258=CARTESIAN_POINT ( 'NONE',  ( 27.90937500061451715, 4.119189519843966529, -2.378215178124998275 ) ) ;
#30278=CARTESIAN_POINT ( 'NONE',  ( 13.39687500061451608, -2.746126346562641984, -4.756430356249999214 ) ) ;
#30291=LINE ( 'NONE', #56904, #59739 ) ;
#30292=ORIENTED_EDGE ( 'NONE', *, *, #17585, .F. ) ;
#30299=( BOUNDED_CURVE ( )  B_SPLINE_CURVE ( 2, ( #32089, #64968, #9555, #26925, #71984, #54261, #65330 ),
 .UNSPECIFIED., .F., .F. ) 
 B_SPLINE_CURVE_WITH_KNOTS ( ( 3, 2, 2, 3 ),
 ( 0.7199999999999999734, 0.7233333333333333837, 0.7266666666666666829, 0.7299999999999999822 ),
 .UNSPECIFIED. ) 
 CURVE ( )  GEOMETRIC_REPRESENTATION_ITEM ( )  RATIONAL_B_SPLINE_CURVE ( ( 1.000000000000000000, 0.8660254037844387076, 1.000000000000000000, 0.8660254037844387076, 1.000000000000000000, 0.8660254037844387076, 1.000000000000000000 ) ) 
 REPRESENTATION_ITEM ( '' )  );
#30309=CARTESIAN_POINT ( 'NONE',  ( 14.74687500061451573, -2.746126346562642428, -4.756430356249999214 ) ) ;
#30318=CARTESIAN_POINT ( 'NONE',  ( 16.87500000000000000, 4.330127018922191873, 2.499999999999999556 ) ) ;
#30321=CARTESIAN_POINT ( 'NONE',  ( 24.60000000000000142, 0.000000000000000000, 4.999999999999998224 ) ) ;
#30322=CARTESIAN_POINT ( 'NONE',  ( 22.35937500061451644, 2.746126346562645981, -4.756430356249997438 ) ) ;
#30331=CARTESIAN_POINT ( 'NONE',  ( 22.02187500061451431, 4.119189519843966529, 2.378215178124999607 ) ) ;
#30334=CARTESIAN_POINT ( 'NONE',  ( 9.009375000614515017, 2.746126346562643317, 4.756430356249998326 ) ) ;
#30341=CARTESIAN_POINT ( 'NONE',  ( 26.45625000122903003, 0.000000000000000000, 4.999999999999998224 ) ) ;
#30345=CARTESIAN_POINT ( 'NONE',  ( 11.59687500061451537, 4.119189519843966529, -2.378215178124998275 ) ) ;
#30362=CARTESIAN_POINT ( 'NONE',  ( 30.00000000000000000, 0.000000000000000000, 4.999999999999998224 ) ) ;
#30365=CARTESIAN_POINT ( 'NONE',  ( 18.38437500061451857, 5.824947211148865298E-16, -4.756430356249998326 ) ) ;
#30380=ORIENTED_EDGE ( 'NONE', *, *, #45595, .T. ) ;
#30396=EDGE_CURVE ( 'NONE', #4240, #67801, #44348, .T. ) ;
#30399=CARTESIAN_POINT ( 'NONE',  ( 22.80937500061451573, -4.119189519843965641, -2.378215178125001383 ) ) ;
#30405=CARTESIAN_POINT ( 'NONE',  ( 25.27499999999999858, 6.123233995736764310E-16, -4.999999999999998224 ) ) ;
#30413=ADVANCED_FACE ( 'NONE', ( #60816 ), #56731, .F. ) ;
#30416=CARTESIAN_POINT ( 'NONE',  ( 10.40625000122903288, -4.330127018922190985, -2.500000000000001332 ) ) ;
#30418=CARTESIAN_POINT ( 'NONE',  ( 16.28437500061451715, -2.746126346562646425, 4.756430356249996549 ) ) ;
#30430=CARTESIAN_POINT ( 'NONE',  ( 11.48437500061451821, -2.746126346562642428, -4.756430356249999214 ) ) ;
#30436=ORIENTED_EDGE ( 'NONE', *, *, #30396, .F. ) ;
#30441=CARTESIAN_POINT ( 'NONE',  ( 28.05937500061451217, -5.492252693125287522, -1.008910452111647106E-15 ) ) ;
#30444=CARTESIAN_POINT ( 'NONE',  ( 8.099999999999999645, -4.330127018922190985, -2.500000000000001332 ) ) ;
#30452=CARTESIAN_POINT ( 'NONE',  ( 26.85937500061451644, -4.119189519843965641, -2.378215178125001383 ) ) ;
#30454=CARTESIAN_POINT ( 'NONE',  ( 10.32187500061451679, 2.746126346562645981, -4.756430356249997438 ) ) ;
#30470=CARTESIAN_POINT ( 'NONE',  ( 21.80625000122903145, 4.330127018922192761, -2.499999999999997780 ) ) ;
#30473=ORIENTED_EDGE ( 'NONE', *, *, #53326, .F. ) ;
#30503=CARTESIAN_POINT ( 'NONE',  ( 7.950000000000001954, 0.000000000000000000, 4.999999999999998224 ) ) ;
#30504=LINE ( 'NONE', #42683, #34807 ) ;
#30523=CARTESIAN_POINT ( 'NONE',  ( 16.54687500061451644, 4.119189519843966529, -2.378215178124998275 ) ) ;
#30539=DIRECTION ( 'NONE',  ( -1.000000000000000000, -0.000000000000000000, -0.000000000000000000 ) ) ;
#30542=CARTESIAN_POINT ( 'NONE',  ( 18.15937500061451715, 0.000000000000000000, 4.756430356249998326 ) ) ;
#30560=CARTESIAN_POINT ( 'NONE',  ( 29.41875000122902861, 2.886751345948129099, -4.999999999999998224 ) ) ;
#30572=ORIENTED_EDGE ( 'NONE', *, *, #42868, .T. ) ;
#30573=VERTEX_POINT ( 'NONE', #70005 ) ;
#30585=CARTESIAN_POINT ( 'NONE',  ( 29.66249999999999432, -5.773502691896255534, -1.060575238724906372E-15 ) ) ;
#30589=ADVANCED_FACE ( 'NONE', ( #19375 ), #67016, .T. ) ;
#30595=CYLINDRICAL_SURFACE ( 'NONE', #63325, 4.999999999999998224 ) ;
#30603=CARTESIAN_POINT ( 'NONE',  ( 14.44687500061451502, 0.000000000000000000, 4.756430356249998326 ) ) ;
#30606=CARTESIAN_POINT ( 'NONE',  ( 24.42187500061451289, -4.119189519843968306, 2.378215178124996054 ) ) ;
#30620=CARTESIAN_POINT ( 'NONE',  ( 24.49687500061451573, -2.746126346562646425, 4.756430356249996549 ) ) ;
#30623=DIRECTION ( 'NONE',  ( 0.000000000000000000, 0.000000000000000000, 1.000000000000000000 ) ) ;
#30638=CARTESIAN_POINT ( 'NONE',  ( 12.79687500061451821, -2.746126346562646425, 4.756430356249996549 ) ) ;
#30651=CARTESIAN_POINT ( 'NONE',  ( 23.30625000122903145, 0.000000000000000000, 4.999999999999998224 ) ) ;
#30667=CARTESIAN_POINT ( 'NONE',  ( 14.63437500061451679, -4.119189519843968306, 2.378215178124996054 ) ) ;
#30674=CARTESIAN_POINT ( 'NONE',  ( 14.84999999999999964, -4.330127018922190985, -2.500000000000001332 ) ) ;
#30678=CARTESIAN_POINT ( 'NONE',  ( 23.89687500061451431, 0.000000000000000000, 4.756430356249998326 ) ) ;
#30682=EDGE_CURVE ( 'NONE', #14158, #31771, #52305, .T. ) ;
#30687=CARTESIAN_POINT ( 'NONE',  ( 21.45937500061451075, 2.746126346562645981, -4.756430356249997438 ) ) ;
#30689=CARTESIAN_POINT ( 'NONE',  ( 9.496875000614517504, 0.000000000000000000, 4.756430356249998326 ) ) ;
#30697=VERTEX_POINT ( 'NONE', #71803 ) ;
#30699=CARTESIAN_POINT ( 'NONE',  ( 8.446875000614515017, 4.119189519843966529, -2.378215178124998275 ) ) ;
#30722=CARTESIAN_POINT ( 'NONE',  ( 19.95937500061451786, 0.000000000000000000, 4.756430356249998326 ) ) ;
#30757=CARTESIAN_POINT ( 'NONE',  ( 21.12187500061451573, 2.746126346562645981, -4.756430356249997438 ) ) ;
#30763=CARTESIAN_POINT ( 'NONE',  ( 21.60000000000000142, -4.330127018922190985, -2.500000000000001332 ) ) ;
#30767=DIRECTION ( 'NONE',  ( -1.000000000000000000, -0.000000000000000000, -0.000000000000000000 ) ) ;
#30775=CARTESIAN_POINT ( 'NONE',  ( 29.63437500061451857, 5.492252693125287522, 3.363034840372157021E-16 ) ) ;
#30777=CARTESIAN_POINT ( 'NONE',  ( 15.34687500061451537, 0.000000000000000000, 4.756430356249998326 ) ) ;
#30789=CARTESIAN_POINT ( 'NONE',  ( 8.034375000614515372, 5.492252693125287522, 3.363034840372157021E-16 ) ) ;
#30792=VECTOR ( 'NONE', #13975, 1000.000000000000000 ) ;
#30800=CARTESIAN_POINT ( 'NONE',  ( 29.37187500061451573, -4.119189519843968306, 2.378215178124996054 ) ) ;
#30803=CARTESIAN_POINT ( 'NONE',  ( 8.324999999999999289, 4.330127018922191873, 2.499999999999999556 ) ) ;
#30810=CARTESIAN_POINT ( 'NONE',  ( 27.08437500061451786, 4.119189519843966529, 2.378215178124999607 ) ) ;
#30812=CARTESIAN_POINT ( 'NONE',  ( 9.346875000614517148, -2.746126346562642428, -4.756430356249999214 ) ) ;
#30829=CARTESIAN_POINT ( 'NONE',  ( 21.65625000122903288, -4.330127018922190985, -2.500000000000001332 ) ) ;
#30844=CARTESIAN_POINT ( 'NONE',  ( 27.79687500061451999, -2.746126346562642428, -4.756430356249999214 ) ) ;
#30852=CARTESIAN_POINT ( 'NONE',  ( 24.89999999999999858, 4.330127018922192761, -2.499999999999997780 ) ) ;
#30860=CARTESIAN_POINT ( 'NONE',  ( 17.84999999999999787, 0.000000000000000000, 4.999999999999998224 ) ) ;
#30868=FACE_OUTER_BOUND ( 'NONE', #4339, .T. ) ;
#30878=CARTESIAN_POINT ( 'NONE',  ( 16.95937500061451431, 2.746126346562645981, -4.756430356249997438 ) ) ;
#30887=ORIENTED_EDGE ( 'NONE', *, *, #69324, .T. ) ;
#30893=CARTESIAN_POINT ( 'NONE',  ( 16.38749999999999929, 5.773502691896255534, 3.535250795749688401E-16 ) ) ;
#30897=CARTESIAN_POINT ( 'NONE',  ( 18.64687500061451786, -2.746126346562646425, 4.756430356249996549 ) ) ;
#30900=( BOUNDED_CURVE ( )  B_SPLINE_CURVE ( 2, ( #55038, #65017, #71667, #19940, #21042, #65379, #37312 ),
 .UNSPECIFIED., .F., .F. ) 
 B_SPLINE_CURVE_WITH_KNOTS ( ( 3, 2, 2, 3 ),
 ( 0.7100000000000001865, 0.7133333333333334858, 0.7166666666666667851, 0.7199999999999999734 ),
 .UNSPECIFIED. ) 
 CURVE ( )  GEOMETRIC_REPRESENTATION_ITEM ( )  RATIONAL_B_SPLINE_CURVE ( ( 0.9999999999999911182, 0.8660254037844475894, 1.000000000000000000, 0.8660254037844387076, 1.000000000000000000, 0.8660254037844387076, 1.000000000000000000 ) ) 
 REPRESENTATION_ITEM ( '' )  );
#30907=EDGE_CURVE ( 'NONE', #32393, #6086, #59852, .T. ) ;
#30909=CARTESIAN_POINT ( 'NONE',  ( 45.00000000000000000, 0.000000000000000000, 0.000000000000000000 ) ) ;
#30912=FACE_OUTER_BOUND ( 'NONE', #52615, .T. ) ;
#30916=CARTESIAN_POINT ( 'NONE',  ( 27.20625000122903359, 4.330127018922192761, -2.499999999999997780 ) ) ;
#30919=CARTESIAN_POINT ( 'NONE',  ( 7.724999999999999645, 6.123233995736764310E-16, -4.999999999999998224 ) ) ;
#30940=CARTESIAN_POINT ( 'NONE',  ( 7.921875000614517326, -5.492252693125287522, -1.008910452111647106E-15 ) ) ;
#30953=DIRECTION ( 'NONE',  ( 0.000000000000000000, 0.000000000000000000, 1.000000000000000000 ) ) ;
#30955=CARTESIAN_POINT ( 'NONE',  ( 22.57499999999999929, 6.123233995736764310E-16, -4.999999999999998224 ) ) ;
#30964=CARTESIAN_POINT ( 'NONE',  ( 14.78437500061451537, 5.492252693125287522, 3.363034840372157021E-16 ) ) ;
#30967=CARTESIAN_POINT ( 'NONE',  ( 23.03437500061451360, -2.746126346562646425, 4.756430356249996549 ) ) ;
#30972=CARTESIAN_POINT ( 'NONE',  ( 24.00000000000000000, 4.330127018922192761, -2.499999999999997780 ) ) ;
#30977=CARTESIAN_POINT ( 'NONE',  ( 23.32499999999999929, -4.330127018922194537, 2.499999999999995559 ) ) ;
#30985=CARTESIAN_POINT ( 'NONE',  ( 23.78437500061451360, 5.824947211148865298E-16, -4.756430356249998326 ) ) ;
#30995=CARTESIAN_POINT ( 'NONE',  ( 25.21875000122903288, -5.773502691896255534, -1.060575238724906372E-15 ) ) ;
#31005=CARTESIAN_POINT ( 'NONE',  ( 12.60937500061451821, 4.119189519843966529, -2.378215178124998275 ) ) ;
#31031=CARTESIAN_POINT ( 'NONE',  ( 13.28437500061451715, -4.119189519843968306, 2.378215178124996054 ) ) ;
#31038=CARTESIAN_POINT ( 'NONE',  ( 16.01249999999999929, 2.886751345948126879, 4.999999999999999112 ) ) ;
#31041=CARTESIAN_POINT ( 'NONE',  ( 24.63749999999999929, -2.886751345948143310, 4.999999999999972466 ) ) ;
#31046=CARTESIAN_POINT ( 'NONE',  ( 26.62500000000000000, 6.123233995736764310E-16, -4.999999999999998224 ) ) ;
#31051=CARTESIAN_POINT ( 'NONE',  ( 22.99687500061451573, 0.000000000000000000, 4.756430356249998326 ) ) ;
#31053=CARTESIAN_POINT ( 'NONE',  ( 8.109375000614518214, 2.746126346562643317, 4.756430356249998326 ) ) ;
#31061=CARTESIAN_POINT ( 'NONE',  ( 8.793750001229033941, 5.773502691896255534, 3.535250795749688401E-16 ) ) ;
#31064=CARTESIAN_POINT ( 'NONE',  ( 8.896875000614517859, 4.119189519843966529, -2.378215178124998275 ) ) ;
#31071=CARTESIAN_POINT ( 'NONE',  ( 7.556250001229035007, 0.000000000000000000, 4.999999999999998224 ) ) ;
#31075=EDGE_LOOP ( 'NONE', ( #19978, #67792, #22346, #25762 ) ) ;
#31083=CARTESIAN_POINT ( 'NONE',  ( 22.87500000000000000, -4.330127018922194537, 2.499999999999995559 ) ) ;
#31087=CARTESIAN_POINT ( 'NONE',  ( 18.64687500061451786, -2.746126346562646425, 4.756430356249996549 ) ) ;
#31121=CARTESIAN_POINT ( 'NONE',  ( 20.97187500061451715, -5.492252693125287522, -1.008910452111647106E-15 ) ) ;
#31127=CARTESIAN_POINT ( 'NONE',  ( 22.16250000000000142, 2.886751345948129099, -4.999999999999998224 ) ) ;
#31131=LINE ( 'NONE', #47761, #38295 ) ;
#31132=CARTESIAN_POINT ( 'NONE',  ( 11.90625000122903465, 4.330127018922192761, -2.499999999999997780 ) ) ;
#31137=CARTESIAN_POINT ( 'NONE',  ( 7.968750001229034652, 2.886751345948126879, 4.999999999999999112 ) ) ;
#31139=CARTESIAN_POINT ( 'NONE',  ( 16.77187500061451431, -4.119189519843968306, 2.378215178124996054 ) ) ;
#31150=CARTESIAN_POINT ( 'NONE',  ( 7.734375000614518214, -2.746126346562646425, 4.756430356249996549 ) ) ;
#31155=ORIENTED_EDGE ( 'NONE', *, *, #18371, .T. ) ;
#31161=CARTESIAN_POINT ( 'NONE',  ( 28.09687500061451715, -4.119189519843965641, -2.378215178125001383 ) ) ;
#31162=ORIENTED_EDGE ( 'NONE', *, *, #62210, .F. ) ;
#31165=CARTESIAN_POINT ( 'NONE',  ( 8.962500000000002132, -5.773502691896255534, -1.060575238724906372E-15 ) ) ;
#31172=CARTESIAN_POINT ( 'NONE',  ( 26.82187500061451857, -5.492252693125287522, -1.008910452111647106E-15 ) ) ;
#31174=CARTESIAN_POINT ( 'NONE',  ( 9.909375000614517148, 4.119189519843966529, -2.378215178124998275 ) ) ;
#31194=CARTESIAN_POINT ( 'NONE',  ( 20.15625000122903288, 0.000000000000000000, 4.999999999999998224 ) ) ;
#31207=( BOUNDED_CURVE ( )  B_SPLINE_CURVE ( 2, ( #45129, #11141, #38494, #10417, #32948, #55125, #33670 ),
 .UNSPECIFIED., .F., .F. ) 
 B_SPLINE_CURVE_WITH_KNOTS ( ( 3, 2, 2, 3 ),
 ( 0.6900000000000000577, 0.6933333333333334680, 0.6966666666666668783, 0.7000000000000001776 ),
 .UNSPECIFIED. ) 
 CURVE ( )  GEOMETRIC_REPRESENTATION_ITEM ( )  RATIONAL_B_SPLINE_CURVE ( ( 0.9999999999999955591, 0.8660254037844431485, 1.000000000000000000, 0.8660254037844387076, 1.000000000000000000, 0.8660254037844298258, 1.000000000000008882 ) ) 
 REPRESENTATION_ITEM ( '' )  );
#31210=CARTESIAN_POINT ( 'NONE',  ( 27.72187500061451715, -5.492252693125287522, -1.008910452111647106E-15 ) ) ;
#31228=CARTESIAN_POINT ( 'NONE',  ( 16.44375000122903074, 5.773502691896255534, 3.535250795749688401E-16 ) ) ;
#31233=FACE_OUTER_BOUND ( 'NONE', #21159, .T. ) ;
#31240=EDGE_LOOP ( 'NONE', ( #25487, #34140, #7533, #60770 ) ) ;
#31243=VERTEX_POINT ( 'NONE', #44721 ) ;
#31247=CARTESIAN_POINT ( 'NONE',  ( 17.18437500061451573, -2.746126346562646425, 4.756430356249996549 ) ) ;
#31267=CARTESIAN_POINT ( 'NONE',  ( 16.43437500061451573, -4.119189519843968306, 2.378215178124996054 ) ) ;
#31278=ORIENTED_EDGE ( 'NONE', *, *, #34726, .T. ) ;
#31286=CARTESIAN_POINT ( 'NONE',  ( 28.25625000122903074, 0.000000000000000000, 4.999999999999998224 ) ) ;
#31302=CARTESIAN_POINT ( 'NONE',  ( 20.77500000000000213, 6.123233995736764310E-16, -4.999999999999998224 ) ) ;
#31313=CARTESIAN_POINT ( 'NONE',  ( 28.31250000000000000, -5.773502691896255534, -1.060575238724906372E-15 ) ) ;
#31318=EDGE_CURVE ( 'NONE', #64487, #53529, #28797, .T. ) ;
#31323=VECTOR ( 'NONE', #6854, 1000.000000000000000 ) ;
#31328=AXIS2_PLACEMENT_3D ( 'NONE', #24071, #12628, #52157 ) ;
#31333=CARTESIAN_POINT ( 'NONE',  ( 15.53437500061451360, -2.746126346562642428, -4.756430356249999214 ) ) ;
#31334=ORIENTED_EDGE ( 'NONE', *, *, #3173, .T. ) ;
#31337=CARTESIAN_POINT ( 'NONE',  ( 24.19687500061451502, 4.119189519843966529, -2.378215178124998275 ) ) ;
#31342=CARTESIAN_POINT ( 'NONE',  ( 16.03125000122903288, 4.330127018922191873, 2.499999999999999556 ) ) ;
#31348=CARTESIAN_POINT ( 'NONE',  ( 12.93750000000000178, -2.886751345948129988, 4.999999999999997335 ) ) ;
#31355=CARTESIAN_POINT ( 'NONE',  ( 24.57187500061451502, -5.492252693125287522, -1.008910452111647106E-15 ) ) ;
#31358=CARTESIAN_POINT ( 'NONE',  ( 45.00000000000000000, 6.123233995736764310E-16, -4.999999999999998224 ) ) ;
#31375=CARTESIAN_POINT ( 'NONE',  ( 12.12187500061451573, 2.746126346562645981, -4.756430356249997438 ) ) ;
#31404=CARTESIAN_POINT ( 'NONE',  ( 13.02187500061451608, 2.746126346562645981, -4.756430356249997438 ) ) ;
#31413=CARTESIAN_POINT ( 'NONE',  ( 15.41250000000000142, 2.886751345948129099, -4.999999999999998224 ) ) ;
#31421=CARTESIAN_POINT ( 'NONE',  ( 26.51249999999999929, -5.773502691896255534, -1.060575238724906372E-15 ) ) ;
#31425=CARTESIAN_POINT ( 'NONE',  ( 21.94687500061451146, 4.119189519843966529, -2.378215178124998275 ) ) ;
#31427=CARTESIAN_POINT ( 'NONE',  ( 7.996875000614515727, 4.119189519843966529, -2.378215178124998275 ) ) ;
#31438=CARTESIAN_POINT ( 'NONE',  ( 9.121875000614517504, -4.119189519843968306, 2.378215178124996054 ) ) ;
#31457=CARTESIAN_POINT ( 'NONE',  ( 14.26875000122903181, 2.886751345948182834, 4.999999999999902300 ) ) ;
#31460=CARTESIAN_POINT ( 'NONE',  ( 19.43437500061451928, 4.119189519843966529, 2.378215178124999607 ) ) ;
#31479=ADVANCED_FACE ( 'NONE', ( #61685 ), #5905, .T. ) ;
#31496=CARTESIAN_POINT ( 'NONE',  ( 20.14687500061451786, -2.746126346562642428, -4.756430356249999214 ) ) ;
#31502=CARTESIAN_POINT ( 'NONE',  ( 21.37499999999999645, 4.330127018922191873, 2.499999999999999556 ) ) ;
#31509=DIRECTION ( 'NONE',  ( -1.000000000000000000, -0.000000000000000000, -0.000000000000000000 ) ) ;
#31513=CARTESIAN_POINT ( 'NONE',  ( 29.67187500061451644, 4.119189519843966529, 2.378215178124999607 ) ) ;
#31515=CARTESIAN_POINT ( 'NONE',  ( 15.42187500061451466, -4.119189519843968306, 2.378215178124996054 ) ) ;
#31518=VERTEX_POINT ( 'NONE', #67256 ) ;
#31521=CARTESIAN_POINT ( 'NONE',  ( 17.04375000122903572, -2.886751345948130876, 4.999999999999996447 ) ) ;
#31523=VECTOR ( 'NONE', #23553, 1000.000000000000000 ) ;
#31525=CARTESIAN_POINT ( 'NONE',  ( 8.859375000614514661, 2.746126346562645981, -4.756430356249997438 ) ) ;
#31536=CARTESIAN_POINT ( 'NONE',  ( 27.60937500061451644, -5.492252693125287522, -1.008910452111647106E-15 ) ) ;
#31540=CARTESIAN_POINT ( 'NONE',  ( 25.74375000122903856, -2.886751345948098013, -5.000000000000047073 ) ) ;
#31547=CARTESIAN_POINT ( 'NONE',  ( 27.49687500061451573, 5.492252693125287522, 3.363034840372157021E-16 ) ) ;
#31549=CARTESIAN_POINT ( 'NONE',  ( 9.234375000614518214, -4.119189519843968306, 2.378215178124996054 ) ) ;
#31559=CARTESIAN_POINT ( 'NONE',  ( 45.00000000000000000, 6.123233995736764310E-16, -4.999999999999998224 ) ) ;
#31566=CARTESIAN_POINT ( 'NONE',  ( 21.28125000122903288, 6.123233995736764310E-16, -4.999999999999998224 ) ) ;
#31576=EDGE_CURVE ( 'NONE', #12847, #58973, #19722, .T. ) ;
#31582=CARTESIAN_POINT ( 'NONE',  ( 27.27187500061451431, -5.492252693125287522, -1.008910452111647106E-15 ) ) ;
#31591=CARTESIAN_POINT ( 'NONE',  ( 22.06875000122903074, -5.773502691896255534, -1.060575238724906372E-15 ) ) ;
#31611=ADVANCED_FACE ( 'NONE', ( #371 ), #39902, .T. ) ;
#31615=ORIENTED_EDGE ( 'NONE', *, *, #26754, .T. ) ;
#31620=CARTESIAN_POINT ( 'NONE',  ( 11.58750000000000036, -2.886751345948074920, 5.000000000000092371 ) ) ;
#31623=CARTESIAN_POINT ( 'NONE',  ( 17.37187500061451573, 5.824947211148865298E-16, -4.756430356249998326 ) ) ;
#31635=VECTOR ( 'NONE', #39156, 1000.000000000000000 ) ;
#31638=CARTESIAN_POINT ( 'NONE',  ( 25.78125000122903288, 6.123233995736764310E-16, -4.999999999999998224 ) ) ;
#31642=CARTESIAN_POINT ( 'NONE',  ( 27.05625000122903145, -4.330127018922190985, -2.500000000000001332 ) ) ;
#31643=CARTESIAN_POINT ( 'NONE',  ( 17.18437500061451573, 4.119189519843966529, 2.378215178124999607 ) ) ;
#31653=CYLINDRICAL_SURFACE ( 'NONE', #52523, 4.999999999999998224 ) ;
#31659=CARTESIAN_POINT ( 'NONE',  ( 28.81875000122903074, -5.773502691896255534, -1.060575238724906372E-15 ) ) ;
#31661=CARTESIAN_POINT ( 'NONE',  ( 29.92968750030725644, 0.000000000000000000, 4.878215178124998275 ) ) ;
#31673=CARTESIAN_POINT ( 'NONE',  ( 16.50000000000000000, 0.000000000000000000, 4.999999999999998224 ) ) ;
#31684=CARTESIAN_POINT ( 'NONE',  ( 7.659375000614518036, 4.119189519843966529, -2.378215178124998275 ) ) ;
#31693=CARTESIAN_POINT ( 'NONE',  ( 27.58125000122903359, 6.123233995736764310E-16, -4.999999999999998224 ) ) ;
#31701=CARTESIAN_POINT ( 'NONE',  ( 15.04687500061451466, -4.119189519843965641, -2.378215178125001383 ) ) ;
#31702=VERTEX_POINT ( 'NONE', #13979 ) ;
#31705=CARTESIAN_POINT ( 'NONE',  ( 22.95937500061451786, 2.746126346562643317, 4.756430356249998326 ) ) ;
#31715=CARTESIAN_POINT ( 'NONE',  ( 12.44999999999999929, 0.000000000000000000, 4.999999999999998224 ) ) ;
#31722=CARTESIAN_POINT ( 'NONE',  ( 25.80937500061451928, 0.000000000000000000, 4.756430356249998326 ) ) ;
#31743=CARTESIAN_POINT ( 'NONE',  ( 8.784375000614518925, -4.119189519843968306, 2.378215178124996054 ) ) ;
#31744=ADVANCED_FACE ( 'NONE', ( #46520 ), #8442, .T. ) ;
#31771=VERTEX_POINT ( 'NONE', #25061 ) ;
#31774=CARTESIAN_POINT ( 'NONE',  ( 14.03437500061451715, 4.119189519843966529, 2.378215178124999607 ) ) ;
#31781=CARTESIAN_POINT ( 'NONE',  ( 15.59999999999999964, 0.000000000000000000, 4.999999999999998224 ) ) ;
#31784=DIRECTION ( 'NONE',  ( 0.000000000000000000, 0.000000000000000000, 1.000000000000000000 ) ) ;
#31793=CARTESIAN_POINT ( 'NONE',  ( 23.40937500061451715, 2.746126346562643317, 4.756430356249998326 ) ) ;
#31806=CARTESIAN_POINT ( 'NONE',  ( 9.421875000614514661, 4.119189519843966529, 2.378215178124999607 ) ) ;
#31828=CARTESIAN_POINT ( 'NONE',  ( 16.13437500061451502, 5.824947211148865298E-16, -4.756430356249998326 ) ) ;
#31842=ORIENTED_EDGE ( 'NONE', *, *, #5278, .T. ) ;
#31861=CARTESIAN_POINT ( 'NONE',  ( 21.90937500061451715, -4.119189519843965641, -2.378215178125001383 ) ) ;
#31867=CARTESIAN_POINT ( 'NONE',  ( 21.07499999999999929, -4.330127018922194537, 2.499999999999995559 ) ) ;
#31874=DIRECTION ( 'NONE',  ( -1.000000000000000000, -0.000000000000000000, -0.000000000000000000 ) ) ;
#31879=CARTESIAN_POINT ( 'NONE',  ( 29.52187500061451431, 5.824947211148865298E-16, -4.756430356249998326 ) ) ;
#31881=CARTESIAN_POINT ( 'NONE',  ( 15.15937500061451892, 2.746126346562645981, -4.756430356249997438 ) ) ;
#31884=EDGE_LOOP ( 'NONE', ( #23785, #71661, #15987, #7470 ) ) ;
#31891=CARTESIAN_POINT ( 'NONE',  ( 7.921875000614517326, 5.824947211148865298E-16, -4.756430356249998326 ) ) ;
#31892=VERTEX_POINT ( 'NONE', #2185 ) ;
#31901=CARTESIAN_POINT ( 'NONE',  ( 16.10625000122903216, 0.000000000000000000, 4.999999999999998224 ) ) ;
#31902=EDGE_LOOP ( 'NONE', ( #3214, #35834, #7435, #16992 ) ) ;
#31913=CARTESIAN_POINT ( 'NONE',  ( 25.88437500061451502, -4.119189519843968306, 2.378215178124996054 ) ) ;
#31915=CARTESIAN_POINT ( 'NONE',  ( 7.621875000614519280, 2.746126346562645981, -4.756430356249997438 ) ) ;
#31931=CARTESIAN_POINT ( 'NONE',  ( 18.16875000122903216, 2.886751345948129099, -4.999999999999998224 ) ) ;
#31947=CARTESIAN_POINT ( 'NONE',  ( 28.62187500061451573, -5.492252693125287522, -1.008910452111647106E-15 ) ) ;
#31954=CARTESIAN_POINT ( 'NONE',  ( 10.25625000122903252, 0.000000000000000000, 4.999999999999998224 ) ) ;
#31968=CARTESIAN_POINT ( 'NONE',  ( 45.00000000000000000, 0.000000000000000000, 0.000000000000000000 ) ) ;
#31975=ORIENTED_EDGE ( 'NONE', *, *, #50679, .F. ) ;
#31978=EDGE_CURVE ( 'NONE', #53311, #7820, #3026, .T. ) ;
#31980=VERTEX_POINT ( 'NONE', #68698 ) ;
#31984=CARTESIAN_POINT ( 'NONE',  ( 13.84687500061451715, 4.119189519843966529, -2.378215178124998275 ) ) ;
#31992=EDGE_LOOP ( 'NONE', ( #17725, #55241, #61873, #24191 ) ) ;
#31998=CARTESIAN_POINT ( 'NONE',  ( 16.42500000000000071, 4.330127018922191873, 2.499999999999999556 ) ) ;
#32002=CARTESIAN_POINT ( 'NONE',  ( 45.00000000000000000, 6.123233995736764310E-16, -4.999999999999998224 ) ) ;
#32003=CARTESIAN_POINT ( 'NONE',  ( 14.93437500061451750, 4.119189519843966529, 2.378215178124999607 ) ) ;
#32013=CARTESIAN_POINT ( 'NONE',  ( 13.08750000000000213, -2.886751345948126435, -5.000000000000000000 ) ) ;
#32019=CARTESIAN_POINT ( 'NONE',  ( 28.96875000122903288, 2.886751345948129099, -4.999999999999998224 ) ) ;
#32021=DIRECTION ( 'NONE',  ( 0.000000000000000000, 0.000000000000000000, 1.000000000000000000 ) ) ;
#32030=ORIENTED_EDGE ( 'NONE', *, *, #54265, .F. ) ;
#32043=( BOUNDED_CURVE ( )  B_SPLINE_CURVE ( 2, ( #33790, #11629, #5723, #62943, #57400, #192, #34145 ),
 .UNSPECIFIED., .F., .F. ) 
 B_SPLINE_CURVE_WITH_KNOTS ( ( 3, 2, 2, 3 ),
 ( 0.8300000000000000711, 0.8333333333333334814, 0.8366666666666666696, 0.8399999999999999689 ),
 .UNSPECIFIED. ) 
 CURVE ( )  GEOMETRIC_REPRESENTATION_ITEM ( )  RATIONAL_B_SPLINE_CURVE ( ( 0.9999999999999955591, 0.8660254037844431485, 1.000000000000000000, 0.8660254037844387076, 1.000000000000000000, 0.8660254037844387076, 1.000000000000000000 ) ) 
 REPRESENTATION_ITEM ( '' )  );
#32047=CARTESIAN_POINT ( 'NONE',  ( 26.21249999999999858, 2.886751345948129099, -4.999999999999998224 ) ) ;
#32070=CARTESIAN_POINT ( 'NONE',  ( 21.49687500061451573, 4.119189519843966529, -2.378215178124998275 ) ) ;
#32079=CARTESIAN_POINT ( 'NONE',  ( 13.23750000000000071, 5.773502691896255534, 3.535250795749688894E-16 ) ) ;
#32086=CARTESIAN_POINT ( 'NONE',  ( 25.95937500061451431, -4.119189519843965641, -2.378215178125001383 ) ) ;
#32089=CARTESIAN_POINT ( 'NONE',  ( 13.40625000122903288, 0.000000000000000000, 4.999999999999998224 ) ) ;
#32106=CARTESIAN_POINT ( 'NONE',  ( 9.684375000614517504, -4.119189519843968306, 2.378215178124996054 ) ) ;
#32117=ORIENTED_EDGE ( 'NONE', *, *, #28533, .T. ) ;
#32118=ORIENTED_EDGE ( 'NONE', *, *, #65260, .T. ) ;
#32133=CARTESIAN_POINT ( 'NONE',  ( 12.19687500061451679, 5.492252693125287522, 3.363034840372157021E-16 ) ) ;
#32155=CARTESIAN_POINT ( 'NONE',  ( 20.03437500061451715, -2.746126346562642428, -4.756430356249999214 ) ) ;
#32169=CARTESIAN_POINT ( 'NONE',  ( 10.08749999999999858, 5.773502691896255534, 3.535250795749688401E-16 ) ) ;
#32171=CARTESIAN_POINT ( 'NONE',  ( 9.234375000614514661, -2.746126346562642428, -4.756430356249999214 ) ) ;
#32180=CARTESIAN_POINT ( 'NONE',  ( 14.96250000000000036, 2.886751345948129099, -4.999999999999997335 ) ) ;
#32194=CARTESIAN_POINT ( 'NONE',  ( 17.59687500061451715, 5.492252693125287522, 3.363034840372157021E-16 ) ) ;
#32221=ORIENTED_EDGE ( 'NONE', *, *, #39155, .T. ) ;
#32224=CARTESIAN_POINT ( 'NONE',  ( 20.67187500061451289, 2.746126346562645981, -4.756430356249997438 ) ) ;
#32230=CARTESIAN_POINT ( 'NONE',  ( 23.32499999999999929, -4.330127018922194537, 2.499999999999995559 ) ) ;
#32232=CARTESIAN_POINT ( 'NONE',  ( 20.73750000000000071, -2.886751345948098013, -5.000000000000047073 ) ) ;
#32233=CARTESIAN_POINT ( 'NONE',  ( 45.00000000000000000, 0.000000000000000000, 0.000000000000000000 ) ) ;
#32241=CARTESIAN_POINT ( 'NONE',  ( 26.78437500061451715, -2.746126346562642428, -4.756430356249999214 ) ) ;
#32243=CARTESIAN_POINT ( 'NONE',  ( 14.25937500061451857, 2.746126346562645981, -4.756430356249997438 ) ) ;
#32253=CARTESIAN_POINT ( 'NONE',  ( 7.846875000614515372, -4.119189519843965641, -2.378215178125001383 ) ) ;
#32259=ORIENTED_EDGE ( 'NONE', *, *, #59745, .T. ) ;
#32270=CARTESIAN_POINT ( 'NONE',  ( 45.00000000000000000, 0.000000000000000000, 0.000000000000000000 ) ) ;
#32276=CARTESIAN_POINT ( 'NONE',  ( 23.52187500061451786, 2.746126346562643317, 4.756430356249998326 ) ) ;
#32278=FACE_OUTER_BOUND ( 'NONE', #20044, .T. ) ;
#32287=CARTESIAN_POINT ( 'NONE',  ( 17.41875000122903216, 2.886751345948182834, 4.999999999999902300 ) ) ;
#32295=CARTESIAN_POINT ( 'NONE',  ( 18.01875000122903359, -5.773502691896255534, -1.060575238724906372E-15 ) ) ;
#32297=CARTESIAN_POINT ( 'NONE',  ( 45.00000000000000000, 0.000000000000000000, 0.000000000000000000 ) ) ;
#32311=CARTESIAN_POINT ( 'NONE',  ( 27.64687500061452141, -2.746126346562646425, 4.756430356249996549 ) ) ;
#32328=CARTESIAN_POINT ( 'NONE',  ( 21.04687500061451644, 4.119189519843966529, -2.378215178124998275 ) ) ;
#32331=ORIENTED_EDGE ( 'NONE', *, *, #45231, .F. ) ;
#32332=CARTESIAN_POINT ( 'NONE',  ( 23.47499999999999787, 6.123233995736764310E-16, -4.999999999999998224 ) ) ;
#32343=CARTESIAN_POINT ( 'NONE',  ( 18.97499999999999787, 6.123233995736764310E-16, -4.999999999999998224 ) ) ;
#32346=CARTESIAN_POINT ( 'NONE',  ( 14.78437500061451537, 5.492252693125287522, 3.363034840372157021E-16 ) ) ;
#32364=CARTESIAN_POINT ( 'NONE',  ( 15.98437500061451821, -4.119189519843968306, 2.378215178124996054 ) ) ;
#32377=CARTESIAN_POINT ( 'NONE',  ( 25.68750000000000000, -2.886751345948167735, -4.999999999999927169 ) ) ;
#32381=CARTESIAN_POINT ( 'NONE',  ( 26.38125000122903430, 4.330127018922191873, 2.499999999999999556 ) ) ;
#32385=DIRECTION ( 'NONE',  ( -1.000000000000000000, -0.000000000000000000, -0.000000000000000000 ) ) ;
#32393=VERTEX_POINT ( 'NONE', #46057 ) ;
#32395=DIRECTION ( 'NONE',  ( -1.000000000000000000, -0.000000000000000000, -0.000000000000000000 ) ) ;
#32412=CARTESIAN_POINT ( 'NONE',  ( 45.00000000000000000, 0.000000000000000000, 0.000000000000000000 ) ) ;
#32421=CARTESIAN_POINT ( 'NONE',  ( 27.35625000122903216, 0.000000000000000000, 4.999999999999998224 ) ) ;
#32433=CARTESIAN_POINT ( 'NONE',  ( 21.19687500061451502, 0.000000000000000000, 4.756430356249998326 ) ) ;
#32437=VECTOR ( 'NONE', #59983, 1000.000000000000000 ) ;
#32444=CARTESIAN_POINT ( 'NONE',  ( 12.26249999999999929, 2.886751345948129099, -4.999999999999998224 ) ) ;
#32452=CARTESIAN_POINT ( 'NONE',  ( 21.98437500061451644, 5.824947211148865298E-16, -4.756430356249998326 ) ) ;
#32466=VECTOR ( 'NONE', #54505, 1000.000000000000000 ) ;
#32476=CARTESIAN_POINT ( 'NONE',  ( 10.80937500061451928, 4.119189519843966529, -2.378215178124998275 ) ) ;
#32480=( BOUNDED_CURVE ( )  B_SPLINE_CURVE ( 2, ( #50154, #16514, #23147, #51602, #44253, #67154, #22066 ),
 .UNSPECIFIED., .F., .F. ) 
 B_SPLINE_CURVE_WITH_KNOTS ( ( 3, 2, 2, 3 ),
 ( 0.01999999999999995878, 0.02333333333333328583, 0.02666666666666661634, 0.02999999999999993991 ),
 .UNSPECIFIED. ) 
 CURVE ( )  GEOMETRIC_REPRESENTATION_ITEM ( )  RATIONAL_B_SPLINE_CURVE ( ( 1.000000000000001554, 0.8660254037844370423, 1.000000000000000000, 0.8660254037844387076, 1.000000000000000000, 0.8660254037844410391, 0.9999999999999976685 ) ) 
 REPRESENTATION_ITEM ( '' )  );
#32485=ORIENTED_EDGE ( 'NONE', *, *, #14319, .F. ) ;
#32494=EDGE_CURVE ( 'NONE', #60311, #24417, #2084, .T. ) ;
#32501=CARTESIAN_POINT ( 'NONE',  ( 12.57187500061451857, 2.746126346562645981, -4.756430356249997438 ) ) ;
#32510=VECTOR ( 'NONE', #43348, 1000.000000000000000 ) ;
#32520=CARTESIAN_POINT ( 'NONE',  ( 19.32187500061451857, 4.119189519843966529, 2.378215178124999607 ) ) ;
#32523=CARTESIAN_POINT ( 'NONE',  ( 14.41875000122903394, -5.773502691896255534, -1.060575238724906372E-15 ) ) ;
#32537=CARTESIAN_POINT ( 'NONE',  ( 29.70937500061451431, 4.119189519843966529, -2.378215178124998275 ) ) ;
#32546=VECTOR ( 'NONE', #27493, 1000.000000000000227 ) ;
#32547=ORIENTED_EDGE ( 'NONE', *, *, #11487, .F. ) ;
#32559=CARTESIAN_POINT ( 'NONE',  ( 18.04687500061451999, 5.492252693125287522, 3.363034840372157021E-16 ) ) ;
#32563=VERTEX_POINT ( 'NONE', #35680 ) ;
#32588=ADVANCED_FACE ( 'NONE', ( #30868 ), #59293, .T. ) ;
#32592=CARTESIAN_POINT ( 'NONE',  ( 19.09687500061451360, -2.746126346562646425, 4.756430356249996549 ) ) ;
#32598=CARTESIAN_POINT ( 'NONE',  ( 20.81250000000000000, 2.886751345948129099, -4.999999999999998224 ) ) ;
#32600=LINE ( 'NONE', #60288, #11157 ) ;
#32608=CARTESIAN_POINT ( 'NONE',  ( 27.19687500061451502, -4.119189519843965641, -2.378215178125001383 ) ) ;
#32610=CARTESIAN_POINT ( 'NONE',  ( 12.90937500061451537, 2.746126346562645981, -4.756430356249997438 ) ) ;
#32613=VERTEX_POINT ( 'NONE', #2433 ) ;
#32616=DIRECTION ( 'NONE',  ( 0.000000000000000000, 0.000000000000000000, 1.000000000000000000 ) ) ;
#32626=ORIENTED_EDGE ( 'NONE', *, *, #70340, .T. ) ;
#32627=DIRECTION ( 'NONE',  ( -1.000000000000000000, -0.000000000000000000, -0.000000000000000000 ) ) ;
#32642=CARTESIAN_POINT ( 'NONE',  ( 25.28437500061451715, 4.119189519843966529, 2.378215178124999607 ) ) ;
#32644=CARTESIAN_POINT ( 'NONE',  ( 8.071875000614518569, 2.746126346562645981, -4.756430356249997438 ) ) ;
#32649=ORIENTED_EDGE ( 'NONE', *, *, #22474, .T. ) ;
#32663=CARTESIAN_POINT ( 'NONE',  ( 18.35625000122903216, 0.000000000000000000, 4.999999999999998224 ) ) ;
#32665=CARTESIAN_POINT ( 'NONE',  ( 21.43125000122903145, 4.330127018922191873, 2.499999999999999556 ) ) ;
#32675=EDGE_CURVE ( 'NONE', #38481, #55366, #7006, .T. ) ;
#32680=CARTESIAN_POINT ( 'NONE',  ( 27.00937500061451857, 4.119189519843966529, -2.378215178124998275 ) ) ;
#32685=EDGE_CURVE ( 'NONE', #52965, #40553, #14239, .T. ) ;
#32697=CARTESIAN_POINT ( 'NONE',  ( 10.93125000122903501, 6.123233995736764310E-16, -4.999999999999998224 ) ) ;
#32701=CARTESIAN_POINT ( 'NONE',  ( 20.07187500061451502, 5.824947211148865298E-16, -4.756430356249998326 ) ) ;
#32712=ORIENTED_EDGE ( 'NONE', *, *, #31576, .F. ) ;
#32716=CARTESIAN_POINT ( 'NONE',  ( 21.28125000122903288, 6.123233995736764310E-16, -4.999999999999998224 ) ) ;
#32718=CARTESIAN_POINT ( 'NONE',  ( 10.87500000000000000, 6.123233995736764310E-16, -4.999999999999998224 ) ) ;
#32719=CARTESIAN_POINT ( 'NONE',  ( 13.32187500061451502, 5.824947211148865298E-16, -4.756430356249998326 ) ) ;
#32722=DIRECTION ( 'NONE',  ( 0.000000000000000000, 0.000000000000000000, 1.000000000000000000 ) ) ;
#32728=CARTESIAN_POINT ( 'NONE',  ( 16.89375000122903359, 5.773502691896255534, 3.535250795749688401E-16 ) ) ;
#32735=CARTESIAN_POINT ( 'NONE',  ( 29.44687500061451146, -4.119189519843965641, -2.378215178125001383 ) ) ;
#32736=CARTESIAN_POINT ( 'NONE',  ( 15.00937500061451679, 0.000000000000000000, 4.756430356249998326 ) ) ;
#32754=CARTESIAN_POINT ( 'NONE',  ( 26.71875000122903288, 2.886751345948129099, -4.999999999999998224 ) ) ;
#32766=CARTESIAN_POINT ( 'NONE',  ( 45.00000000000000000, 0.000000000000000000, 0.000000000000000000 ) ) ;
#32769=FACE_OUTER_BOUND ( 'NONE', #2269, .T. ) ;
#32782=CARTESIAN_POINT ( 'NONE',  ( 12.67499999999999893, 6.123233995736764310E-16, -4.999999999999998224 ) ) ;
#32786=CARTESIAN_POINT ( 'NONE',  ( 26.08125000122903003, -4.330127018922194537, 2.499999999999995559 ) ) ;
#32794=VERTEX_POINT ( 'NONE', #14603 ) ;
#32798=ORIENTED_EDGE ( 'NONE', *, *, #48942, .T. ) ;
#32801=CARTESIAN_POINT ( 'NONE',  ( 22.24687500061451573, -4.119189519843965641, -2.378215178125001383 ) ) ;
#32807=CARTESIAN_POINT ( 'NONE',  ( 26.73749999999999716, 5.773502691896255534, 3.535250795749688401E-16 ) ) ;
#32809=CARTESIAN_POINT ( 'NONE',  ( 13.35000000000000142, 0.000000000000000000, 4.999999999999998224 ) ) ;
#32816=CARTESIAN_POINT ( 'NONE',  ( 22.28437500061451715, -4.119189519843968306, 2.378215178124996054 ) ) ;
#32828=ORIENTED_EDGE ( 'NONE', *, *, #43413, .T. ) ;
#32832=CARTESIAN_POINT ( 'NONE',  ( 27.35625000122903216, 0.000000000000000000, 4.999999999999998224 ) ) ;
#32834=EDGE_CURVE ( 'NONE', #8302, #23570, #46782, .T. ) ;
#32839=CARTESIAN_POINT ( 'NONE',  ( 11.10937500061451644, -4.119189519843965641, -2.378215178125001383 ) ) ;
#32863=CARTESIAN_POINT ( 'NONE',  ( 12.08437500061451608, 5.824947211148865298E-16, -4.756430356249998326 ) ) ;
#32872=CARTESIAN_POINT ( 'NONE',  ( 16.94999999999999929, 0.000000000000000000, 4.999999999999998224 ) ) ;
#32876=CARTESIAN_POINT ( 'NONE',  ( 19.50000000000000000, 4.330127018922192761, -2.499999999999997780 ) ) ;
#32879=FACE_OUTER_BOUND ( 'NONE', #10039, .T. ) ;
#32881=CARTESIAN_POINT ( 'NONE',  ( 20.59687500061451715, 4.119189519843966529, -2.378215178124998275 ) ) ;
#32884=CARTESIAN_POINT ( 'NONE',  ( 13.25625000122903074, 4.330127018922192761, -2.499999999999997780 ) ) ;
#32891=CARTESIAN_POINT ( 'NONE',  ( 21.71249999999999858, 2.886751345948129099, -4.999999999999997335 ) ) ;
#32899=CARTESIAN_POINT ( 'NONE',  ( 28.43437500061451573, 4.119189519843966529, 2.378215178124999607 ) ) ;
#32908=FACE_OUTER_BOUND ( 'NONE', #5989, .T. ) ;
#32922=CARTESIAN_POINT ( 'NONE',  ( 16.95937500061451786, -4.119189519843965641, -2.378215178125001383 ) ) ;
#32948=CARTESIAN_POINT ( 'NONE',  ( 14.32500000000000107, -4.330127018922194537, 2.499999999999995559 ) ) ;
#32953=CARTESIAN_POINT ( 'NONE',  ( 19.24687500061452283, -2.746126346562642428, -4.756430356249999214 ) ) ;
#32960=CARTESIAN_POINT ( 'NONE',  ( 20.62499999999999645, -4.330127018922194537, 2.499999999999995559 ) ) ;
#32965=CARTESIAN_POINT ( 'NONE',  ( 17.58749999999999858, -2.886751345948070480, -5.000000000000095923 ) ) ;
#32969=CARTESIAN_POINT ( 'NONE',  ( 27.53437500061451715, -2.746126346562646425, 4.756430356249996549 ) ) ;
#32971=CARTESIAN_POINT ( 'NONE',  ( 12.60937500061451289, 2.746126346562643317, 4.756430356249998326 ) ) ;
#32977=CARTESIAN_POINT ( 'NONE',  ( 17.23125000122903572, 6.123233995736764310E-16, -4.999999999999998224 ) ) ;
#32980=CARTESIAN_POINT ( 'NONE',  ( 45.00000000000000000, 0.000000000000000000, 0.000000000000000000 ) ) ;
#32981=CARTESIAN_POINT ( 'NONE',  ( 18.56250000000000000, 2.886751345948129099, -4.999999999999997335 ) ) ;
#33004=CARTESIAN_POINT ( 'NONE',  ( 24.53437500061451715, -4.119189519843968306, 2.378215178124996054 ) ) ;
#33006=CARTESIAN_POINT ( 'NONE',  ( 8.259375000614518569, 0.000000000000000000, 4.756430356249998326 ) ) ;
#33011=ORIENTED_EDGE ( 'NONE', *, *, #32685, .F. ) ;
#33016=CYLINDRICAL_SURFACE ( 'NONE', #17135, 4.999999999999998224 ) ;
#33024=CARTESIAN_POINT ( 'NONE',  ( 19.81875000122903430, -5.773502691896255534, -1.060575238724906372E-15 ) ) ;
#33040=CARTESIAN_POINT ( 'NONE',  ( 26.37187500061451217, -5.492252693125287522, -1.008910452111647106E-15 ) ) ;
#33054=CARTESIAN_POINT ( 'NONE',  ( 11.15625000122903288, 0.000000000000000000, 4.999999999999998224 ) ) ;
#33056=CARTESIAN_POINT ( 'NONE',  ( 14.08125000122903181, 6.123233995736764310E-16, -4.999999999999998224 ) ) ;
#33058=CARTESIAN_POINT ( 'NONE',  ( 19.77187500061451786, 4.119189519843966529, 2.378215178124999607 ) ) ;
#33068=CARTESIAN_POINT ( 'NONE',  ( 11.89687500061451608, -4.119189519843965641, -2.378215178125001383 ) ) ;
#33078=CARTESIAN_POINT ( 'NONE',  ( 14.29687500061451644, 4.119189519843966529, -2.378215178124998275 ) ) ;
#33093=CARTESIAN_POINT ( 'NONE',  ( 29.18437500061451217, 5.492252693125287522, 3.363034840372157021E-16 ) ) ;
#33094=CARTESIAN_POINT ( 'NONE',  ( 15.64687500061451608, -2.746126346562642428, -4.756430356249999214 ) ) ;
#33104=CARTESIAN_POINT ( 'NONE',  ( 13.10625000122903394, -4.330127018922190985, -2.500000000000001332 ) ) ;
#33107=CARTESIAN_POINT ( 'NONE',  ( 21.54375000122902861, -2.886751345948130876, 4.999999999999996447 ) ) ;
#33112=CARTESIAN_POINT ( 'NONE',  ( 25.96875000122903288, 2.886751345948126879, 4.999999999999999112 ) ) ;
#33125=FACE_OUTER_BOUND ( 'NONE', #64647, .T. ) ;
#33154=VERTEX_POINT ( 'NONE', #20878 ) ;
#33161=CARTESIAN_POINT ( 'NONE',  ( 20.37187500061451217, -4.119189519843968306, 2.378215178124996054 ) ) ;
#33169=ORIENTED_EDGE ( 'NONE', *, *, #26658, .T. ) ;
#33170=CARTESIAN_POINT ( 'NONE',  ( 10.49999999999999822, 4.330127018922192761, -2.499999999999997780 ) ) ;
#33177=CARTESIAN_POINT ( 'NONE',  ( 21.42187500061451644, -5.492252693125287522, -1.008910452111647106E-15 ) ) ;
#33180=CARTESIAN_POINT ( 'NONE',  ( 28.33125000122903359, -4.330127018922194537, 2.499999999999995559 ) ) ;
#33199=CARTESIAN_POINT ( 'NONE',  ( 9.121875000614517504, 2.746126346562643317, 4.756430356249998326 ) ) ;
#33207=ORIENTED_EDGE ( 'NONE', *, *, #62697, .T. ) ;
#33222=CARTESIAN_POINT ( 'NONE',  ( 12.68437500061451573, 4.119189519843966529, 2.378215178124999607 ) ) ;
#33245=CARTESIAN_POINT ( 'NONE',  ( 21.15937500061451715, 2.746126346562643317, 4.756430356249998326 ) ) ;
#33248=CARTESIAN_POINT ( 'NONE',  ( 13.63125000122903252, 6.123233995736764310E-16, -4.999999999999998224 ) ) ;
#33263=CARTESIAN_POINT ( 'NONE',  ( 7.809375000614515727, -5.492252693125287522, -1.008910452111647106E-15 ) ) ;
#33268=DIRECTION ( 'NONE',  ( -1.000000000000000000, -0.000000000000000000, -0.000000000000000000 ) ) ;
#33283=CARTESIAN_POINT ( 'NONE',  ( 16.39687500061451786, -2.746126346562646425, 4.756430356249996549 ) ) ;
#33316=CARTESIAN_POINT ( 'NONE',  ( 19.80937500061451573, 4.119189519843966529, -2.378215178124998275 ) ) ;
#33322=CARTESIAN_POINT ( 'NONE',  ( 19.34999999999999787, -4.330127018922190985, -2.500000000000001332 ) ) ;
#33326=CARTESIAN_POINT ( 'NONE',  ( 25.05937500061451217, 2.746126346562645981, -4.756430356249997438 ) ) ;
#33327=CARTESIAN_POINT ( 'NONE',  ( 18.99375000122903501, -2.886751345948209480, -4.999999999999856115 ) ) ;
#33330=CARTESIAN_POINT ( 'NONE',  ( 24.14999999999999858, 0.000000000000000000, 4.999999999999998224 ) ) ;
#33334=CARTESIAN_POINT ( 'NONE',  ( 26.18437500061451573, -2.746126346562646425, 4.756430356249996549 ) ) ;
#33336=CARTESIAN_POINT ( 'NONE',  ( 14.70937500061451608, 2.746126346562645981, -4.756430356249997438 ) ) ;
#33339=ORIENTED_EDGE ( 'NONE', *, *, #40326, .F. ) ;
#33344=EDGE_CURVE ( 'NONE', #45665, #29422, #32043, .T. ) ;
#33346=CARTESIAN_POINT ( 'NONE',  ( 18.52499999999999858, 6.123233995736764310E-16, -4.999999999999998224 ) ) ;
#33369=CARTESIAN_POINT ( 'NONE',  ( 24.60937500061451644, -4.119189519843965641, -2.378215178125001383 ) ) ;
#33371=CARTESIAN_POINT ( 'NONE',  ( 7.584375000614516082, 5.824947211148865298E-16, -4.756430356249998326 ) ) ;
#33377=CARTESIAN_POINT ( 'NONE',  ( 27.11250000000000071, 2.886751345948115333, -5.000000000000023093 ) ) ;
#33380=CARTESIAN_POINT ( 'NONE',  ( 7.743750001229034119, -2.886751345948126435, -5.000000000000000000 ) ) ;
#33387=CARTESIAN_POINT ( 'NONE',  ( 17.94375000122903074, -2.886751345948129988, 4.999999999999997335 ) ) ;
#33403=CARTESIAN_POINT ( 'NONE',  ( 25.09687500061451715, -2.746126346562642428, -4.756430356249999214 ) ) ;
#33408=CARTESIAN_POINT ( 'NONE',  ( 26.51249999999999929, -5.773502691896255534, -1.060575238724906372E-15 ) ) ;
#33415=CARTESIAN_POINT ( 'NONE',  ( 11.08125000122903181, 4.330127018922191873, 2.499999999999999556 ) ) ;
#33418=CARTESIAN_POINT ( 'NONE',  ( 20.78437500061451715, -2.746126346562646425, 4.756430356249996549 ) ) ;
#33428=CARTESIAN_POINT ( 'NONE',  ( 12.15937500061451360, 2.746126346562643317, 4.756430356249998326 ) ) ;
#33452=CARTESIAN_POINT ( 'NONE',  ( 14.59687500061452070, -2.746126346562646425, 4.756430356249996549 ) ) ;
#33468=CARTESIAN_POINT ( 'NONE',  ( 24.80625000122903145, -4.330127018922190985, -2.500000000000001332 ) ) ;
#33492=DIRECTION ( 'NONE',  ( -1.000000000000000000, -0.000000000000000000, -0.000000000000000000 ) ) ;
#33510=ORIENTED_EDGE ( 'NONE', *, *, #50852, .T. ) ;
#33513=CARTESIAN_POINT ( 'NONE',  ( 22.28437500061451360, -2.746126346562642428, -4.756430356249999214 ) ) ;
#33521=CARTESIAN_POINT ( 'NONE',  ( 7.724999999999999645, 6.123233995736764310E-16, -4.999999999999998224 ) ) ;
#33522=ORIENTED_EDGE ( 'NONE', *, *, #10883, .F. ) ;
#33524=CARTESIAN_POINT ( 'NONE',  ( 10.72500000000000142, -4.330127018922194537, 2.499999999999995559 ) ) ;
#33525=( BOUNDED_CURVE ( )  B_SPLINE_CURVE ( 2, ( #54171, #37536, #48998, #2460, #48265, #60058, #71529 ),
 .UNSPECIFIED., .F., .F. ) 
 B_SPLINE_CURVE_WITH_KNOTS ( ( 3, 2, 2, 3 ),
 ( 0.7000000000000001776, 0.7033333333333335879, 0.7066666666666668872, 0.7100000000000001865 ),
 .UNSPECIFIED. ) 
 CURVE ( )  GEOMETRIC_REPRESENTATION_ITEM ( )  RATIONAL_B_SPLINE_CURVE ( ( 0.9999999999999911182, 0.8660254037844475894, 1.000000000000000000, 0.8660254037844387076, 1.000000000000000000, 0.8660254037844298258, 1.000000000000008882 ) ) 
 REPRESENTATION_ITEM ( '' )  );
#33531=CYLINDRICAL_SURFACE ( 'NONE', #66977, 4.999999999999998224 ) ;
#33532=CARTESIAN_POINT ( 'NONE',  ( 21.83437500061451786, -4.119189519843968306, 2.378215178124996054 ) ) ;
#33535=CARTESIAN_POINT ( 'NONE',  ( 20.13750000000000639, -2.886751345948130876, 4.999999999999996447 ) ) ;
#33559=( BOUNDED_CURVE ( )  B_SPLINE_CURVE ( 2, ( #16485, #5421, #10597, #10958, #71928, #27227, #26866 ),
 .UNSPECIFIED., .F., .F. ) 
 B_SPLINE_CURVE_WITH_KNOTS ( ( 3, 2, 2, 3 ),
 ( 0.2499999999999999722, 0.2533333333333333548, 0.2566666666666667096, 0.2600000000000000644 ),
 .UNSPECIFIED. ) 
 CURVE ( )  GEOMETRIC_REPRESENTATION_ITEM ( )  RATIONAL_B_SPLINE_CURVE ( ( 1.000000000000001110, 0.8660254037844374864, 1.000000000000000000, 0.8660254037844387076, 1.000000000000000000, 0.8660254037844364872, 1.000000000000002220 ) ) 
 REPRESENTATION_ITEM ( '' )  );
#33575=ORIENTED_EDGE ( 'NONE', *, *, #35397, .T. ) ;
#33578=CARTESIAN_POINT ( 'NONE',  ( 17.21249999999999858, 2.886751345948073588, -5.000000000000094147 ) ) ;
#33580=CARTESIAN_POINT ( 'NONE',  ( 11.40937500061451892, 0.000000000000000000, 4.756430356249998326 ) ) ;
#33589=CARTESIAN_POINT ( 'NONE',  ( 12.11250000000000249, -5.773502691896255534, -1.060575238724906372E-15 ) ) ;
#33593=DIRECTION ( 'NONE',  ( -1.000000000000000000, -0.000000000000000000, -0.000000000000000000 ) ) ;
#33601=CARTESIAN_POINT ( 'NONE',  ( 19.69687500061451502, 4.119189519843966529, -2.378215178124998275 ) ) ;
#33604=CARTESIAN_POINT ( 'NONE',  ( 15.39375000122903181, -2.886751345948125991, -5.000000000000000000 ) ) ;
#33608=CARTESIAN_POINT ( 'NONE',  ( 27.00000000000000000, -4.330127018922190985, -2.500000000000001332 ) ) ;
#33619=CARTESIAN_POINT ( 'NONE',  ( 7.659375000614514484, 2.746126346562643317, 4.756430356249998326 ) ) ;
#33625=DIRECTION ( 'NONE',  ( -1.000000000000000000, -0.000000000000000000, -0.000000000000000000 ) ) ;
#33627=CARTESIAN_POINT ( 'NONE',  ( 15.07499999999999929, 4.330127018922191873, 2.499999999999999556 ) ) ;
#33642=CARTESIAN_POINT ( 'NONE',  ( 13.92187500061451289, 2.746126346562645981, -4.756430356249997438 ) ) ;
#33660=EDGE_CURVE ( 'NONE', #1565, #40669, #49515, .T. ) ;
#33670=CARTESIAN_POINT ( 'NONE',  ( 14.24999999999999822, 0.000000000000000000, 4.999999999999998224 ) ) ;
#33673=VECTOR ( 'NONE', #47141, 1000.000000000000000 ) ;
#33677=CARTESIAN_POINT ( 'NONE',  ( 18.04687500061451999, 5.492252693125287522, 3.363034840372157021E-16 ) ) ;
#33681=CARTESIAN_POINT ( 'NONE',  ( 19.57500000000000284, 4.330127018922191873, 2.499999999999999556 ) ) ;
#33684=CARTESIAN_POINT ( 'NONE',  ( 25.69687500061451502, 0.000000000000000000, 4.756430356249998326 ) ) ;
#33688=CARTESIAN_POINT ( 'NONE',  ( 24.82499999999999929, 6.123233995736764310E-16, -4.999999999999998224 ) ) ;
#33691=CARTESIAN_POINT ( 'NONE',  ( 26.14687500061451431, 0.000000000000000000, 4.756430356249998326 ) ) ;
#33693=CARTESIAN_POINT ( 'NONE',  ( 13.32187500061451502, 5.824947211148865298E-16, -4.756430356249998326 ) ) ;
#33702=CARTESIAN_POINT ( 'NONE',  ( 20.64375000122903359, -2.886751345948102898, 5.000000000000044409 ) ) ;
#33719=CARTESIAN_POINT ( 'NONE',  ( 45.00000000000000000, 0.000000000000000000, 4.999999999999998224 ) ) ;
#33720=ORIENTED_EDGE ( 'NONE', *, *, #45399, .F. ) ;
#33723=VECTOR ( 'NONE', #35433, 1000.000000000000000 ) ;
#33730=CARTESIAN_POINT ( 'NONE',  ( 24.94687500061451502, -2.746126346562646425, 4.756430356249996549 ) ) ;
#33748=CARTESIAN_POINT ( 'NONE',  ( 17.00625000122903074, 0.000000000000000000, 4.999999999999998224 ) ) ;
#33750=CARTESIAN_POINT ( 'NONE',  ( 45.00000000000000000, 0.000000000000000000, 0.000000000000000000 ) ) ;
#33762=VECTOR ( 'NONE', #47375, 1000.000000000000000 ) ;
#33764=CARTESIAN_POINT ( 'NONE',  ( 25.73437500061451644, 4.119189519843966529, 2.378215178124999607 ) ) ;
#33771=CARTESIAN_POINT ( 'NONE',  ( 28.12499999999999645, 4.330127018922191873, 2.499999999999999556 ) ) ;
#33773=CARTESIAN_POINT ( 'NONE',  ( 9.862499999999997158, -5.773502691896255534, -1.060575238724906372E-15 ) ) ;
#33779=CARTESIAN_POINT ( 'NONE',  ( 11.71875000122903465, -5.773502691896255534, -1.060575238724906372E-15 ) ) ;
#33781=CARTESIAN_POINT ( 'NONE',  ( 13.85625000122903216, 0.000000000000000000, 4.999999999999998224 ) ) ;
#33783=CARTESIAN_POINT ( 'NONE',  ( 21.72187500061451715, -4.119189519843968306, 2.378215178124996054 ) ) ;
#33789=CARTESIAN_POINT ( 'NONE',  ( 27.75000000000000000, 0.000000000000000000, 4.999999999999998224 ) ) ;
#33790=CARTESIAN_POINT ( 'NONE',  ( 10.93125000122903501, 6.123233995736764310E-16, -4.999999999999998224 ) ) ;
#33794=CARTESIAN_POINT ( 'NONE',  ( 12.57187500061451502, 4.119189519843966529, 2.378215178124999607 ) ) ;
#33800=ORIENTED_EDGE ( 'NONE', *, *, #24709, .F. ) ;
#33801=CARTESIAN_POINT ( 'NONE',  ( 21.16875000122903216, -5.773502691896255534, -1.060575238724906372E-15 ) ) ;
#33803=LINE ( 'NONE', #56347, #39480 ) ;
#33818=CARTESIAN_POINT ( 'NONE',  ( 13.92187500061451644, 2.746126346562645981, -4.756430356249997438 ) ) ;
#33837=CARTESIAN_POINT ( 'NONE',  ( 26.26875000122903359, 2.886751345948129099, -4.999999999999998224 ) ) ;
#33867=LINE ( 'NONE', #16510, #1785 ) ;
#33880=CARTESIAN_POINT ( 'NONE',  ( 18.98437500061451289, -2.746126346562646425, 4.756430356249996549 ) ) ;
#33896=CARTESIAN_POINT ( 'NONE',  ( 21.38437500061451502, -4.119189519843968306, 2.378215178124996054 ) ) ;
#33899=CARTESIAN_POINT ( 'NONE',  ( 12.75000000000000178, 4.330127018922192761, -2.499999999999997780 ) ) ;
#33907=VERTEX_POINT ( 'NONE', #25231 ) ;
#33919=CARTESIAN_POINT ( 'NONE',  ( 8.146875000614516082, 5.492252693125287522, 3.363034840372157021E-16 ) ) ;
#33939=CARTESIAN_POINT ( 'NONE',  ( 9.384375000614518569, 5.824947211148865298E-16, -4.756430356249998326 ) ) ;
#33940=DIRECTION ( 'NONE',  ( -1.000000000000000000, -0.000000000000000000, -0.000000000000000000 ) ) ;
#33944=AXIS2_PLACEMENT_3D ( 'NONE', #73003, #6851, #61910 ) ;
#33951=CARTESIAN_POINT ( 'NONE',  ( 29.85937500061451644, 0.000000000000000000, 4.756430356249998326 ) ) ;
#33960=( BOUNDED_CURVE ( )  B_SPLINE_CURVE ( 2, ( #72051, #17342, #62414, #72413, #16613, #32891, #39901 ),
 .UNSPECIFIED., .F., .F. ) 
 B_SPLINE_CURVE_WITH_KNOTS ( ( 3, 2, 2, 3 ),
 ( 0.3599999999999999867, 0.3633333333333333415, 0.3666666666666666408, 0.3699999999999999956 ),
 .UNSPECIFIED. ) 
 CURVE ( )  GEOMETRIC_REPRESENTATION_ITEM ( )  RATIONAL_B_SPLINE_CURVE ( ( 1.000000000000000000, 0.8660254037844387076, 1.000000000000000000, 0.8660254037844387076, 1.000000000000000000, 0.8660254037844387076, 1.000000000000000000 ) ) 
 REPRESENTATION_ITEM ( '' )  );
#33962=CARTESIAN_POINT ( 'NONE',  ( 17.44687500061451502, 4.119189519843966529, -2.378215178124998275 ) ) ;
#33965=CARTESIAN_POINT ( 'NONE',  ( 13.03125000122903110, -4.330127018922194537, 2.499999999999995559 ) ) ;
#33979=CARTESIAN_POINT ( 'NONE',  ( 29.10937500061451644, -4.119189519843965641, -2.378215178125001383 ) ) ;
#34002=CARTESIAN_POINT ( 'NONE',  ( 13.73437500061451821, -4.119189519843968306, 2.378215178124996054 ) ) ;
#34006=ORIENTED_EDGE ( 'NONE', *, *, #11564, .F. ) ;
#34016=ORIENTED_EDGE ( 'NONE', *, *, #48422, .T. ) ;
#34028=EDGE_LOOP ( 'NONE', ( #8358, #41983, #30572, #57847 ) ) ;
#34031=CARTESIAN_POINT ( 'NONE',  ( 17.82187500061451502, -5.492252693125287522, -1.008910452111647106E-15 ) ) ;
#34032=CYLINDRICAL_SURFACE ( 'NONE', #20829, 4.999999999999998224 ) ;
#34037=CARTESIAN_POINT ( 'NONE',  ( 20.47500000000000142, 4.330127018922191873, 2.499999999999999556 ) ) ;
#34041=CARTESIAN_POINT ( 'NONE',  ( 24.83437500061451431, -2.746126346562646425, 4.756430356249996549 ) ) ;
#34042=CARTESIAN_POINT ( 'NONE',  ( 12.67499999999999893, 6.123233995736764310E-16, -4.999999999999998224 ) ) ;
#34048=CARTESIAN_POINT ( 'NONE',  ( 24.27187500061451431, 4.119189519843966529, 2.378215178124999607 ) ) ;
#34050=CARTESIAN_POINT ( 'NONE',  ( 11.82187500061451502, -4.119189519843968306, 2.378215178124996054 ) ) ;
#34053=EDGE_LOOP ( 'NONE', ( #61234, #45254, #52697, #61245 ) ) ;
#34055=CARTESIAN_POINT ( 'NONE',  ( 25.94999999999999929, 0.000000000000000000, 4.999999999999998224 ) ) ;
#34060=EDGE_LOOP ( 'NONE', ( #6493, #6678, #26060, #22912 ) ) ;
#34066=EDGE_CURVE ( 'NONE', #17484, #71135, #58115, .T. ) ;
#34084=CARTESIAN_POINT ( 'NONE',  ( 20.85937500061451644, 0.000000000000000000, 4.756430356249998326 ) ) ;
#34105=CARTESIAN_POINT ( 'NONE',  ( 15.80625000122903145, -4.330127018922190985, -2.500000000000001332 ) ) ;
#34107=DIRECTION ( 'NONE',  ( 0.000000000000000000, 0.000000000000000000, 1.000000000000000000 ) ) ;
#34114=DIRECTION ( 'NONE',  ( -1.000000000000000000, -0.000000000000000000, -0.000000000000000000 ) ) ;
#34120=CARTESIAN_POINT ( 'NONE',  ( 26.03437500061451715, 5.824947211148865298E-16, -4.756430356249998326 ) ) ;
#34126=CARTESIAN_POINT ( 'NONE',  ( 26.47499999999999787, -4.330127018922194537, 2.499999999999995559 ) ) ;
#34128=CARTESIAN_POINT ( 'NONE',  ( 9.937500000000001776, -2.886751345948126435, -5.000000000000000000 ) ) ;
#34132=CARTESIAN_POINT ( 'NONE',  ( 23.08125000122903359, 6.123233995736764310E-16, -4.999999999999998224 ) ) ;
#34134=CARTESIAN_POINT ( 'NONE',  ( 11.83125000122903181, 6.123233995736764310E-16, -4.999999999999998224 ) ) ;
#34137=CARTESIAN_POINT ( 'NONE',  ( 18.27187500061451431, 5.824947211148865298E-16, -4.756430356249998326 ) ) ;
#34140=ORIENTED_EDGE ( 'NONE', *, *, #11487, .T. ) ;
#34143=CARTESIAN_POINT ( 'NONE',  ( 27.97500000000000142, 6.123233995736764310E-16, -4.999999999999998224 ) ) ;
#34145=CARTESIAN_POINT ( 'NONE',  ( 10.70625000122903536, 0.000000000000000000, 4.999999999999998224 ) ) ;
#34149=CARTESIAN_POINT ( 'NONE',  ( 13.99687500061451395, 0.000000000000000000, 4.756430356249998326 ) ) ;
#34150=ORIENTED_EDGE ( 'NONE', *, *, #66954, .F. ) ;
#34163=ORIENTED_EDGE ( 'NONE', *, *, #36053, .F. ) ;
#34169=CARTESIAN_POINT ( 'NONE',  ( 28.65937500061451715, -4.119189519843965641, -2.378215178125001383 ) ) ;
#34173=CARTESIAN_POINT ( 'NONE',  ( 13.99687500061451928, 5.492252693125287522, 3.363034840372157021E-16 ) ) ;
#34181=CARTESIAN_POINT ( 'NONE',  ( 8.137500000000002842, -2.886751345948126435, -5.000000000000000000 ) ) ;
#34191=CARTESIAN_POINT ( 'NONE',  ( 24.43125000122903145, 6.123233995736764310E-16, -4.999999999999998224 ) ) ;
#34218=EDGE_CURVE ( 'NONE', #7983, #24010, #69777, .T. ) ;
#34237=CARTESIAN_POINT ( 'NONE',  ( 19.62187500061451573, 5.824947211148865298E-16, -4.756430356249998326 ) ) ;
#34249=ADVANCED_FACE ( 'NONE', ( #59947 ), #55517, .T. ) ;
#34254=CARTESIAN_POINT ( 'NONE',  ( 19.02187500061451786, 2.746126346562643317, 4.756430356249998326 ) ) ;
#34257=CARTESIAN_POINT ( 'NONE',  ( 20.21250000000000213, -5.773502691896255534, -1.060575238724906372E-15 ) ) ;
#34264=DIRECTION ( 'NONE',  ( -1.000000000000000000, -0.000000000000000000, -0.000000000000000000 ) ) ;
#34271=LINE ( 'NONE', #18725, #25611 ) ;
#34277=CARTESIAN_POINT ( 'NONE',  ( 7.471875000614519813, -5.492252693125287522, -1.008910452111647106E-15 ) ) ;
#34287=ORIENTED_EDGE ( 'NONE', *, *, #41535, .F. ) ;
#34298=CARTESIAN_POINT ( 'NONE',  ( 9.009375000614518569, 4.119189519843966529, -2.378215178124998275 ) ) ;
#34318=CARTESIAN_POINT ( 'NONE',  ( 45.00000000000000000, 0.000000000000000000, 4.999999999999998224 ) ) ;
#34320=CARTESIAN_POINT ( 'NONE',  ( 17.78437500061451360, -2.746126346562642428, -4.756430356249999214 ) ) ;
#34323=CARTESIAN_POINT ( 'NONE',  ( 25.02187500061451431, 5.824947211148865298E-16, -4.756430356249998326 ) ) ;
#34337=CARTESIAN_POINT ( 'NONE',  ( 26.82187500061451857, -5.492252693125287522, -1.008910452111647106E-15 ) ) ;
#34347=VERTEX_POINT ( 'NONE', #15248 ) ;
#34358=CARTESIAN_POINT ( 'NONE',  ( 15.79687500061451644, 5.492252693125287522, 3.363034840372157021E-16 ) ) ;
#34362=ORIENTED_EDGE ( 'NONE', *, *, #42665, .F. ) ;
#34371=CARTESIAN_POINT ( 'NONE',  ( 29.38125000122903074, 6.123233995736764310E-16, -4.999999999999998224 ) ) ;
#34372=ORIENTED_EDGE ( 'NONE', *, *, #62833, .T. ) ;
#34390=CARTESIAN_POINT ( 'NONE',  ( 17.33437500061451431, -4.119189519843968306, 2.378215178124996054 ) ) ;
#34393=( BOUNDED_CURVE ( )  B_SPLINE_CURVE ( 2, ( #9699, #32232, #27065, #49596, #21137, #44056, #72121 ),
 .UNSPECIFIED., .F., .F. ) 
 B_SPLINE_CURVE_WITH_KNOTS ( ( 3, 2, 2, 3 ),
 ( 0.4099999999999999201, 0.4133333333333333304, 0.4166666666666667407, 0.4200000000000000955 ),
 .UNSPECIFIED. ) 
 CURVE ( )  GEOMETRIC_REPRESENTATION_ITEM ( )  RATIONAL_B_SPLINE_CURVE ( ( 1.000000000000002220, 0.8660254037844364872, 1.000000000000000000, 0.8660254037844387076, 1.000000000000000000, 0.8660254037844342667, 1.000000000000004441 ) ) 
 REPRESENTATION_ITEM ( '' )  );
#34396=ADVANCED_FACE ( 'NONE', ( #60672 ), #48516, .T. ) ;
#34400=CARTESIAN_POINT ( 'NONE',  ( 17.55000000000000071, -4.330127018922190985, -2.500000000000001332 ) ) ;
#34403=CARTESIAN_POINT ( 'NONE',  ( 26.84999999999999787, 0.000000000000000000, 4.999999999999998224 ) ) ;
#34404=CARTESIAN_POINT ( 'NONE',  ( 26.63437500061451502, -2.746126346562646425, 4.756430356249996549 ) ) ;
#34410=( BOUNDED_CURVE ( )  B_SPLINE_CURVE ( 2, ( #47863, #19394, #9435, #70392, #3166, #36040, #20493 ),
 .UNSPECIFIED., .F., .T. ) 
 B_SPLINE_CURVE_WITH_KNOTS ( ( 3, 2, 2, 3 ),
 ( 0.8200000000000000622, 0.8233333333333334725, 0.8266666666666667718, 0.8300000000000000711 ),
 .UNSPECIFIED. ) 
 CURVE ( )  GEOMETRIC_REPRESENTATION_ITEM ( )  RATIONAL_B_SPLINE_CURVE ( ( 0.9999999999999955591, 0.8660254037844431485, 1.000000000000000000, 0.8660254037844387076, 1.000000000000000000, 0.8660254037844342667, 1.000000000000004441 ) ) 
 REPRESENTATION_ITEM ( '' )  );
#34412=CARTESIAN_POINT ( 'NONE',  ( 24.79687500061451644, 0.000000000000000000, 4.756430356249998326 ) ) ;
#34414=CARTESIAN_POINT ( 'NONE',  ( 11.63437500061451502, 5.492252693125287522, 3.363034840372157021E-16 ) ) ;
#34423=DIRECTION ( 'NONE',  ( 0.000000000000000000, 0.000000000000000000, 1.000000000000000000 ) ) ;
#34426=CARTESIAN_POINT ( 'NONE',  ( 13.28437500061451537, -2.746126346562642428, -4.756430356249999214 ) ) ;
#34433=AXIS2_PLACEMENT_3D ( 'NONE', #9409, #61108, #4967 ) ;
#34438=ORIENTED_EDGE ( 'NONE', *, *, #26979, .T. ) ;
#34447=CARTESIAN_POINT ( 'NONE',  ( 22.13437500061451502, 4.119189519843966529, 2.378215178124999607 ) ) ;
#34454=ORIENTED_EDGE ( 'NONE', *, *, #9967, .F. ) ;
#34467=CARTESIAN_POINT ( 'NONE',  ( 16.96875000122903288, 2.886751345948126879, 4.999999999999999112 ) ) ;
#34469=FACE_OUTER_BOUND ( 'NONE', #5485, .T. ) ;
#34483=CARTESIAN_POINT ( 'NONE',  ( 24.75937500061451502, 4.119189519843966529, -2.378215178124998275 ) ) ;
#34489=CARTESIAN_POINT ( 'NONE',  ( 26.69999999999999929, 4.330127018922192761, -2.499999999999997780 ) ) ;
#34497=CARTESIAN_POINT ( 'NONE',  ( 9.581250001229033586, 6.123233995736764310E-16, -4.999999999999998224 ) ) ;
#34501=CARTESIAN_POINT ( 'NONE',  ( 17.89687500061451431, 4.119189519843966529, -2.378215178124998275 ) ) ;
#34508=CARTESIAN_POINT ( 'NONE',  ( 20.43749999999999645, 5.773502691896255534, 3.535250795749688401E-16 ) ) ;
#34512=CARTESIAN_POINT ( 'NONE',  ( 10.65937500061451892, 2.746126346562645981, -4.756430356249997438 ) ) ;
#34519=CARTESIAN_POINT ( 'NONE',  ( 19.65000000000000213, 0.000000000000000000, 4.999999999999998224 ) ) ;
#34521=CARTESIAN_POINT ( 'NONE',  ( 9.093750001229031099, -2.886751345948126435, -5.000000000000000000 ) ) ;
#34532=CARTESIAN_POINT ( 'NONE',  ( 29.25937500061451502, 4.119189519843966529, -2.378215178124998275 ) ) ;
#34535=CARTESIAN_POINT ( 'NONE',  ( 28.39687500061451431, 0.000000000000000000, 4.756430356249998326 ) ) ;
#34536=CARTESIAN_POINT ( 'NONE',  ( 13.28437500061451715, -4.119189519843968306, 2.378215178124996054 ) ) ;
#34544=EDGE_CURVE ( 'NONE', #21883, #38944, #54682, .T. ) ;
#34554=CARTESIAN_POINT ( 'NONE',  ( 22.25625000122903074, 4.330127018922192761, -2.499999999999997780 ) ) ;
#34579=CYLINDRICAL_SURFACE ( 'NONE', #67732, 4.999999999999998224 ) ;
#34583=CARTESIAN_POINT ( 'NONE',  ( 23.69999999999999929, 0.000000000000000000, 4.999999999999998224 ) ) ;
#34587=CARTESIAN_POINT ( 'NONE',  ( 17.96249999999999858, -5.773502691896255534, -1.060575238724906372E-15 ) ) ;
#34589=DIRECTION ( 'NONE',  ( 0.000000000000000000, 1.000000000000000000, -8.673617379884036705E-17 ) ) ;
#34596=VERTEX_POINT ( 'NONE', #17064 ) ;
#34602=CARTESIAN_POINT ( 'NONE',  ( 20.07187500061451502, 5.824947211148865298E-16, -4.756430356249998326 ) ) ;
#34610=CARTESIAN_POINT ( 'NONE',  ( 11.56875000122903430, 2.886751345948126879, 4.999999999999998224 ) ) ;
#34617=CARTESIAN_POINT ( 'NONE',  ( 22.16250000000000142, 2.886751345948073588, -5.000000000000094147 ) ) ;
#34618=CARTESIAN_POINT ( 'NONE',  ( 20.44687500061451857, -2.746126346562646425, 4.756430356249996549 ) ) ;
#34631=VERTEX_POINT ( 'NONE', #29912 ) ;
#34638=LINE ( 'NONE', #35007, #31523 ) ;
#34642=CARTESIAN_POINT ( 'NONE',  ( 8.446875000614518569, -2.746126346562641984, -4.756430356249999214 ) ) ;
#34664=CARTESIAN_POINT ( 'NONE',  ( 9.459375000614517859, 4.119189519843966529, -2.378215178124998275 ) ) ;
#34679=CYLINDRICAL_SURFACE ( 'NONE', #10049, 4.999999999999998224 ) ;
#34685=CARTESIAN_POINT ( 'NONE',  ( 17.03437500061451715, 5.492252693125287522, 3.363034840372157021E-16 ) ) ;
#34688=CARTESIAN_POINT ( 'NONE',  ( 26.48437500061450933, 5.492252693125287522, 3.363034840372157021E-16 ) ) ;
#34693=CARTESIAN_POINT ( 'NONE',  ( 28.64999999999999858, 0.000000000000000000, 4.999999999999998224 ) ) ;
#34703=CARTESIAN_POINT ( 'NONE',  ( 27.12187500061451573, 2.746126346562643317, 4.756430356249998326 ) ) ;
#34709=CYLINDRICAL_SURFACE ( 'NONE', #45487, 4.999999999999998224 ) ;
#34721=CARTESIAN_POINT ( 'NONE',  ( 15.64687500061451608, -2.746126346562641984, -4.756430356249999214 ) ) ;
#34725=VERTEX_POINT ( 'NONE', #7872 ) ;
#34726=EDGE_CURVE ( 'NONE', #44169, #2080, #41851, .T. ) ;
#34753=CARTESIAN_POINT ( 'NONE',  ( 17.18437500061451573, 4.119189519843966529, 2.378215178124999607 ) ) ;
#34760=CARTESIAN_POINT ( 'NONE',  ( 17.47499999999999787, -4.330127018922194537, 2.499999999999995559 ) ) ;
#34765=CARTESIAN_POINT ( 'NONE',  ( 25.99687500061451573, 4.119189519843966529, -2.378215178124998275 ) ) ;
#34774=CARTESIAN_POINT ( 'NONE',  ( 23.70937500061451075, 2.746126346562645981, -4.756430356249997438 ) ) ;
#34776=CARTESIAN_POINT ( 'NONE',  ( 11.37187500061451573, -4.119189519843968306, 2.378215178124996054 ) ) ;
#34785=CARTESIAN_POINT ( 'NONE',  ( 17.66249999999999787, 2.886751345948185055, -4.999999999999902300 ) ) ;
#34788=CARTESIAN_POINT ( 'NONE',  ( 11.25937500061451679, 2.746126346562643317, 4.756430356249998326 ) ) ;
#34807=VECTOR ( 'NONE', #2426, 1000.000000000000000 ) ;
#34809=CARTESIAN_POINT ( 'NONE',  ( 22.28437500061451715, -4.119189519843968306, 2.378215178124996054 ) ) ;
#34819=EDGE_CURVE ( 'NONE', #24506, #57706, #24851, .T. ) ;
#34823=CARTESIAN_POINT ( 'NONE',  ( 15.20625000122903181, 0.000000000000000000, 4.999999999999998224 ) ) ;
#34832=CARTESIAN_POINT ( 'NONE',  ( 16.44375000122903074, 5.773502691896255534, 3.535250795749688894E-16 ) ) ;
#34834=DIRECTION ( 'NONE',  ( 0.000000000000000000, 0.000000000000000000, 1.000000000000000000 ) ) ;
#34840=CARTESIAN_POINT ( 'NONE',  ( 10.83750000000000036, -2.886751345948237457, -4.999999999999807265 ) ) ;
#34848=CARTESIAN_POINT ( 'NONE',  ( 24.00937500061451502, 0.000000000000000000, 4.756430356249998326 ) ) ;
#34853=CARTESIAN_POINT ( 'NONE',  ( 25.80000000000000071, 4.330127018922192761, -2.499999999999997780 ) ) ;
#34862=CARTESIAN_POINT ( 'NONE',  ( 10.06875000122903252, 2.886751345948129099, -4.999999999999998224 ) ) ;
#34863=CARTESIAN_POINT ( 'NONE',  ( 18.97499999999999787, 6.123233995736764310E-16, -4.999999999999998224 ) ) ;
#34865=CARTESIAN_POINT ( 'NONE',  ( 17.52187500061451431, 4.119189519843966529, 2.378215178124999607 ) ) ;
#34876=CARTESIAN_POINT ( 'NONE',  ( 11.22187500061451537, 4.119189519843966529, 2.378215178124999607 ) ) ;
#34882=ORIENTED_EDGE ( 'NONE', *, *, #34218, .F. ) ;
#34883=EDGE_CURVE ( 'NONE', #58840, #63177, #53671, .T. ) ;
#34886=DIRECTION ( 'NONE',  ( -1.000000000000000000, -0.000000000000000000, -0.000000000000000000 ) ) ;
#34890=CARTESIAN_POINT ( 'NONE',  ( 10.16249999999999964, 2.886751345948126879, 4.999999999999999112 ) ) ;
#34893=ORIENTED_EDGE ( 'NONE', *, *, #47275, .T. ) ;
#34900=CARTESIAN_POINT ( 'NONE',  ( 29.22187500061451715, 2.746126346562645981, -4.756430356249997438 ) ) ;
#34903=CARTESIAN_POINT ( 'NONE',  ( 27.79687500061451289, 4.119189519843966529, -2.378215178124998275 ) ) ;
#34904=CARTESIAN_POINT ( 'NONE',  ( 12.64687500061451608, 5.492252693125287522, 3.363034840372157021E-16 ) ) ;
#34921=CARTESIAN_POINT ( 'NONE',  ( 23.04375000122903216, -2.886751345948125991, -5.000000000000000000 ) ) ;
#34947=CARTESIAN_POINT ( 'NONE',  ( 22.33125000122903003, 4.330127018922191873, 2.499999999999999556 ) ) ;
#34955=CARTESIAN_POINT ( 'NONE',  ( 19.25625000122903430, 0.000000000000000000, 4.999999999999998224 ) ) ;
#34959=EDGE_LOOP ( 'NONE', ( #72249, #31278, #12968, #39766 ) ) ;
#34964=CARTESIAN_POINT ( 'NONE',  ( 27.58125000122903359, 6.123233995736764310E-16, -4.999999999999998224 ) ) ;
#34969=VERTEX_POINT ( 'NONE', #42586 ) ;
#34972=CARTESIAN_POINT ( 'NONE',  ( 18.49687500061451573, 0.000000000000000000, 4.756430356249998326 ) ) ;
#34981=CYLINDRICAL_SURFACE ( 'NONE', #4159, 4.999999999999998224 ) ;
#34990=CARTESIAN_POINT ( 'NONE',  ( 20.29687500061451644, 5.492252693125287522, 3.363034840372157021E-16 ) ) ;
#35002=ORIENTED_EDGE ( 'NONE', *, *, #68503, .F. ) ;
#35007=CARTESIAN_POINT ( 'NONE',  ( -5.000000000000000000, 0.000000000000000000, 50.00000000000000000 ) ) ;
#35011=CARTESIAN_POINT ( 'NONE',  ( 8.409375000614518925, -4.119189519843965641, -2.378215178125001383 ) ) ;
#35032=CARTESIAN_POINT ( 'NONE',  ( 27.99375000122903145, -2.886751345948126435, -5.000000000000000000 ) ) ;
#35033=CARTESIAN_POINT ( 'NONE',  ( 9.084375000614517859, 4.119189519843966529, 2.378215178124999607 ) ) ;
#35035=CARTESIAN_POINT ( 'NONE',  ( 24.14999999999999858, 0.000000000000000000, 4.999999999999998224 ) ) ;
#35051=CARTESIAN_POINT ( 'NONE',  ( 22.85625000122903216, 0.000000000000000000, 4.999999999999998224 ) ) ;
#35052=( BOUNDED_CURVE ( )  B_SPLINE_CURVE ( 2, ( #47687, #70591, #59492, #31061, #2625, #54342, #19966 ),
 .UNSPECIFIED., .F., .F. ) 
 B_SPLINE_CURVE_WITH_KNOTS ( ( 3, 2, 2, 3 ),
 ( 0.9200000000000001510, 0.9233333333333334503, 0.9266666666666667496, 0.9300000000000001599 ),
 .UNSPECIFIED. ) 
 CURVE ( )  GEOMETRIC_REPRESENTATION_ITEM ( )  RATIONAL_B_SPLINE_CURVE ( ( 0.9999999999999955591, 0.8660254037844431485, 1.000000000000000000, 0.8660254037844387076, 1.000000000000000000, 0.8660254037844342667, 1.000000000000004441 ) ) 
 REPRESENTATION_ITEM ( '' )  );
#35055=CARTESIAN_POINT ( 'NONE',  ( 16.62187500061451573, 4.119189519843966529, 2.378215178124999607 ) ) ;
#35058=CARTESIAN_POINT ( 'NONE',  ( 27.08437500061451431, -2.746126346562646425, 4.756430356249996549 ) ) ;
#35066=CARTESIAN_POINT ( 'NONE',  ( 21.91875000122903216, 2.886751345948154857, 4.999999999999951150 ) ) ;
#35073=CARTESIAN_POINT ( 'NONE',  ( 27.72187500061451715, -5.492252693125287522, -1.008910452111647106E-15 ) ) ;
#35092=CARTESIAN_POINT ( 'NONE',  ( 15.75937500061451857, 4.119189519843966529, -2.378215178124998275 ) ) ;
#35104=CARTESIAN_POINT ( 'NONE',  ( 29.23125000122903216, -4.330127018922194537, 2.499999999999995559 ) ) ;
#35105=ORIENTED_EDGE ( 'NONE', *, *, #43096, .T. ) ;
#35121=UNCERTAINTY_MEASURE_WITH_UNIT (LENGTH_MEASURE( 1.000000000000000082E-05 ), #24909, 'distance_accuracy_value', 'NONE');
#35123=CARTESIAN_POINT ( 'NONE',  ( 15.75937500061451857, 4.119189519843966529, -2.378215178124998275 ) ) ;
#35129=CARTESIAN_POINT ( 'NONE',  ( 18.18750000000000000, 5.773502691896255534, 3.535250795749688894E-16 ) ) ;
#35133=CARTESIAN_POINT ( 'NONE',  ( 24.15937500061451715, 2.746126346562645981, -4.756430356249997438 ) ) ;
#35142=CARTESIAN_POINT ( 'NONE',  ( 25.43437500061451217, -2.746126346562642428, -4.756430356249999214 ) ) ;
#35144=CARTESIAN_POINT ( 'NONE',  ( 11.14687500061451608, 4.119189519843966529, -2.378215178124998275 ) ) ;
#35153=CARTESIAN_POINT ( 'NONE',  ( 17.84999999999999787, 0.000000000000000000, 4.999999999999998224 ) ) ;
#35156=CARTESIAN_POINT ( 'NONE',  ( 11.48437500061451821, -2.746126346562642428, -4.756430356249999214 ) ) ;
#35167=ORIENTED_EDGE ( 'NONE', *, *, #24217, .T. ) ;
#35173=CARTESIAN_POINT ( 'NONE',  ( 11.55000000000000071, 0.000000000000000000, 4.999999999999998224 ) ) ;
#35175=CARTESIAN_POINT ( 'NONE',  ( 21.27187500061451786, 2.746126346562643317, 4.756430356249998326 ) ) ;
#35191=CYLINDRICAL_SURFACE ( 'NONE', #19753, 4.999999999999998224 ) ;
#35194=CARTESIAN_POINT ( 'NONE',  ( 16.14375000122903359, -2.886751345948129988, 4.999999999999997335 ) ) ;
#35196=CARTESIAN_POINT ( 'NONE',  ( 10.18125000122903323, 4.330127018922191873, 2.499999999999999556 ) ) ;
#35212=CARTESIAN_POINT ( 'NONE',  ( 22.62187500061451573, 2.746126346562643317, 4.756430356249998326 ) ) ;
#35216=( BOUNDED_CURVE ( )  B_SPLINE_CURVE ( 2, ( #58186, #30128, #1702, #64466, #52659, #53023, #63016 ),
 .UNSPECIFIED., .F., .F. ) 
 B_SPLINE_CURVE_WITH_KNOTS ( ( 3, 2, 2, 3 ),
 ( 0.2000000000000000389, 0.2033333333333333659, 0.2066666666666667207, 0.2100000000000000477 ),
 .UNSPECIFIED. ) 
 CURVE ( )  GEOMETRIC_REPRESENTATION_ITEM ( )  RATIONAL_B_SPLINE_CURVE ( ( 0.9999999999999988898, 0.8660254037844398178, 1.000000000000000000, 0.8660254037844387076, 1.000000000000000000, 0.8660254037844364872, 1.000000000000002220 ) ) 
 REPRESENTATION_ITEM ( '' )  );
#35218=CARTESIAN_POINT ( 'NONE',  ( 25.50000000000000000, 0.000000000000000000, 4.999999999999998224 ) ) ;
#35221=CARTESIAN_POINT ( 'NONE',  ( 12.84375000122903288, 5.773502691896255534, 3.535250795749688401E-16 ) ) ;
#35222=EDGE_CURVE ( 'NONE', #28145, #37967, #32600, .T. ) ;
#35225=CARTESIAN_POINT ( 'NONE',  ( 22.89375000122903003, -2.886751345948130876, 4.999999999999996447 ) ) ;
#35227=CARTESIAN_POINT ( 'NONE',  ( 9.318750001229034297, 2.886751345948126879, 4.999999999999999112 ) ) ;
#35230=CARTESIAN_POINT ( 'NONE',  ( 18.60937500061450578, -5.492252693125287522, -1.008910452111647106E-15 ) ) ;
#35241=CARTESIAN_POINT ( 'NONE',  ( 10.88437500061451679, -2.746126346562646425, 4.756430356249996549 ) ) ;
#35249=CARTESIAN_POINT ( 'NONE',  ( 9.131250001229034297, 6.123233995736764310E-16, -4.999999999999998224 ) ) ;
#35253=CARTESIAN_POINT ( 'NONE',  ( 10.95000000000000107, 4.330127018922192761, -2.499999999999997780 ) ) ;
#35261=CARTESIAN_POINT ( 'NONE',  ( 29.82187500061451502, 2.746126346562643317, 4.756430356249998326 ) ) ;
#35263=CARTESIAN_POINT ( 'NONE',  ( 27.53437500061451360, -2.746126346562646425, 4.756430356249996549 ) ) ;
#35264=CARTESIAN_POINT ( 'NONE',  ( 12.19687500061451679, 5.492252693125287522, 3.363034840372157021E-16 ) ) ;
#35280=CARTESIAN_POINT ( 'NONE',  ( 22.78125000122903288, 4.330127018922191873, 2.499999999999999556 ) ) ;
#35290=EDGE_CURVE ( 'NONE', #10453, #1565, #34393, .T. ) ;
#35317=ORIENTED_EDGE ( 'NONE', *, *, #46133, .F. ) ;
#35331=CARTESIAN_POINT ( 'NONE',  ( 18.15937500061451715, -5.492252693125287522, -1.008910452111647106E-15 ) ) ;
#35348=CARTESIAN_POINT ( 'NONE',  ( 20.59687500061451360, -2.746126346562642428, -4.756430356249999214 ) ) ;
#35367=DIRECTION ( 'NONE',  ( -1.000000000000000000, -0.000000000000000000, -0.000000000000000000 ) ) ;
#35372=CARTESIAN_POINT ( 'NONE',  ( 22.81875000122903074, 2.886751345948126879, 4.999999999999998224 ) ) ;
#35381=VERTEX_POINT ( 'NONE', #5252 ) ;
#35392=CARTESIAN_POINT ( 'NONE',  ( 8.409375000614518925, -4.119189519843965641, -2.378215178125001383 ) ) ;
#35397=EDGE_CURVE ( 'NONE', #49807, #57706, #39596, .T. ) ;
#35403=CARTESIAN_POINT ( 'NONE',  ( 24.20625000122903359, 0.000000000000000000, 4.999999999999998224 ) ) ;
#35412=CARTESIAN_POINT ( 'NONE',  ( 18.57187500061451857, -4.119189519843968306, 2.378215178124996054 ) ) ;
#35415=CARTESIAN_POINT ( 'NONE',  ( 25.95937500061451431, 2.746126346562645981, -4.756430356249997438 ) ) ;
#35430=CARTESIAN_POINT ( 'NONE',  ( 27.04687500061451644, 5.492252693125287522, 3.363034840372157021E-16 ) ) ;
#35433=DIRECTION ( 'NONE',  ( -1.000000000000000000, -0.000000000000000000, -0.000000000000000000 ) ) ;
#35448=CARTESIAN_POINT ( 'NONE',  ( 11.33437500061451608, 4.119189519843966529, 2.378215178124999607 ) ) ;
#35460=EDGE_CURVE ( 'NONE', #61955, #4995, #68763, .T. ) ;
#35477=EDGE_LOOP ( 'NONE', ( #2959, #13324, #66476, #26123 ) ) ;
#35481=CARTESIAN_POINT ( 'NONE',  ( 17.40937500061451715, -4.119189519843965641, -2.378215178125001383 ) ) ;
#35485=( BOUNDED_CURVE ( )  B_SPLINE_CURVE ( 2, ( #36563, #59820, #55023, #59083, #8487, #9225, #15120 ),
 .UNSPECIFIED., .F., .F. ) 
 B_SPLINE_CURVE_WITH_KNOTS ( ( 3, 2, 2, 3 ),
 ( 0.6500000000000000222, 0.6533333333333333215, 0.6566666666666666208, 0.6600000000000000311 ),
 .UNSPECIFIED. ) 
 CURVE ( )  GEOMETRIC_REPRESENTATION_ITEM ( )  RATIONAL_B_SPLINE_CURVE ( ( 1.000000000000000000, 0.8660254037844387076, 1.000000000000000000, 0.8660254037844387076, 1.000000000000000000, 0.8660254037844387076, 1.000000000000000000 ) ) 
 REPRESENTATION_ITEM ( '' )  );
#35489=CARTESIAN_POINT ( 'NONE',  ( 16.68750000000000000, -2.886751345948125991, -5.000000000000000000 ) ) ;
#35493=CARTESIAN_POINT ( 'NONE',  ( 22.69687500061451502, -4.119189519843965641, -2.378215178125001383 ) ) ;
#35500=CARTESIAN_POINT ( 'NONE',  ( 25.58437500061451431, 5.492252693125287522, 3.363034840372157021E-16 ) ) ;
#35503=CARTESIAN_POINT ( 'NONE',  ( 12.12187500061451573, 4.119189519843966529, 2.378215178124999607 ) ) ;
#35511=LINE ( 'NONE', #69861, #27835 ) ;
#35513=EDGE_LOOP ( 'NONE', ( #17174, #41361, #34016, #44889 ) ) ;
#35515=CARTESIAN_POINT ( 'NONE',  ( 11.93437500061451750, -2.746126346562642428, -4.756430356249999214 ) ) ;
#35533=CARTESIAN_POINT ( 'NONE',  ( 21.15937500061451715, 4.119189519843966529, -2.378215178124998275 ) ) ;
#35536=VECTOR ( 'NONE', #47917, 1000.000000000000000 ) ;
#35546=CARTESIAN_POINT ( 'NONE',  ( 7.556250001229035007, 0.000000000000000000, 4.999999999999998224 ) ) ;
#35555=CARTESIAN_POINT ( 'NONE',  ( 9.375000000000001776, -4.330127018922194537, 2.499999999999995559 ) ) ;
#35566=VERTEX_POINT ( 'NONE', #34403 ) ;
#35570=CARTESIAN_POINT ( 'NONE',  ( 23.44687500061451502, 5.492252693125287522, 3.363034840372157021E-16 ) ) ;
#35575=CARTESIAN_POINT ( 'NONE',  ( 24.33749999999999858, -2.886751345948125991, -5.000000000000000000 ) ) ;
#35584=CARTESIAN_POINT ( 'NONE',  ( 15.15000000000000036, 0.000000000000000000, 4.999999999999998224 ) ) ;
#35586=CARTESIAN_POINT ( 'NONE',  ( 9.843750001229032875, -2.886751345948129988, 4.999999999999997335 ) ) ;
#35589=CARTESIAN_POINT ( 'NONE',  ( 17.93437500061451928, 5.492252693125287522, 3.363034840372157021E-16 ) ) ;
#35596=ADVANCED_FACE ( 'NONE', ( #45510 ), #63203, .T. ) ;
#35600=CARTESIAN_POINT ( 'NONE',  ( 9.684375000614517504, -2.746126346562642428, -4.756430356249999214 ) ) ;
#35611=CARTESIAN_POINT ( 'NONE',  ( 28.84687500061451360, 0.000000000000000000, 4.756430356249998326 ) ) ;
#35614=CARTESIAN_POINT ( 'NONE',  ( 7.762500000000001954, 2.886751345948129099, -4.999999999999998224 ) ) ;
#35622=CARTESIAN_POINT ( 'NONE',  ( 28.28437500061451715, 5.824947211148865298E-16, -4.756430356249998326 ) ) ;
#35624=CARTESIAN_POINT ( 'NONE',  ( 27.04687500061451289, 0.000000000000000000, 4.756430356249998326 ) ) ;
#35625=CARTESIAN_POINT ( 'NONE',  ( 11.10937500061451644, -4.119189519843965641, -2.378215178125001383 ) ) ;
#35640=CARTESIAN_POINT ( 'NONE',  ( 24.28125000122903288, -4.330127018922194537, 2.499999999999995559 ) ) ;
#35643=ORIENTED_EDGE ( 'NONE', *, *, #22404, .T. ) ;
#35658=CARTESIAN_POINT ( 'NONE',  ( 29.85937500061451644, 0.000000000000000000, 4.756430356249998326 ) ) ;
#35680=CARTESIAN_POINT ( 'NONE',  ( 12.28125000122903110, 6.123233995736764310E-16, -4.999999999999998224 ) ) ;
#35685=ORIENTED_EDGE ( 'NONE', *, *, #41825, .T. ) ;
#35690=VECTOR ( 'NONE', #41509, 1000.000000000000000 ) ;
#35693=CARTESIAN_POINT ( 'NONE',  ( 16.92187500061451644, 5.824947211148865298E-16, -4.756430356249998326 ) ) ;
#35708=CARTESIAN_POINT ( 'NONE',  ( 8.456250001229033586, 0.000000000000000000, 4.999999999999998224 ) ) ;
#35711=CARTESIAN_POINT ( 'NONE',  ( 19.58437500061451786, -4.119189519843968306, 2.378215178124996054 ) ) ;
#35722=FACE_OUTER_BOUND ( 'NONE', #71628, .T. ) ;
#35723=EDGE_LOOP ( 'NONE', ( #42695, #780, #56798, #32030 ) ) ;
#35733=CARTESIAN_POINT ( 'NONE',  ( 7.650000000000000355, -4.330127018922190985, -2.500000000000001332 ) ) ;
#35734=FACE_OUTER_BOUND ( 'NONE', #61060, .T. ) ;
#35755=CARTESIAN_POINT ( 'NONE',  ( 28.76249999999999929, -5.773502691896255534, -1.060575238724906372E-15 ) ) ;
#35765=DIRECTION ( 'NONE',  ( 0.000000000000000000, 0.000000000000000000, 1.000000000000000000 ) ) ;
#35773=CARTESIAN_POINT ( 'NONE',  ( 16.20937500061451431, 2.746126346562643317, 4.756430356249998326 ) ) ;
#35776=CARTESIAN_POINT ( 'NONE',  ( 24.83437500061451075, -2.746126346562646425, 4.756430356249996549 ) ) ;
#35782=CARTESIAN_POINT ( 'NONE',  ( 21.76875000122904069, 2.886751345948073588, -5.000000000000094147 ) ) ;
#35790=CARTESIAN_POINT ( 'NONE',  ( 26.33437500061451431, -4.119189519843968306, 2.378215178124996054 ) ) ;
#35793=LINE ( 'NONE', #40998, #33723 ) ;
#35798=EDGE_CURVE ( 'NONE', #23511, #50673, #67677, .T. ) ;
#35809=CARTESIAN_POINT ( 'NONE',  ( 11.29687500061451644, 5.492252693125287522, 3.363034840372157021E-16 ) ) ;
#35834=ORIENTED_EDGE ( 'NONE', *, *, #10973, .T. ) ;
#35838=CARTESIAN_POINT ( 'NONE',  ( 17.07187500061451502, 2.746126346562645981, -4.756430356249997438 ) ) ;
#35845=CARTESIAN_POINT ( 'NONE',  ( 17.73750000000000071, 5.773502691896255534, 3.535250795749688894E-16 ) ) ;
#35850=CARTESIAN_POINT ( 'NONE',  ( 22.43437500061451573, 5.492252693125287522, 3.363034840372157021E-16 ) ) ;
#35858=CARTESIAN_POINT ( 'NONE',  ( 22.43437500061451217, 5.492252693125287522, 3.363034840372157021E-16 ) ) ;
#35860=CARTESIAN_POINT ( 'NONE',  ( 9.759375000614516793, 2.746126346562645981, -4.756430356249997438 ) ) ;
#35868=CARTESIAN_POINT ( 'NONE',  ( 12.50625000122903430, 0.000000000000000000, 4.999999999999998224 ) ) ;
#35869=ORIENTED_EDGE ( 'NONE', *, *, #43284, .F. ) ;
#35871=CARTESIAN_POINT ( 'NONE',  ( 11.52187500061451608, 5.824947211148865298E-16, -4.756430356249998326 ) ) ;
#35889=CARTESIAN_POINT ( 'NONE',  ( 12.13125000122903430, -4.330127018922194537, 2.499999999999995559 ) ) ;
#35892=CARTESIAN_POINT ( 'NONE',  ( 19.73437500061451644, 5.824947211148865298E-16, -4.756430356249998326 ) ) ;
#35914=CARTESIAN_POINT ( 'NONE',  ( 10.14375000122903181, 5.773502691896255534, 3.535250795749688401E-16 ) ) ;
#35924=( BOUNDED_CURVE ( )  B_SPLINE_CURVE ( 2, ( #30919, #64166, #35733, #58253, #30198, #25380, #1773 ),
 .UNSPECIFIED., .F., .F. ) 
 B_SPLINE_CURVE_WITH_KNOTS ( ( 3, 2, 2, 3 ),
 ( 0.9900000000000002132, 0.9933333333333334014, 0.9966666666666668117, 1.000000000000000000 ),
 .UNSPECIFIED. ) 
 CURVE ( )  GEOMETRIC_REPRESENTATION_ITEM ( )  RATIONAL_B_SPLINE_CURVE ( ( 0.9999999999999911182, 0.8660254037844475894, 1.000000000000000000, 0.8660254037844387076, 1.000000000000000000, 0.8660254037844387076, 1.000000000000000000 ) ) 
 REPRESENTATION_ITEM ( '' )  );
#35927=VECTOR ( 'NONE', #29236, 1000.000000000000000 ) ;
#35929=CARTESIAN_POINT ( 'NONE',  ( 23.40937500061451715, 4.119189519843966529, -2.378215178124998275 ) ) ;
#35934=CARTESIAN_POINT ( 'NONE',  ( 25.34999999999999787, 4.330127018922192761, -2.499999999999997780 ) ) ;
#35946=CARTESIAN_POINT ( 'NONE',  ( 10.21875000122903288, 2.886751345948126879, 4.999999999999999112 ) ) ;
#35948=CARTESIAN_POINT ( 'NONE',  ( 16.54687500061451644, 4.119189519843966529, -2.378215178124998275 ) ) ;
#35957=DIRECTION ( 'NONE',  ( -0.000000000000000000, -1.000000000000000000, 8.673617379884035472E-17 ) ) ;
#35961=CARTESIAN_POINT ( 'NONE',  ( 10.48125000122903216, 6.123233995736764310E-16, -4.999999999999998224 ) ) ;
#35962=CARTESIAN_POINT ( 'NONE',  ( 9.309375000614515727, 2.746126346562645981, -4.756430356249997438 ) ) ;
#35969=ORIENTED_EDGE ( 'NONE', *, *, #35460, .T. ) ;
#35972=CARTESIAN_POINT ( 'NONE',  ( 8.906250001229031099, 0.000000000000000000, 4.999999999999998224 ) ) ;
#35974=CARTESIAN_POINT ( 'NONE',  ( 28.02187500061451431, -4.119189519843968306, 2.378215178124996054 ) ) ;
#35977=CARTESIAN_POINT ( 'NONE',  ( 8.175000000000002487, 6.123233995736764310E-16, -4.999999999999998224 ) ) ;
#35978=AXIS2_PLACEMENT_3D ( 'NONE', #31968, #70758, #20133 ) ;
#35986=CARTESIAN_POINT ( 'NONE',  ( 27.42187500061451644, 2.746126346562645981, -4.756430356249997438 ) ) ;
#35988=CARTESIAN_POINT ( 'NONE',  ( 27.57187500061451502, -4.119189519843968306, 2.378215178124996054 ) ) ;
#35989=CARTESIAN_POINT ( 'NONE',  ( 10.28437500061451715, 5.824947211148865298E-16, -4.756430356249998326 ) ) ;
#35994=CARTESIAN_POINT ( 'NONE',  ( 45.00000000000000000, 6.123233995736764310E-16, -4.999999999999998224 ) ) ;
#36003=CARTESIAN_POINT ( 'NONE',  ( 21.35625000122903216, 4.330127018922192761, -2.499999999999997780 ) ) ;
#36005=CARTESIAN_POINT ( 'NONE',  ( 22.72499999999999787, 4.330127018922191873, 2.499999999999999556 ) ) ;
#36006=ORIENTED_EDGE ( 'NONE', *, *, #51854, .T. ) ;
#36009=EDGE_CURVE ( 'NONE', #1724, #68363, #25503, .T. ) ;
#36018=VECTOR ( 'NONE', #36901, 1000.000000000000000 ) ;
#36026=AXIS2_PLACEMENT_3D ( 'NONE', #6641, #22879, #45437 ) ;
#36028=AXIS2_PLACEMENT_3D ( 'NONE', #32270, #54803, #9374 ) ;
#36031=DIRECTION ( 'NONE',  ( -1.000000000000000000, -0.000000000000000000, -0.000000000000000000 ) ) ;
#36039=CARTESIAN_POINT ( 'NONE',  ( 19.36875000122903501, -5.773502691896255534, -1.060575238724906372E-15 ) ) ;
#36040=CARTESIAN_POINT ( 'NONE',  ( 10.96875000122903110, 2.886751345948073588, -5.000000000000094147 ) ) ;
#36044=CARTESIAN_POINT ( 'NONE',  ( 20.10000000000000142, 0.000000000000000000, 4.999999999999998224 ) ) ;
#36051=ORIENTED_EDGE ( 'NONE', *, *, #11681, .F. ) ;
#36053=EDGE_CURVE ( 'NONE', #51146, #48021, #24473, .T. ) ;
#36055=ORIENTED_EDGE ( 'NONE', *, *, #72027, .F. ) ;
#36056=CARTESIAN_POINT ( 'NONE',  ( 26.62500000000000000, 6.123233995736764310E-16, -4.999999999999998224 ) ) ;
#36059=CARTESIAN_POINT ( 'NONE',  ( 16.88437500061451857, -2.746126346562642428, -4.756430356249999214 ) ) ;
#36079=CARTESIAN_POINT ( 'NONE',  ( 18.60937500061451644, 0.000000000000000000, 4.756430356249998326 ) ) ;
#36097=CARTESIAN_POINT ( 'NONE',  ( 29.34375000122903288, -2.886751345948125991, -5.000000000000000000 ) ) ;
#36109=VERTEX_POINT ( 'NONE', #59105 ) ;
#36115=ADVANCED_FACE ( 'NONE', ( #65024 ), #8512, .T. ) ;
#36122=CARTESIAN_POINT ( 'NONE',  ( 17.49375000122903145, -2.886751345948074920, 5.000000000000092371 ) ) ;
#36124=CARTESIAN_POINT ( 'NONE',  ( 7.471875000614519813, -5.492252693125287522, -1.008910452111647106E-15 ) ) ;
#36131=CARTESIAN_POINT ( 'NONE',  ( 28.89375000122902648, -2.886751345948096237, -5.000000000000050626 ) ) ;
#36134=CARTESIAN_POINT ( 'NONE',  ( 15.54375000122903216, 5.773502691896255534, 3.535250795749688401E-16 ) ) ;
#36144=CARTESIAN_POINT ( 'NONE',  ( 14.14687500061451431, -4.119189519843965641, -2.378215178125001383 ) ) ;
#36147=CARTESIAN_POINT ( 'NONE',  ( 22.69687500061451502, -4.119189519843965641, -2.378215178125001383 ) ) ;
#36162=CARTESIAN_POINT ( 'NONE',  ( 24.68437500061451573, 5.824947211148865298E-16, -4.756430356249998326 ) ) ;
#36166=DIRECTION ( 'NONE',  ( -1.000000000000000000, -0.000000000000000000, -0.000000000000000000 ) ) ;
#36173=ORIENTED_EDGE ( 'NONE', *, *, #8082, .T. ) ;
#36182=CARTESIAN_POINT ( 'NONE',  ( 13.28437500061451715, -4.119189519843968306, 2.378215178124996054 ) ) ;
#36198=CARTESIAN_POINT ( 'NONE',  ( 25.33125000122903003, 6.123233995736764310E-16, -4.999999999999998224 ) ) ;
#36212=CARTESIAN_POINT ( 'NONE',  ( 13.73437500061451821, -4.119189519843968306, 2.378215178124996054 ) ) ;
#36215=VECTOR ( 'NONE', #68638, 1000.000000000000000 ) ;
#36220=CARTESIAN_POINT ( 'NONE',  ( 15.26249999999999929, -5.773502691896255534, -1.060575238724906372E-15 ) ) ;
#36224=CARTESIAN_POINT ( 'NONE',  ( 23.25937500061451857, 2.746126346562645981, -4.756430356249997438 ) ) ;
#36234=CARTESIAN_POINT ( 'NONE',  ( 21.53437500061451360, 5.492252693125287522, 3.363034840372157021E-16 ) ) ;
#36236=CARTESIAN_POINT ( 'NONE',  ( 9.946875000614516793, 0.000000000000000000, 4.756430356249998326 ) ) ;
#36247=CARTESIAN_POINT ( 'NONE',  ( 11.33437500061451431, -2.746126346562646425, 4.756430356249996549 ) ) ;
#36254=CARTESIAN_POINT ( 'NONE',  ( 23.69999999999999929, 0.000000000000000000, 4.999999999999998224 ) ) ;
#36258=ORIENTED_EDGE ( 'NONE', *, *, #21481, .F. ) ;
#36266=CARTESIAN_POINT ( 'NONE',  ( 29.77499999999999858, 6.123233995736764310E-16, -4.999999999999998224 ) ) ;
#36268=VECTOR ( 'NONE', #45294, 1000.000000000000000 ) ;
#36270=CARTESIAN_POINT ( 'NONE',  ( 19.54687500061451289, -2.746126346562646425, 4.756430356249996549 ) ) ;
#36304=CARTESIAN_POINT ( 'NONE',  ( 21.34687500061451715, -2.746126346562646425, 4.756430356249996549 ) ) ;
#36309=CARTESIAN_POINT ( 'NONE',  ( 23.85000000000000142, -4.330127018922190985, -2.500000000000001332 ) ) ;
#36314=DIRECTION ( 'NONE',  ( -1.000000000000000000, -0.000000000000000000, -0.000000000000000000 ) ) ;
#36320=CARTESIAN_POINT ( 'NONE',  ( 28.80937500061451217, 2.746126346562643317, 4.756430356249998326 ) ) ;
#36322=CARTESIAN_POINT ( 'NONE',  ( 15.64687500061451608, 4.119189519843966529, -2.378215178124998275 ) ) ;
#36335=CARTESIAN_POINT ( 'NONE',  ( 8.484375000614518214, 5.492252693125287522, 3.363034840372157021E-16 ) ) ;
#36343=DIRECTION ( 'NONE',  ( -1.000000000000000000, -0.000000000000000000, -0.000000000000000000 ) ) ;
#36345=CARTESIAN_POINT ( 'NONE',  ( 29.74687500061451573, 0.000000000000000000, 4.756430356249998326 ) ) ;
#36349=CARTESIAN_POINT ( 'NONE',  ( 7.800000000000001599, 4.330127018922192761, -2.499999999999997780 ) ) ;
#36356=CARTESIAN_POINT ( 'NONE',  ( 25.73437500061451644, 4.119189519843966529, 2.378215178124999607 ) ) ;
#36358=CARTESIAN_POINT ( 'NONE',  ( 10.65937500061451715, -4.119189519843965641, -2.378215178125001383 ) ) ;
#36373=CARTESIAN_POINT ( 'NONE',  ( 20.83125000122903359, 6.123233995736764310E-16, -4.999999999999998224 ) ) ;
#36381=CARTESIAN_POINT ( 'NONE',  ( 8.006250001229034297, 0.000000000000000000, 4.999999999999998224 ) ) ;
#36387=( BOUNDED_CURVE ( )  B_SPLINE_CURVE ( 2, ( #64197, #64931, #57924, #8416, #8784, #70110, #12866 ),
 .UNSPECIFIED., .F., .F. ) 
 B_SPLINE_CURVE_WITH_KNOTS ( ( 3, 2, 2, 3 ),
 ( 0.8000000000000000444, 0.8033333333333333437, 0.8066666666666666430, 0.8100000000000000533 ),
 .UNSPECIFIED. ) 
 CURVE ( )  GEOMETRIC_REPRESENTATION_ITEM ( )  RATIONAL_B_SPLINE_CURVE ( ( 1.000000000000000000, 0.8660254037844387076, 1.000000000000000000, 0.8660254037844387076, 1.000000000000000000, 0.8660254037844387076, 1.000000000000000000 ) ) 
 REPRESENTATION_ITEM ( '' )  );
#36396=ADVANCED_FACE ( 'NONE', ( #48778 ), #27338, .T. ) ;
#36423=EDGE_LOOP ( 'NONE', ( #38912, #32118, #66415, #52537 ) ) ;
#36426=CARTESIAN_POINT ( 'NONE',  ( 19.65000000000000213, 0.000000000000000000, 4.999999999999998224 ) ) ;
#36427=CARTESIAN_POINT ( 'NONE',  ( 17.70937500061451786, -5.492252693125287522, -1.008910452111647106E-15 ) ) ;
#36444=LINE ( 'NONE', #2461, #5639 ) ;
#36447=CARTESIAN_POINT ( 'NONE',  ( 16.62187500061451573, 2.746126346562645981, -4.756430356249997438 ) ) ;
#36458=EDGE_LOOP ( 'NONE', ( #48513, #11412, #39485, #43078 ) ) ;
#36464=CARTESIAN_POINT ( 'NONE',  ( 28.85625000122903216, -4.330127018922190985, -2.500000000000001332 ) ) ;
#36475=ORIENTED_EDGE ( 'NONE', *, *, #3065, .T. ) ;
#36487=CARTESIAN_POINT ( 'NONE',  ( 28.98750000000000071, 5.773502691896255534, 3.535250795749688894E-16 ) ) ;
#36493=CARTESIAN_POINT ( 'NONE',  ( 45.00000000000000000, 0.000000000000000000, 0.000000000000000000 ) ) ;
#36506=CARTESIAN_POINT ( 'NONE',  ( 14.82187500061451502, 4.119189519843966529, 2.378215178124999607 ) ) ;
#36509=CARTESIAN_POINT ( 'NONE',  ( 23.14687500061451786, -4.119189519843965641, -2.378215178125001383 ) ) ;
#36517=ADVANCED_FACE ( 'NONE', ( #61664 ), #55047, .T. ) ;
#36525=CARTESIAN_POINT ( 'NONE',  ( 24.79687500061451999, 5.492252693125287522, 3.363034840372157021E-16 ) ) ;
#36528=DIRECTION ( 'NONE',  ( -1.000000000000000000, -0.000000000000000000, -0.000000000000000000 ) ) ;
#36535=CARTESIAN_POINT ( 'NONE',  ( 7.218750001229033764, -5.773502691896255534, -1.060575238724906372E-15 ) ) ;
#36545=CARTESIAN_POINT ( 'NONE',  ( 12.64687500061451786, 5.492252693125287522, 3.363034840372157021E-16 ) ) ;
#36563=CARTESIAN_POINT ( 'NONE',  ( 14.98125000122903216, 6.123233995736764310E-16, -4.999999999999998224 ) ) ;
#36575=CARTESIAN_POINT ( 'NONE',  ( 14.89687500061451786, 5.492252693125287522, 3.363034840372157021E-16 ) ) ;
#36582=CARTESIAN_POINT ( 'NONE',  ( 15.90000000000000036, 4.330127018922192761, -2.499999999999997780 ) ) ;
#36594=CARTESIAN_POINT ( 'NONE',  ( 22.32187500061451502, 5.824947211148865298E-16, -4.756430356249998326 ) ) ;
#36596=CARTESIAN_POINT ( 'NONE',  ( 8.596875000614515372, 0.000000000000000000, 4.756430356249998326 ) ) ;
#36607=CARTESIAN_POINT ( 'NONE',  ( 9.909375000614517148, 2.746126346562643317, 4.756430356249998326 ) ) ;
#36629=CARTESIAN_POINT ( 'NONE',  ( 18.94687500061451857, 5.492252693125287522, 3.363034840372157021E-16 ) ) ;
#36642=EDGE_LOOP ( 'NONE', ( #51254, #31155, #33720, #34150 ) ) ;
#36648=CARTESIAN_POINT ( 'NONE',  ( 20.38125000122903430, 6.123233995736764310E-16, -4.999999999999998224 ) ) ;
#36663=CARTESIAN_POINT ( 'NONE',  ( 21.00937500061451857, -4.119189519843965641, -2.378215178125001383 ) ) ;
#36669=CARTESIAN_POINT ( 'NONE',  ( 22.98749999999999716, -2.886751345948125991, -5.000000000000000000 ) ) ;
#36671=CARTESIAN_POINT ( 'NONE',  ( 9.262499999999997513, 2.886751345948182834, 4.999999999999902300 ) ) ;
#36672=CARTESIAN_POINT ( 'NONE',  ( 45.00000000000000000, 0.000000000000000000, 4.999999999999998224 ) ) ;
#36679=CARTESIAN_POINT ( 'NONE',  ( 28.50937500061451857, -5.492252693125287522, -1.008910452111647106E-15 ) ) ;
#36681=CARTESIAN_POINT ( 'NONE',  ( 14.85937500061451999, 2.746126346562643317, 4.756430356249998326 ) ) ;
#36691=CARTESIAN_POINT ( 'NONE',  ( 7.471875000614514484, 5.824947211148865298E-16, -4.756430356249998326 ) ) ;
#36702=CARTESIAN_POINT ( 'NONE',  ( 28.47187500061451715, -4.119189519843968306, 2.378215178124996054 ) ) ;
#36703=ORIENTED_EDGE ( 'NONE', *, *, #1145, .T. ) ;
#36706=CARTESIAN_POINT ( 'NONE',  ( 8.362500000000002487, 2.886751345948126879, 4.999999999999999112 ) ) ;
#36713=CARTESIAN_POINT ( 'NONE',  ( 27.23437500061451644, -4.119189519843968306, 2.378215178124996054 ) ) ;
#36715=CARTESIAN_POINT ( 'NONE',  ( 10.35937500061451644, 4.119189519843966529, -2.378215178124998275 ) ) ;
#36733=CARTESIAN_POINT ( 'NONE',  ( 20.64375000122903359, -2.886751345948129988, 4.999999999999997335 ) ) ;
#36734=VECTOR ( 'NONE', #38049, 1000.000000000000227 ) ;
#36736=DIRECTION ( 'NONE',  ( -1.000000000000000000, -0.000000000000000000, -0.000000000000000000 ) ) ;
#36750=CARTESIAN_POINT ( 'NONE',  ( 28.28437500061451715, 5.824947211148865298E-16, -4.756430356249998326 ) ) ;
#36777=DIRECTION ( 'NONE',  ( -1.000000000000000000, -0.000000000000000000, -0.000000000000000000 ) ) ;
#36781=ORIENTED_EDGE ( 'NONE', *, *, #23281, .T. ) ;
#36786=DIRECTION ( 'NONE',  ( -0.000000000000000000, -0.000000000000000000, -1.000000000000000000 ) ) ;
#36789=CARTESIAN_POINT ( 'NONE',  ( 17.07187500061451502, 4.119189519843966529, 2.378215178124999607 ) ) ;
#36804=CARTESIAN_POINT ( 'NONE',  ( 25.81875000122903430, 2.886751345948157077, -4.999999999999949374 ) ) ;
#36805=CARTESIAN_POINT ( 'NONE',  ( 9.618750001229033231, 2.886751345948129099, -4.999999999999997335 ) ) ;
#36808=CARTESIAN_POINT ( 'NONE',  ( 17.40937500061451715, -4.119189519843965641, -2.378215178125001383 ) ) ;
#36819=DIRECTION ( 'NONE',  ( -1.000000000000000000, -0.000000000000000000, -0.000000000000000000 ) ) ;
#36820=VERTEX_POINT ( 'NONE', #54677 ) ;
#36828=CARTESIAN_POINT ( 'NONE',  ( 28.74375000122903501, -2.886751345948129988, 4.999999999999997335 ) ) ;
#36851=CARTESIAN_POINT ( 'NONE',  ( 28.68749999999999645, -2.886751345948129988, 4.999999999999997335 ) ) ;
#36857=CARTESIAN_POINT ( 'NONE',  ( 27.29999999999999716, 0.000000000000000000, 4.999999999999998224 ) ) ;
#36859=VECTOR ( 'NONE', #71150, 1000.000000000000000 ) ;
#36870=CARTESIAN_POINT ( 'NONE',  ( 14.55937500061451750, -5.492252693125287522, -1.008910452111647106E-15 ) ) ;
#36873=CARTESIAN_POINT ( 'NONE',  ( 23.40937500061451715, 2.746126346562643317, 4.756430356249998326 ) ) ;
#36878=CARTESIAN_POINT ( 'NONE',  ( 24.07499999999999929, 4.330127018922191873, 2.499999999999999556 ) ) ;
#36883=CARTESIAN_POINT ( 'NONE',  ( 23.60625000122903216, 4.330127018922192761, -2.499999999999997780 ) ) ;
#36884=CARTESIAN_POINT ( 'NONE',  ( 12.78749999999999964, 5.773502691896255534, 3.535250795749688894E-16 ) ) ;
#36891=CARTESIAN_POINT ( 'NONE',  ( 25.35937500061451644, 0.000000000000000000, 4.756430356249998326 ) ) ;
#36894=EDGE_CURVE ( 'NONE', #55926, #33907, #6582, .T. ) ;
#36901=DIRECTION ( 'NONE',  ( -1.000000000000000000, -0.000000000000000000, -0.000000000000000000 ) ) ;
#36911=CARTESIAN_POINT ( 'NONE',  ( 11.70937500061451608, 4.119189519843966529, -2.378215178124998275 ) ) ;
#36914=CARTESIAN_POINT ( 'NONE',  ( 7.593750001229034652, -2.886751345948130876, 4.999999999999996447 ) ) ;
#36940=CARTESIAN_POINT ( 'NONE',  ( 13.09687500061451892, 5.492252693125287522, 3.363034840372157021E-16 ) ) ;
#36943=CARTESIAN_POINT ( 'NONE',  ( 21.95625000122903003, 0.000000000000000000, 4.999999999999998224 ) ) ;
#36948=CARTESIAN_POINT ( 'NONE',  ( 15.45000000000000107, 4.330127018922192761, -2.499999999999997780 ) ) ;
#36959=CARTESIAN_POINT ( 'NONE',  ( 22.47187500061451360, 4.119189519843966529, 2.378215178124999607 ) ) ;
#36961=CARTESIAN_POINT ( 'NONE',  ( 9.309375000614517504, 2.746126346562645981, -4.756430356249997438 ) ) ;
#36971=CARTESIAN_POINT ( 'NONE',  ( 8.559375000614515727, 2.746126346562643317, 4.756430356249998326 ) ) ;
#36974=EDGE_CURVE ( 'NONE', #38724, #60669, #49511, .T. ) ;
#36991=CARTESIAN_POINT ( 'NONE',  ( 14.19375000122903252, 5.773502691896255534, 3.535250795749688401E-16 ) ) ;
#36994=CARTESIAN_POINT ( 'NONE',  ( 18.83437500061451431, 5.824947211148865298E-16, -4.756430356249998326 ) ) ;
#37001=( BOUNDED_CURVE ( )  B_SPLINE_CURVE ( 2, ( #38603, #44523, #61487, #27887, #66680, #67056, #49325 ),
 .UNSPECIFIED., .F., .F. ) 
 B_SPLINE_CURVE_WITH_KNOTS ( ( 3, 2, 2, 3 ),
 ( 0.9400000000000001688, 0.9433333333333335791, 0.9466666666666667673, 0.9500000000000000666 ),
 .UNSPECIFIED. ) 
 CURVE ( )  GEOMETRIC_REPRESENTATION_ITEM ( )  RATIONAL_B_SPLINE_CURVE ( ( 0.9999999999999911182, 0.8660254037844475894, 1.000000000000000000, 0.8660254037844387076, 1.000000000000000000, 0.8660254037844342667, 1.000000000000004441 ) ) 
 REPRESENTATION_ITEM ( '' )  );
#37022=ORIENTED_EDGE ( 'NONE', *, *, #8224, .F. ) ;
#37026=CARTESIAN_POINT ( 'NONE',  ( 20.22187500061451715, 2.746126346562645981, -4.756430356249997438 ) ) ;
#37028=EDGE_CURVE ( 'NONE', #28470, #28191, #6147, .T. ) ;
#37033=CARTESIAN_POINT ( 'NONE',  ( 23.21250000000000213, 2.886751345948126879, 4.999999999999999112 ) ) ;
#37039=CARTESIAN_POINT ( 'NONE',  ( 19.48125000122903216, 6.123233995736764310E-16, -4.999999999999998224 ) ) ;
#37043=CARTESIAN_POINT ( 'NONE',  ( 28.77187500061451431, 4.119189519843966529, 2.378215178124999607 ) ) ;
#37045=CARTESIAN_POINT ( 'NONE',  ( 15.79687500061451644, 0.000000000000000000, 4.756430356249998326 ) ) ;
#37061=ORIENTED_EDGE ( 'NONE', *, *, #55693, .F. ) ;
#37067=CARTESIAN_POINT ( 'NONE',  ( 29.25937500061451857, 2.746126346562643317, 4.756430356249998326 ) ) ;
#37068=VECTOR ( 'NONE', #63473, 1000.000000000000000 ) ;
#37072=CARTESIAN_POINT ( 'NONE',  ( 25.78125000122903288, 6.123233995736764310E-16, -4.999999999999998224 ) ) ;
#37079=CARTESIAN_POINT ( 'NONE',  ( 26.40937500061451715, -4.119189519843965641, -2.378215178125001383 ) ) ;
#37081=CARTESIAN_POINT ( 'NONE',  ( 11.52187500061451608, -5.492252693125287522, -1.008910452111647106E-15 ) ) ;
#37097=CARTESIAN_POINT ( 'NONE',  ( 21.50625000122903074, 0.000000000000000000, 4.999999999999998224 ) ) ;
#37105=CARTESIAN_POINT ( 'NONE',  ( 23.08125000122903359, 6.123233995736764310E-16, -4.999999999999998224 ) ) ;
#37112=CARTESIAN_POINT ( 'NONE',  ( 27.30937500061451573, -4.119189519843965641, -2.378215178125001383 ) ) ;
#37125=VECTOR ( 'NONE', #37251, 1000.000000000000000 ) ;
#37135=ORIENTED_EDGE ( 'NONE', *, *, #20329, .T. ) ;
#37149=ORIENTED_EDGE ( 'NONE', *, *, #23556, .T. ) ;
#37150=CARTESIAN_POINT ( 'NONE',  ( 11.77500000000000036, 6.123233995736764310E-16, -4.999999999999998224 ) ) ;
#37153=CARTESIAN_POINT ( 'NONE',  ( 15.83437500061451253, -2.746126346562646425, 4.756430356249996549 ) ) ;
#37160=DIRECTION ( 'NONE',  ( -1.000000000000000000, -0.000000000000000000, -0.000000000000000000 ) ) ;
#37168=CARTESIAN_POINT ( 'NONE',  ( 45.00000000000000000, 0.000000000000000000, 4.999999999999998224 ) ) ;
#37172=CARTESIAN_POINT ( 'NONE',  ( 17.48437500061451999, 5.824947211148865298E-16, -4.756430356249998326 ) ) ;
#37183=DIRECTION ( 'NONE',  ( 0.000000000000000000, 0.000000000000000000, 1.000000000000000000 ) ) ;
#37191=CARTESIAN_POINT ( 'NONE',  ( 27.76875000122903003, 2.886751345948126879, 4.999999999999999112 ) ) ;
#37193=CARTESIAN_POINT ( 'NONE',  ( 26.68125000122903145, 6.123233995736764310E-16, -4.999999999999998224 ) ) ;
#37196=CARTESIAN_POINT ( 'NONE',  ( -5.000000000000004441, 0.000000000000000000, 4.999999999999998224 ) ) ;
#37206=DIRECTION ( 'NONE',  ( 0.000000000000000000, 0.000000000000000000, 1.000000000000000000 ) ) ;
#37217=CYLINDRICAL_SURFACE ( 'NONE', #11220, 4.999999999999998224 ) ;
#37218=CARTESIAN_POINT ( 'NONE',  ( 29.09999999999999787, 0.000000000000000000, 4.999999999999998224 ) ) ;
#37227=VECTOR ( 'NONE', #43181, 1000.000000000000000 ) ;
#37238=CARTESIAN_POINT ( 'NONE',  ( 16.05937500061451573, 2.746126346562645981, -4.756430356249997438 ) ) ;
#37242=CARTESIAN_POINT ( 'NONE',  ( 24.90937500061451004, -5.492252693125287522, -1.008910452111647106E-15 ) ) ;
#37247=CARTESIAN_POINT ( 'NONE',  ( 15.48749999999999893, 5.773502691896255534, 3.535250795749688401E-16 ) ) ;
#37251=DIRECTION ( 'NONE',  ( 0.000000000000000000, 1.000000000000000000, -8.673617379884036705E-17 ) ) ;
#37252=CARTESIAN_POINT ( 'NONE',  ( 12.71250000000000036, 2.886751345948129099, -4.999999999999998224 ) ) ;
#37259=CARTESIAN_POINT ( 'NONE',  ( 25.77187500061451075, 2.746126346562643317, 4.756430356249998326 ) ) ;
#37263=CARTESIAN_POINT ( 'NONE',  ( 15.20625000122903181, 0.000000000000000000, 4.999999999999998224 ) ) ;
#37269=CARTESIAN_POINT ( 'NONE',  ( 7.331250001229031810, 6.123233995736764310E-16, -4.999999999999998224 ) ) ;
#37280=CARTESIAN_POINT ( 'NONE',  ( 10.02187500061451964, 2.746126346562643317, 4.756430356249998326 ) ) ;
#37292=CARTESIAN_POINT ( 'NONE',  ( 23.34375000122902577, -2.886751345948130876, 4.999999999999996447 ) ) ;
#37309=CARTESIAN_POINT ( 'NONE',  ( 12.94687500061451857, -2.746126346562642428, -4.756430356249999214 ) ) ;
#37312=CARTESIAN_POINT ( 'NONE',  ( 13.40625000122903288, 0.000000000000000000, 4.999999999999998224 ) ) ;
#37317=CARTESIAN_POINT ( 'NONE',  ( 15.67500000000000071, -4.330127018922194537, 2.499999999999995559 ) ) ;
#37330=CARTESIAN_POINT ( 'NONE',  ( 22.62187500061451573, -4.119189519843968306, 2.378215178124996054 ) ) ;
#37332=CARTESIAN_POINT ( 'NONE',  ( 9.384375000614515017, 5.492252693125287522, 3.363034840372157021E-16 ) ) ;
#37344=CARTESIAN_POINT ( 'NONE',  ( 9.646875000614514306, -4.119189519843965641, -2.378215178125001383 ) ) ;
#37367=CARTESIAN_POINT ( 'NONE',  ( 19.88437500061451857, 4.119189519843966529, 2.378215178124999607 ) ) ;
#37382=AXIS2_PLACEMENT_3D ( 'NONE', #25819, #64603, #71621 ) ;
#37398=CARTESIAN_POINT ( 'NONE',  ( 19.99687500061451573, -2.746126346562646425, 4.756430356249996549 ) ) ;
#37405=CARTESIAN_POINT ( 'NONE',  ( 21.18749999999999645, -2.886751345948125991, -5.000000000000000000 ) ) ;
#37412=CARTESIAN_POINT ( 'NONE',  ( 29.60625000122903216, 0.000000000000000000, 4.999999999999998224 ) ) ;
#37416=CARTESIAN_POINT ( 'NONE',  ( 29.37187500061451573, -4.119189519843968306, 2.378215178124996054 ) ) ;
#37418=CARTESIAN_POINT ( 'NONE',  ( 17.14687500061451431, 0.000000000000000000, 4.756430356249998326 ) ) ;
#37453=CARTESIAN_POINT ( 'NONE',  ( 26.18437500061451573, 4.119189519843966529, 2.378215178124999607 ) ) ;
#37455=CARTESIAN_POINT ( 'NONE',  ( 8.971875000614515372, 2.746126346562645981, -4.756430356249997438 ) ) ;
#37471=CARTESIAN_POINT ( 'NONE',  ( 21.09375000122903288, -2.886751345948129988, 4.999999999999997335 ) ) ;
#37473=CARTESIAN_POINT ( 'NONE',  ( 21.39375000122903359, 5.773502691896255534, 3.535250795749688401E-16 ) ) ;
#37479=CARTESIAN_POINT ( 'NONE',  ( 45.00000000000000000, 0.000000000000000000, 4.999999999999998224 ) ) ;
#37486=CARTESIAN_POINT ( 'NONE',  ( 28.80937500061451573, 4.119189519843966529, -2.378215178124998275 ) ) ;
#37494=CARTESIAN_POINT ( 'NONE',  ( 22.10625000122903216, -4.330127018922190985, -2.500000000000001332 ) ) ;
#37515=ORIENTED_EDGE ( 'NONE', *, *, #35397, .F. ) ;
#37522=CARTESIAN_POINT ( 'NONE',  ( 13.58437500061451431, -2.746126346562646425, 4.756430356249996549 ) ) ;
#37535=CARTESIAN_POINT ( 'NONE',  ( 16.50000000000000000, 0.000000000000000000, 4.999999999999998224 ) ) ;
#37536=CARTESIAN_POINT ( 'NONE',  ( 14.21249999999999858, 2.886751345948238789, 4.999999999999807265 ) ) ;
#37539=CARTESIAN_POINT ( 'NONE',  ( 8.606250001229033941, -4.330127018922190985, -2.500000000000001332 ) ) ;
#37540=CARTESIAN_POINT ( 'NONE',  ( 18.57187500061451857, 2.746126346562643317, 4.756430356249998326 ) ) ;
#37557=CARTESIAN_POINT ( 'NONE',  ( 29.00625000122903074, 4.330127018922192761, -2.499999999999997780 ) ) ;
#37583=CARTESIAN_POINT ( 'NONE',  ( 27.26249999999999929, 2.886751345948126879, 4.999999999999999112 ) ) ;
#37585=CARTESIAN_POINT ( 'NONE',  ( 26.64375000122903003, -2.886751345948139758, -4.999999999999975131 ) ) ;
#37594=CARTESIAN_POINT ( 'NONE',  ( 27.43125000122903145, -4.330127018922194537, 2.499999999999995559 ) ) ;
#37605=CARTESIAN_POINT ( 'NONE',  ( 20.33437500061451786, -2.746126346562646425, 4.756430356249996549 ) ) ;
#37609=CARTESIAN_POINT ( 'NONE',  ( 15.56249999999999467, 2.886751345948182834, 4.999999999999902300 ) ) ;
#37613=DIRECTION ( 'NONE',  ( 0.000000000000000000, 0.000000000000000000, 1.000000000000000000 ) ) ;
#37614=CARTESIAN_POINT ( 'NONE',  ( 13.38750000000000107, -2.886751345948129988, 4.999999999999997335 ) ) ;
#37621=CARTESIAN_POINT ( 'NONE',  ( 24.23437500061451644, 5.824947211148865298E-16, -4.756430356249998326 ) ) ;
#37641=CARTESIAN_POINT ( 'NONE',  ( 10.50937500061451679, 0.000000000000000000, 4.756430356249998326 ) ) ;
#37653=ORIENTED_EDGE ( 'NONE', *, *, #32494, .F. ) ;
#37665=ORIENTED_EDGE ( 'NONE', *, *, #57573, .F. ) ;
#37669=CARTESIAN_POINT ( 'NONE',  ( 15.00937500061451679, 0.000000000000000000, 4.756430356249998326 ) ) ;
#37679=CARTESIAN_POINT ( 'NONE',  ( 45.00000000000000000, 0.000000000000000000, 0.000000000000000000 ) ) ;
#37683=CARTESIAN_POINT ( 'NONE',  ( 20.04375000122902861, 5.773502691896255534, 3.535250795749688401E-16 ) ) ;
#37685=CARTESIAN_POINT ( 'NONE',  ( 7.176562500921773946, 0.000000000000000000, 4.878215178124998275 ) ) ;
#37687=CARTESIAN_POINT ( 'NONE',  ( 21.08437500061451786, 5.492252693125287522, 3.363034840372157021E-16 ) ) ;
#37694=CARTESIAN_POINT ( 'NONE',  ( 16.10625000122903216, 0.000000000000000000, 4.999999999999998224 ) ) ;
#37702=CARTESIAN_POINT ( 'NONE',  ( 9.571875000614515017, -4.119189519843968306, 2.378215178124996054 ) ) ;
#37726=CARTESIAN_POINT ( 'NONE',  ( 15.98437500061451821, -4.119189519843968306, 2.378215178124996054 ) ) ;
#37747=CARTESIAN_POINT ( 'NONE',  ( 20.56875000122903785, 2.886751345948154857, 4.999999999999951150 ) ) ;
#37753=CARTESIAN_POINT ( 'NONE',  ( 23.92499999999999716, 6.123233995736764310E-16, -4.999999999999998224 ) ) ;
#37760=CARTESIAN_POINT ( 'NONE',  ( 22.13437500061451502, 4.119189519843966529, 2.378215178124999607 ) ) ;
#37766=CARTESIAN_POINT ( 'NONE',  ( 22.05000000000000071, -4.330127018922190985, -2.500000000000001332 ) ) ;
#37770=CARTESIAN_POINT ( 'NONE',  ( 18.46875000122902932, -5.773502691896255534, -1.060575238724906372E-15 ) ) ;
#37776=CARTESIAN_POINT ( 'NONE',  ( 28.95937500061451075, -5.492252693125287522, -1.008910452111647106E-15 ) ) ;
#37778=CARTESIAN_POINT ( 'NONE',  ( 13.65937500061451537, -5.492252693125287522, -1.008910452111647106E-15 ) ) ;
#37781=EDGE_LOOP ( 'NONE', ( #49342, #13419, #72321, #23749 ) ) ;
#37785=CARTESIAN_POINT ( 'NONE',  ( 26.06250000000000000, -5.773502691896255534, -1.060575238724906372E-15 ) ) ;
#37788=LINE ( 'NONE', #60308, #41940 ) ;
#37789=CARTESIAN_POINT ( 'NONE',  ( 8.634375000614515017, -2.746126346562646425, 4.756430356249996549 ) ) ;
#37794=EDGE_CURVE ( 'NONE', #32613, #26559, #72166, .T. ) ;
#37802=ORIENTED_EDGE ( 'NONE', *, *, #8067, .T. ) ;
#37813=CARTESIAN_POINT ( 'NONE',  ( 24.49687500061451573, -2.746126346562646425, 4.756430356249996549 ) ) ;
#37832=CARTESIAN_POINT ( 'NONE',  ( 17.53125000122903288, -4.330127018922194537, 2.499999999999995559 ) ) ;
#37840=CARTESIAN_POINT ( 'NONE',  ( 20.77500000000000213, 6.123233995736764310E-16, -4.999999999999998224 ) ) ;
#37847=CARTESIAN_POINT ( 'NONE',  ( 28.20937500061451786, -4.119189519843965641, -2.378215178125001383 ) ) ;
#37850=( BOUNDED_CURVE ( )  B_SPLINE_CURVE ( 2, ( #11380, #21723, #61978, #34257, #56790, #33535, #44652 ),
 .UNSPECIFIED., .F., .F. ) 
 B_SPLINE_CURVE_WITH_KNOTS ( ( 3, 2, 2, 3 ),
 ( 0.4300000000000001044, 0.4333333333333334036, 0.4366666666666667029, 0.4400000000000000022 ),
 .UNSPECIFIED. ) 
 CURVE ( )  GEOMETRIC_REPRESENTATION_ITEM ( )  RATIONAL_B_SPLINE_CURVE ( ( 0.9999999999999955591, 0.8660254037844431485, 1.000000000000000000, 0.8660254037844387076, 1.000000000000000000, 0.8660254037844387076, 1.000000000000000000 ) ) 
 REPRESENTATION_ITEM ( '' )  );
#37851=EDGE_CURVE ( 'NONE', #52599, #67375, #38704, .T. ) ;
#37856=CARTESIAN_POINT ( 'NONE',  ( 22.03125000122903288, -4.330127018922194537, 2.499999999999995559 ) ) ;
#37868=CARTESIAN_POINT ( 'NONE',  ( 20.22187500061451715, 4.119189519843966529, 2.378215178124999607 ) ) ;
#37871=ORIENTED_EDGE ( 'NONE', *, *, #27156, .T. ) ;
#37885=CARTESIAN_POINT ( 'NONE',  ( 14.97187500061451537, -4.119189519843968306, 2.378215178124996054 ) ) ;
#37901=CARTESIAN_POINT ( 'NONE',  ( 15.39375000122903359, -2.886751345948126435, -5.000000000000000000 ) ) ;
#37902=CARTESIAN_POINT ( 'NONE',  ( 24.37500000000000000, 6.123233995736764310E-16, -4.999999999999998224 ) ) ;
#37906=CARTESIAN_POINT ( 'NONE',  ( 14.18437500061451750, -4.119189519843968306, 2.378215178124996054 ) ) ;
#37924=CARTESIAN_POINT ( 'NONE',  ( 25.29375000122902861, -2.886751345948125991, -5.000000000000000000 ) ) ;
#37958=CARTESIAN_POINT ( 'NONE',  ( 27.46875000122902577, -5.773502691896255534, -1.060575238724906372E-15 ) ) ;
#37967=VERTEX_POINT ( 'NONE', #51957 ) ;
#37970=CARTESIAN_POINT ( 'NONE',  ( 20.18437500061451217, 5.492252693125287522, 3.363034840372157021E-16 ) ) ;
#37974=CARTESIAN_POINT ( 'NONE',  ( 24.11250000000000071, 2.886751345948154857, 4.999999999999951150 ) ) ;
#37979=CARTESIAN_POINT ( 'NONE',  ( 13.61250000000000071, 2.886751345948129099, -4.999999999999998224 ) ) ;
#37986=CARTESIAN_POINT ( 'NONE',  ( 22.09687500061451715, 5.492252693125287522, 3.363034840372157021E-16 ) ) ;
#37990=DIRECTION ( 'NONE',  ( 0.000000000000000000, 0.000000000000000000, 1.000000000000000000 ) ) ;
#38004=CARTESIAN_POINT ( 'NONE',  ( 28.51875000122903359, 2.886751345948104674, -5.000000000000039968 ) ) ;
#38009=CARTESIAN_POINT ( 'NONE',  ( 10.47187500061451715, 2.746126346562643317, 4.756430356249998326 ) ) ;
#38019=ORIENTED_EDGE ( 'NONE', *, *, #5554, .F. ) ;
#38028=( BOUNDED_CURVE ( )  B_SPLINE_CURVE ( 2, ( #54044, #36671, #25593, #3440, #70296, #19667, #25959 ),
 .UNSPECIFIED., .F., .F. ) 
 B_SPLINE_CURVE_WITH_KNOTS ( ( 3, 2, 2, 3 ),
 ( 0.9200000000000001510, 0.9233333333333334503, 0.9266666666666667496, 0.9300000000000001599 ),
 .UNSPECIFIED. ) 
 CURVE ( )  GEOMETRIC_REPRESENTATION_ITEM ( )  RATIONAL_B_SPLINE_CURVE ( ( 0.9999999999999955591, 0.8660254037844431485, 1.000000000000000000, 0.8660254037844387076, 1.000000000000000000, 0.8660254037844342667, 1.000000000000004441 ) ) 
 REPRESENTATION_ITEM ( '' )  );
#38034=CARTESIAN_POINT ( 'NONE',  ( 11.29687500061451644, 5.492252693125287522, 3.363034840372157021E-16 ) ) ;
#38035=FACE_OUTER_BOUND ( 'NONE', #17430, .T. ) ;
#38046=CARTESIAN_POINT ( 'NONE',  ( 19.57500000000000284, 4.330127018922191873, 2.499999999999999556 ) ) ;
#38049=DIRECTION ( 'NONE',  ( -0.4999999999999975575, -0.000000000000000000, 0.8660254037844400399 ) ) ;
#38052=CARTESIAN_POINT ( 'NONE',  ( 21.00937500061451857, 2.746126346562645981, -4.756430356249997438 ) ) ;
#38055=CARTESIAN_POINT ( 'NONE',  ( 14.00625000122903252, -4.330127018922190985, -2.500000000000001332 ) ) ;
#38069=CARTESIAN_POINT ( 'NONE',  ( 28.84687500061452070, 5.492252693125287522, 3.363034840372157021E-16 ) ) ;
#38073=( BOUNDED_CURVE ( )  B_SPLINE_CURVE ( 2, ( #18779, #35066, #40986, #12889, #23971, #35782, #6995 ),
 .UNSPECIFIED., .F., .F. ) 
 B_SPLINE_CURVE_WITH_KNOTS ( ( 3, 2, 2, 3 ),
 ( 0.3400000000000000799, 0.3433333333333333792, 0.3466666666666667895, 0.3500000000000000888 ),
 .UNSPECIFIED. ) 
 CURVE ( )  GEOMETRIC_REPRESENTATION_ITEM ( )  RATIONAL_B_SPLINE_CURVE ( ( 0.9999999999999977796, 0.8660254037844409281, 1.000000000000000000, 0.8660254037844387076, 1.000000000000000000, 0.8660254037844342667, 1.000000000000004441 ) ) 
 REPRESENTATION_ITEM ( '' )  );
#38091=CARTESIAN_POINT ( 'NONE',  ( 17.48437500061451999, 5.824947211148865298E-16, -4.756430356249998326 ) ) ;
#38106=ORIENTED_EDGE ( 'NONE', *, *, #42868, .F. ) ;
#38121=VERTEX_POINT ( 'NONE', #22777 ) ;
#38124=CARTESIAN_POINT ( 'NONE',  ( 18.49687500061452283, 5.492252693125287522, 3.363034840372157021E-16 ) ) ;
#38130=CARTESIAN_POINT ( 'NONE',  ( 21.75000000000000000, 4.330127018922192761, -2.499999999999997780 ) ) ;
#38140=CARTESIAN_POINT ( 'NONE',  ( 26.52187500061451431, 4.119189519843966529, 2.378215178124999607 ) ) ;
#38142=CARTESIAN_POINT ( 'NONE',  ( 13.17187500061451466, -4.119189519843968306, 2.378215178124996054 ) ) ;
#38168=CARTESIAN_POINT ( 'NONE',  ( 29.51249999999999929, 2.886751345948106007, 5.000000000000033751 ) ) ;
#38175=CARTESIAN_POINT ( 'NONE',  ( 25.35937500061451644, 0.000000000000000000, 4.756430356249998326 ) ) ;
#38194=CARTESIAN_POINT ( 'NONE',  ( 19.10625000122903216, 4.330127018922192761, -2.499999999999997780 ) ) ;
#38203=CARTESIAN_POINT ( 'NONE',  ( 20.81249999999999645, 2.886751345948157077, -4.999999999999949374 ) ) ;
#38210=CARTESIAN_POINT ( 'NONE',  ( 24.94687500061451502, -2.746126346562646425, 4.756430356249996549 ) ) ;
#38225=CARTESIAN_POINT ( 'NONE',  ( 12.01875000122903181, 2.886751345948126879, 4.999999999999999112 ) ) ;
#38226=CARTESIAN_POINT ( 'NONE',  ( 13.35000000000000142, 0.000000000000000000, 4.999999999999998224 ) ) ;
#38229=CARTESIAN_POINT ( 'NONE',  ( 20.74687500061451217, 0.000000000000000000, 4.756430356249998326 ) ) ;
#38230=VECTOR ( 'NONE', #33492, 1000.000000000000000 ) ;
#38234=CARTESIAN_POINT ( 'NONE',  ( 10.70625000122903536, 0.000000000000000000, 4.999999999999998224 ) ) ;
#38244=ORIENTED_EDGE ( 'NONE', *, *, #69367, .F. ) ;
#38247=CARTESIAN_POINT ( 'NONE',  ( 12.30000000000000249, 4.330127018922192761, -2.499999999999997780 ) ) ;
#38248=CARTESIAN_POINT ( 'NONE',  ( 13.13437500061451679, -2.746126346562646425, 4.756430356249996549 ) ) ;
#38255=ORIENTED_EDGE ( 'NONE', *, *, #13474, .T. ) ;
#38258=CARTESIAN_POINT ( 'NONE',  ( 17.00625000122903074, 0.000000000000000000, 4.999999999999998224 ) ) ;
#38266=LINE ( 'NONE', #26094, #47788 ) ;
#38267=CARTESIAN_POINT ( 'NONE',  ( 14.37187500061451928, 2.746126346562645981, -4.756430356249997438 ) ) ;
#38277=CARTESIAN_POINT ( 'NONE',  ( 12.93750000000000178, -2.886751345948130876, 4.999999999999996447 ) ) ;
#38280=CARTESIAN_POINT ( 'NONE',  ( 28.70625000122903003, 0.000000000000000000, 4.999999999999998224 ) ) ;
#38284=CARTESIAN_POINT ( 'NONE',  ( 26.98125000122903216, -4.330127018922194537, 2.499999999999995559 ) ) ;
#38287=( BOUNDED_CURVE ( )  B_SPLINE_CURVE ( 2, ( #41313, #35032, #63471, #6963, #1797, #24307, #46854 ),
 .UNSPECIFIED., .F., .F. ) 
 B_SPLINE_CURVE_WITH_KNOTS ( ( 3, 2, 2, 3 ),
 ( 0.07000000000000000666, 0.07333333333333333370, 0.07666666666666664687, 0.07999999999999998779 ),
 .UNSPECIFIED. ) 
 CURVE ( )  GEOMETRIC_REPRESENTATION_ITEM ( )  RATIONAL_B_SPLINE_CURVE ( ( 1.000000000000000000, 0.8660254037844387076, 1.000000000000000000, 0.8660254037844387076, 1.000000000000000000, 0.8660254037844392627, 0.9999999999999994449 ) ) 
 REPRESENTATION_ITEM ( '' )  );
#38295=VECTOR ( 'NONE', #7873, 1000.000000000000000 ) ;
#38304=CLOSED_SHELL ( 'NONE', ( #2216, #48570, #64448, #6708, #20115, #50433, #8046, #28701, #58821, #58549, #46169, #50768, #15966, #72319, #71451, #52232, #11530, #5648, #63632, #36115, #68116, #44592, #8217, #938, #40897, #9715, #18812, #38595, #7613, #67122, #65303, #48014, #1343, #21552, #1345, #31744, #26322, #29765, #18778, #12039, #31479, #67767, #63978, #42410, #69023, #63739, #5062, #45529, #63989, #63916, #58073, #13339, #30169, #9477, #58970, #24046, #56340, #26141, #28884, #36517, #68685, #34396, #20596, #10857, #53442, #10366, #8427, #70238, #47871, #18911, #56194, #63573, #11058, #6771, #36396, #3882, #34249, #39935, #43142, #21784, #32588, #43797, #59626, #4259, #38917, #70188, #46405, #64940, #49491, #59332, #53414, #31611, #8789, #54092, #11967, #35596, #8710, #58147, #27806, #12217, #43240, #46440, #59400, #26635, #22141, #30413, #30589, #13175, #14823, #15303, #61928, #13081, #52220, #72490, #41168 ) ) ;
#38309=AXIS2_PLACEMENT_3D ( 'NONE', #61700, #72800, #44001 ) ;
#38317=EDGE_CURVE ( 'NONE', #18378, #1784, #33867, .T. ) ;
#38336=CARTESIAN_POINT ( 'NONE',  ( 22.50937500061451502, 2.746126346562643317, 4.756430356249998326 ) ) ;
#38345=ORIENTED_EDGE ( 'NONE', *, *, #36974, .T. ) ;
#38346=CARTESIAN_POINT ( 'NONE',  ( 12.33750000000000036, 5.773502691896255534, 3.535250795749688894E-16 ) ) ;
#38348=VECTOR ( 'NONE', #33593, 1000.000000000000000 ) ;
#38354=CARTESIAN_POINT ( 'NONE',  ( 22.58437500061451431, 4.119189519843966529, 2.378215178124999607 ) ) ;
#38362=AXIS2_PLACEMENT_3D ( 'NONE', #69373, #8028, #57172 ) ;
#38365=DIRECTION ( 'NONE',  ( -1.000000000000000000, -0.000000000000000000, -0.000000000000000000 ) ) ;
#38368=VECTOR ( 'NONE', #9101, 1000.000000000000000 ) ;
#38379=CARTESIAN_POINT ( 'NONE',  ( 10.05937500061451750, 0.000000000000000000, 4.756430356249998326 ) ) ;
#38402=AXIS2_PLACEMENT_3D ( 'NONE', #16902, #28016, #16185 ) ;
#38403=CARTESIAN_POINT ( 'NONE',  ( 10.80937500061451928, 4.119189519843966529, -2.378215178124998275 ) ) ;
#38410=VECTOR ( 'NONE', #23249, 1000.000000000000000 ) ;
#38415=DIRECTION ( 'NONE',  ( 0.000000000000000000, 0.000000000000000000, 1.000000000000000000 ) ) ;
#38425=CARTESIAN_POINT ( 'NONE',  ( 19.99687500061451217, -4.119189519843965641, -2.378215178125001383 ) ) ;
#38428=CARTESIAN_POINT ( 'NONE',  ( 13.44375000122903252, -2.886751345948129988, 4.999999999999997335 ) ) ;
#38430=CARTESIAN_POINT ( 'NONE',  ( 7.396875000614516082, -4.119189519843965641, -2.378215178125001383 ) ) ;
#38434=CARTESIAN_POINT ( 'NONE',  ( 21.18749999999999645, -2.886751345948126435, -5.000000000000000000 ) ) ;
#38443=CARTESIAN_POINT ( 'NONE',  ( 29.37187500061451928, 2.746126346562643317, 4.756430356249998326 ) ) ;
#38448=CARTESIAN_POINT ( 'NONE',  ( 45.00000000000000000, 0.000000000000000000, 0.000000000000000000 ) ) ;
#38453=ORIENTED_EDGE ( 'NONE', *, *, #71543, .T. ) ;
#38465=CARTESIAN_POINT ( 'NONE',  ( 17.44687500061451502, -2.746126346562641984, -4.756430356249999214 ) ) ;
#38470=ORIENTED_EDGE ( 'NONE', *, *, #48083, .T. ) ;
#38481=VERTEX_POINT ( 'NONE', #53403 ) ;
#38494=CARTESIAN_POINT ( 'NONE',  ( 14.40000000000000036, -4.330127018922190985, -2.500000000000001332 ) ) ;
#38499=CARTESIAN_POINT ( 'NONE',  ( 18.98437500061451644, 4.119189519843966529, 2.378215178124999607 ) ) ;
#38506=CARTESIAN_POINT ( 'NONE',  ( 20.21250000000000213, -5.773502691896255534, -1.060575238724906372E-15 ) ) ;
#38510=CYLINDRICAL_SURFACE ( 'NONE', #7658, 4.999999999999998224 ) ;
#38512=CARTESIAN_POINT ( 'NONE',  ( 28.38749999999999929, -2.886751345948126435, -5.000000000000000000 ) ) ;
#38513=CARTESIAN_POINT ( 'NONE',  ( 17.62500000000000000, 6.123233995736764310E-16, -4.999999999999998224 ) ) ;
#38518=CARTESIAN_POINT ( 'NONE',  ( 28.28437500061451360, 5.492252693125287522, 3.363034840372157021E-16 ) ) ;
#38520=CARTESIAN_POINT ( 'NONE',  ( 12.68437500061451573, -2.746126346562646425, 4.756430356249996549 ) ) ;
#38529=CARTESIAN_POINT ( 'NONE',  ( 20.79375000122903216, -2.886751345948126435, -5.000000000000000000 ) ) ;
#38531=ORIENTED_EDGE ( 'NONE', *, *, #64823, .T. ) ;
#38536=ORIENTED_EDGE ( 'NONE', *, *, #14554, .T. ) ;
#38544=ORIENTED_EDGE ( 'NONE', *, *, #71436, .F. ) ;
#38554=CARTESIAN_POINT ( 'NONE',  ( 23.14687500061451786, -2.746126346562646425, 4.756430356249996549 ) ) ;
#38556=CARTESIAN_POINT ( 'NONE',  ( 7.396875000614519635, -2.746126346562646425, 4.756430356249996549 ) ) ;
#38574=CARTESIAN_POINT ( 'NONE',  ( 19.55625000122903145, 4.330127018922192761, -2.499999999999997780 ) ) ;
#38576=CARTESIAN_POINT ( 'NONE',  ( 26.00625000122903074, 0.000000000000000000, 4.999999999999998224 ) ) ;
#38590=CARTESIAN_POINT ( 'NONE',  ( 27.04687500061451644, 5.492252693125287522, 3.363034840372157021E-16 ) ) ;
#38595=ADVANCED_FACE ( 'NONE', ( #31233 ), #2795, .T. ) ;
#38600=AXIS2_PLACEMENT_3D ( 'NONE', #26371, #48911, #20817 ) ;
#38603=CARTESIAN_POINT ( 'NONE',  ( 8.849999999999999645, 0.000000000000000000, 4.999999999999998224 ) ) ;
#38606=CARTESIAN_POINT ( 'NONE',  ( 11.45625000122903181, 4.330127018922192761, -2.499999999999997780 ) ) ;
#38610=CARTESIAN_POINT ( 'NONE',  ( 20.48437500061451289, -2.746126346562641984, -4.756430356249999214 ) ) ;
#38621=CARTESIAN_POINT ( 'NONE',  ( 12.83437500061451786, -2.746126346562642428, -4.756430356249999214 ) ) ;
#38622=VERTEX_POINT ( 'NONE', #36044 ) ;
#38630=CARTESIAN_POINT ( 'NONE',  ( 14.74687500061451573, 4.119189519843966529, -2.378215178124998275 ) ) ;
#38646=CARTESIAN_POINT ( 'NONE',  ( 28.88437500061451502, -2.746126346562646425, 4.756430356249996549 ) ) ;
#38647=CARTESIAN_POINT ( 'NONE',  ( 14.74687500061451573, -2.746126346562642428, -4.756430356249999214 ) ) ;
#38655=CARTESIAN_POINT ( 'NONE',  ( 8.099999999999999645, -4.330127018922190985, -2.500000000000001332 ) ) ;
#38662=CARTESIAN_POINT ( 'NONE',  ( 25.72499999999999787, 6.123233995736764310E-16, -4.999999999999998224 ) ) ;
#38667=CARTESIAN_POINT ( 'NONE',  ( 26.04375000122902861, -2.886751345948129988, 4.999999999999997335 ) ) ;
#38681=CYLINDRICAL_SURFACE ( 'NONE', #58548, 4.999999999999998224 ) ;
#38704=LINE ( 'NONE', #27616, #57183 ) ;
#38711=ORIENTED_EDGE ( 'NONE', *, *, #9967, .T. ) ;
#38717=CARTESIAN_POINT ( 'NONE',  ( 20.40937500061451360, -5.492252693125287522, -1.008910452111647106E-15 ) ) ;
#38723=CARTESIAN_POINT ( 'NONE',  ( 7.429687500307258219, 0.000000000000000000, 4.878215178124998275 ) ) ;
#38724=VERTEX_POINT ( 'NONE', #58200 ) ;
#38725=CARTESIAN_POINT ( 'NONE',  ( 9.674999999999998934, 4.330127018922191873, 2.499999999999999556 ) ) ;
#38727=( BOUNDED_CURVE ( )  B_SPLINE_CURVE ( 2, ( #22810, #38736, #28723, #68263, #33180, #16543, #27647 ),
 .UNSPECIFIED., .F., .F. ) 
 B_SPLINE_CURVE_WITH_KNOTS ( ( 3, 2, 2, 3 ),
 ( 0.05000000000000005135, 0.05333333333333338533, 0.05666666666666670543, 0.06000000000000003941 ),
 .UNSPECIFIED. ) 
 CURVE ( )  GEOMETRIC_REPRESENTATION_ITEM ( )  RATIONAL_B_SPLINE_CURVE ( ( 0.9999999999999981126, 0.8660254037844407060, 1.000000000000000000, 0.8660254037844387076, 1.000000000000000000, 0.8660254037844370423, 1.000000000000001776 ) ) 
 REPRESENTATION_ITEM ( '' )  );
#38733=CARTESIAN_POINT ( 'NONE',  ( 22.88437500061451857, 5.824947211148865298E-16, -4.756430356249998326 ) ) ;
#38736=CARTESIAN_POINT ( 'NONE',  ( 28.44375000122902719, -2.886751345948149972, -4.999999999999956479 ) ) ;
#38755=CARTESIAN_POINT ( 'NONE',  ( 9.421875000614518214, 2.746126346562645981, -4.756430356249997438 ) ) ;
#38779=CARTESIAN_POINT ( 'NONE',  ( 10.43437500061451750, 4.119189519843966529, 2.378215178124999607 ) ) ;
#38795=CARTESIAN_POINT ( 'NONE',  ( 45.00000000000000000, 6.123233995736764310E-16, -4.999999999999998224 ) ) ;
#38796=CARTESIAN_POINT ( 'NONE',  ( 19.93125000122903145, 6.123233995736764310E-16, -4.999999999999998224 ) ) ;
#38800=CARTESIAN_POINT ( 'NONE',  ( 20.10937500061451644, 2.746126346562645981, -4.756430356249997438 ) ) ;
#38803=CARTESIAN_POINT ( 'NONE',  ( 14.23125000122903394, 4.330127018922191873, 2.499999999999999556 ) ) ;
#38805=CARTESIAN_POINT ( 'NONE',  ( 7.509375000614516793, 2.746126346562645981, -4.756430356249997438 ) ) ;
#38818=CARTESIAN_POINT ( 'NONE',  ( 29.74687500061451217, 5.492252693125287522, 3.363034840372157021E-16 ) ) ;
#38826=CARTESIAN_POINT ( 'NONE',  ( 15.15000000000000036, 0.000000000000000000, 4.999999999999998224 ) ) ;
#38840=CARTESIAN_POINT ( 'NONE',  ( 18.00937500061451502, 4.119189519843966529, -2.378215178124998275 ) ) ;
#38854=VERTEX_POINT ( 'NONE', #32332 ) ;
#38867=ORIENTED_EDGE ( 'NONE', *, *, #43418, .T. ) ;
#38870=CARTESIAN_POINT ( 'NONE',  ( 19.47187500061451360, 2.746126346562643317, 4.756430356249998326 ) ) ;
#38876=CARTESIAN_POINT ( 'NONE',  ( 19.61249999999999716, 2.886751345948126879, 4.999999999999999112 ) ) ;
#38879=CARTESIAN_POINT ( 'NONE',  ( 25.20937500061451431, 2.746126346562643317, 4.756430356249998326 ) ) ;
#38880=DIRECTION ( 'NONE',  ( 0.000000000000000000, 0.000000000000000000, 1.000000000000000000 ) ) ;
#38887=CARTESIAN_POINT ( 'NONE',  ( 26.25937500061451502, -5.492252693125287522, -1.008910452111647106E-15 ) ) ;
#38889=CARTESIAN_POINT ( 'NONE',  ( 13.13437500061451502, -2.746126346562646425, 4.756430356249996549 ) ) ;
#38906=FACE_OUTER_BOUND ( 'NONE', #63070, .T. ) ;
#38912=ORIENTED_EDGE ( 'NONE', *, *, #10796, .T. ) ;
#38917=ADVANCED_FACE ( 'NONE', ( #48233 ), #49701, .T. ) ;
#38921=CARTESIAN_POINT ( 'NONE',  ( 23.85937500061451644, 4.119189519843966529, -2.378215178124998275 ) ) ;
#38923=CARTESIAN_POINT ( 'NONE',  ( 8.371875000614515727, -5.492252693125287522, -1.008910452111647106E-15 ) ) ;
#38932=EDGE_CURVE ( 'NONE', #60154, #59530, #15330, .T. ) ;
#38934=LINE ( 'NONE', #31559, #32437 ) ;
#38941=CARTESIAN_POINT ( 'NONE',  ( 18.31875000122903430, 2.886751345948126879, 4.999999999999999112 ) ) ;
#38944=VERTEX_POINT ( 'NONE', #26061 ) ;
#38957=CARTESIAN_POINT ( 'NONE',  ( 25.20937500061451431, 4.119189519843966529, -2.378215178124998275 ) ) ;
#38964=CARTESIAN_POINT ( 'NONE',  ( 27.97500000000000142, 6.123233995736764310E-16, -4.999999999999998224 ) ) ;
#38966=CARTESIAN_POINT ( 'NONE',  ( 9.131250001229034297, 6.123233995736764310E-16, -4.999999999999998224 ) ) ;
#38968=CARTESIAN_POINT ( 'NONE',  ( 14.98125000122903216, 6.123233995736764310E-16, -4.999999999999998224 ) ) ;
#38971=CARTESIAN_POINT ( 'NONE',  ( 27.67499999999999716, 4.330127018922191873, 2.499999999999999556 ) ) ;
#38973=CARTESIAN_POINT ( 'NONE',  ( 11.49375000122903145, 5.773502691896255534, 3.535250795749688894E-16 ) ) ;
#38975=CARTESIAN_POINT ( 'NONE',  ( 13.93125000122903323, -4.330127018922194537, 2.499999999999995559 ) ) ;
#38977=CARTESIAN_POINT ( 'NONE',  ( 21.15937500061451715, 2.746126346562643317, 4.756430356249998326 ) ) ;
#38988=CARTESIAN_POINT ( 'NONE',  ( 13.43437500061451750, 5.492252693125287522, 3.363034840372157021E-16 ) ) ;
#38989=ORIENTED_EDGE ( 'NONE', *, *, #53045, .T. ) ;
#39002=EDGE_LOOP ( 'NONE', ( #16072, #55084, #37802, #33800 ) ) ;
#39011=CARTESIAN_POINT ( 'NONE',  ( 22.63125000122903430, 6.123233995736764310E-16, -4.999999999999998224 ) ) ;
#39012=CARTESIAN_POINT ( 'NONE',  ( 15.79687500061451821, 5.492252693125287522, 3.363034840372157021E-16 ) ) ;
#39020=CARTESIAN_POINT ( 'NONE',  ( 34.99999999999999289, 2.500000000000000444, 3.499999999999999112 ) ) ;
#39029=LINE ( 'NONE', #44936, #36268 ) ;
#39030=CARTESIAN_POINT ( 'NONE',  ( 25.51875000122903003, 2.886751345948126879, 4.999999999999999112 ) ) ;
#39075=CARTESIAN_POINT ( 'NONE',  ( 20.74687500061451217, 0.000000000000000000, 4.756430356249998326 ) ) ;
#39084=ORIENTED_EDGE ( 'NONE', *, *, #23045, .F. ) ;
#39086=CARTESIAN_POINT ( 'NONE',  ( 11.43750000000000000, 5.773502691896255534, 3.535250795749688894E-16 ) ) ;
#39092=CARTESIAN_POINT ( 'NONE',  ( 16.27499999999999858, 6.123233995736764310E-16, -4.999999999999998224 ) ) ;
#39093=CARTESIAN_POINT ( 'NONE',  ( 22.39687500061451075, -2.746126346562642428, -4.756430356249999214 ) ) ;
#39107=CARTESIAN_POINT ( 'NONE',  ( 27.16875000122903216, 2.886751345948164182, -4.999999999999937828 ) ) ;
#39114=CARTESIAN_POINT ( 'NONE',  ( 7.509375000614517681, -4.119189519843965641, -2.378215178125001383 ) ) ;
#39135=CARTESIAN_POINT ( 'NONE',  ( 11.52187500061451608, -5.492252693125287522, -1.008910452111647106E-15 ) ) ;
#39147=DIRECTION ( 'NONE',  ( 0.000000000000000000, 0.000000000000000000, 1.000000000000000000 ) ) ;
#39149=CARTESIAN_POINT ( 'NONE',  ( 45.00000000000000000, 6.123233995736764310E-16, -4.999999999999998224 ) ) ;
#39155=EDGE_CURVE ( 'NONE', #29422, #42476, #8951, .T. ) ;
#39156=DIRECTION ( 'NONE',  ( -1.000000000000000000, -0.000000000000000000, -0.000000000000000000 ) ) ;
#39159=CARTESIAN_POINT ( 'NONE',  ( 20.33437500061451786, -2.746126346562646425, 4.756430356249996549 ) ) ;
#39162=CARTESIAN_POINT ( 'NONE',  ( 13.29375000122903394, 5.773502691896255534, 3.535250795749688894E-16 ) ) ;
#39166=CARTESIAN_POINT ( 'NONE',  ( 7.781250001229034652, 6.123233995736764310E-16, -4.999999999999998224 ) ) ;
#39176=CARTESIAN_POINT ( 'NONE',  ( 29.33437500061451431, 4.119189519843966529, 2.378215178124999607 ) ) ;
#39200=CARTESIAN_POINT ( 'NONE',  ( 17.33437500061451431, -4.119189519843968306, 2.378215178124996054 ) ) ;
#39204=EDGE_LOOP ( 'NONE', ( #19838, #72818, #44161, #19467 ) ) ;
#39233=CARTESIAN_POINT ( 'NONE',  ( 19.84687500061451360, 5.492252693125287522, 3.363034840372157021E-16 ) ) ;
#39238=CARTESIAN_POINT ( 'NONE',  ( 19.08750000000000213, 5.773502691896255534, 3.535250795749688894E-16 ) ) ;
#39241=CARTESIAN_POINT ( 'NONE',  ( 21.63749999999999929, -2.886751345948126435, -5.000000000000000000 ) ) ;
#39242=CARTESIAN_POINT ( 'NONE',  ( 24.72187500061451360, 4.119189519843966529, 2.378215178124999607 ) ) ;
#39246=LINE ( 'NONE', #50335, #51417 ) ;
#39250=AXIS2_PLACEMENT_3D ( 'NONE', #52529, #51806, #41803 ) ;
#39251=CARTESIAN_POINT ( 'NONE',  ( 27.12187500061451573, -4.119189519843968306, 2.378215178124996054 ) ) ;
#39253=CARTESIAN_POINT ( 'NONE',  ( 13.35937500061451644, 2.746126346562645981, -4.756430356249997438 ) ) ;
#39276=LINE ( 'NONE', #24348, #42067 ) ;
#39286=CARTESIAN_POINT ( 'NONE',  ( 25.20937500061451431, 4.119189519843966529, -2.378215178124998275 ) ) ;
#39297=CARTESIAN_POINT ( 'NONE',  ( 17.26875000122903003, 2.886751345948185055, -4.999999999999902300 ) ) ;
#39306=CARTESIAN_POINT ( 'NONE',  ( 19.78125000122902932, -4.330127018922194537, 2.499999999999995559 ) ) ;
#39308=CARTESIAN_POINT ( 'NONE',  ( 24.60000000000000142, 0.000000000000000000, 4.999999999999998224 ) ) ;
#39323=CARTESIAN_POINT ( 'NONE',  ( 25.24687500061451573, 5.492252693125287522, 3.363034840372157021E-16 ) ) ;
#39328=CARTESIAN_POINT ( 'NONE',  ( 27.93750000000000000, -2.886751345948125991, -5.000000000000000000 ) ) ;
#39337=CARTESIAN_POINT ( 'NONE',  ( 12.39375000122903181, 5.773502691896255534, 3.535250795749688894E-16 ) ) ;
#39338=CARTESIAN_POINT ( 'NONE',  ( 13.12500000000000178, 6.123233995736764310E-16, -4.999999999999998224 ) ) ;
#39339=CARTESIAN_POINT ( 'NONE',  ( 13.89375000122902648, -2.886751345948019409, 5.000000000000189182 ) ) ;
#39341=CARTESIAN_POINT ( 'NONE',  ( 21.42187500061451644, 5.824947211148865298E-16, -4.756430356249998326 ) ) ;
#39352=CARTESIAN_POINT ( 'NONE',  ( 13.35937500061451644, 2.746126346562645981, -4.756430356249997438 ) ) ;
#39353=ORIENTED_EDGE ( 'NONE', *, *, #72743, .T. ) ;
#39358=VERTEX_POINT ( 'NONE', #912 ) ;
#39359=DIRECTION ( 'NONE',  ( -1.000000000000000000, -0.000000000000000000, -0.000000000000000000 ) ) ;
#39361=CARTESIAN_POINT ( 'NONE',  ( 11.10000000000000142, 0.000000000000000000, 4.999999999999998224 ) ) ;
#39374=CARTESIAN_POINT ( 'NONE',  ( 13.62187500061451750, 2.746126346562643317, 4.756430356249998326 ) ) ;
#39392=CARTESIAN_POINT ( 'NONE',  ( 26.68125000122903145, 6.123233995736764310E-16, -4.999999999999998224 ) ) ;
#39431=VERTEX_POINT ( 'NONE', #45286 ) ;
#39433=EDGE_CURVE ( 'NONE', #1784, #28145, #11306, .T. ) ;
#39435=ORIENTED_EDGE ( 'NONE', *, *, #71019, .T. ) ;
#39438=CARTESIAN_POINT ( 'NONE',  ( 18.19687500061451502, -4.119189519843965641, -2.378215178125001383 ) ) ;
#39447=ORIENTED_EDGE ( 'NONE', *, *, #20329, .F. ) ;
#39454=CARTESIAN_POINT ( 'NONE',  ( 21.72187500061451715, 2.746126346562643317, 4.756430356249998326 ) ) ;
#39464=CARTESIAN_POINT ( 'NONE',  ( 17.84999999999999787, 0.000000000000000000, 4.999999999999998224 ) ) ;
#39471=CARTESIAN_POINT ( 'NONE',  ( 18.30000000000000071, 0.000000000000000000, 4.999999999999998224 ) ) ;
#39480=VECTOR ( 'NONE', #34886, 1000.000000000000000 ) ;
#39485=ORIENTED_EDGE ( 'NONE', *, *, #35222, .T. ) ;
#39498=CARTESIAN_POINT ( 'NONE',  ( 17.39999999999999858, 0.000000000000000000, 4.999999999999998224 ) ) ;
#39499=CARTESIAN_POINT ( 'NONE',  ( 9.046875000614518214, 5.492252693125287522, 3.363034840372157021E-16 ) ) ;
#39500=DIRECTION ( 'NONE',  ( 0.000000000000000000, 0.000000000000000000, 1.000000000000000000 ) ) ;
#39511=CARTESIAN_POINT ( 'NONE',  ( 12.50625000122903430, 0.000000000000000000, 4.999999999999998224 ) ) ;
#39521=CARTESIAN_POINT ( 'NONE',  ( 18.75937500061451857, 2.746126346562645981, -4.756430356249997438 ) ) ;
#39524=CARTESIAN_POINT ( 'NONE',  ( 15.28125000122903288, -4.330127018922194537, 2.499999999999995559 ) ) ;
#39539=CARTESIAN_POINT ( 'NONE',  ( 29.22187500061451715, 2.746126346562645981, -4.756430356249997438 ) ) ;
#39543=CARTESIAN_POINT ( 'NONE',  ( 17.17500000000000071, 6.123233995736764310E-16, -4.999999999999998224 ) ) ;
#39546=CARTESIAN_POINT ( 'NONE',  ( 24.80625000122903145, -4.330127018922190985, -2.500000000000001332 ) ) ;
#39550=VERTEX_POINT ( 'NONE', #5761 ) ;
#39561=CARTESIAN_POINT ( 'NONE',  ( 15.15937500061451715, -4.119189519843965641, -2.378215178125001383 ) ) ;
#39565=ORIENTED_EDGE ( 'NONE', *, *, #65890, .F. ) ;
#39574=AXIS2_PLACEMENT_3D ( 'NONE', #64066, #8290, #64434 ) ;
#39593=CARTESIAN_POINT ( 'NONE',  ( 19.05937500061451928, 0.000000000000000000, 4.756430356249998326 ) ) ;
#39594=EDGE_CURVE ( 'NONE', #57985, #19407, #26414, .T. ) ;
#39596=( BOUNDED_CURVE ( )  B_SPLINE_CURVE ( 2, ( #15231, #39241, #49959, #50331, #22237, #26701, #72855 ),
 .UNSPECIFIED., .F., .F. ) 
 B_SPLINE_CURVE_WITH_KNOTS ( ( 3, 2, 2, 3 ),
 ( 0.3699999999999999956, 0.3733333333333333504, 0.3766666666666666496, 0.3800000000000000044 ),
 .UNSPECIFIED. ) 
 CURVE ( )  GEOMETRIC_REPRESENTATION_ITEM ( )  RATIONAL_B_SPLINE_CURVE ( ( 1.000000000000000000, 0.8660254037844387076, 1.000000000000000000, 0.8660254037844387076, 1.000000000000000000, 0.8660254037844387076, 1.000000000000000000 ) ) 
 REPRESENTATION_ITEM ( '' )  );
#39602=CARTESIAN_POINT ( 'NONE',  ( 18.78749999999999432, -2.886751345948129988, 4.999999999999997335 ) ) ;
#39606=CARTESIAN_POINT ( 'NONE',  ( 25.73437500061451644, -2.746126346562646425, 4.756430356249996549 ) ) ;
#39610=CARTESIAN_POINT ( 'NONE',  ( 17.51249999999999929, -5.773502691896255534, -1.060575238724906372E-15 ) ) ;
#39613=( BOUNDED_CURVE ( )  B_SPLINE_CURVE ( 2, ( #37150, #9083, #48245, #3550, #42336, #31620, #3918 ),
 .UNSPECIFIED., .F., .F. ) 
 B_SPLINE_CURVE_WITH_KNOTS ( ( 3, 2, 2, 3 ),
 ( 0.8100000000000000533, 0.8133333333333333526, 0.8166666666666667629, 0.8200000000000000622 ),
 .UNSPECIFIED. ) 
 CURVE ( )  GEOMETRIC_REPRESENTATION_ITEM ( )  RATIONAL_B_SPLINE_CURVE ( ( 1.000000000000000000, 0.8660254037844387076, 1.000000000000000000, 0.8660254037844387076, 1.000000000000000000, 0.8660254037844342667, 1.000000000000004441 ) ) 
 REPRESENTATION_ITEM ( '' )  );
#39615=CARTESIAN_POINT ( 'NONE',  ( 27.38437500061451502, 5.492252693125287522, 3.363034840372157021E-16 ) ) ;
#39617=CARTESIAN_POINT ( 'NONE',  ( 10.62187500061451395, 5.824947211148865298E-16, -4.756430356249998326 ) ) ;
#39623=CARTESIAN_POINT ( 'NONE',  ( 16.50000000000000000, 0.000000000000000000, 4.999999999999998224 ) ) ;
#39627=DIRECTION ( 'NONE',  ( -1.000000000000000000, -0.000000000000000000, -0.000000000000000000 ) ) ;
#39629=ORIENTED_EDGE ( 'NONE', *, *, #56668, .F. ) ;
#39643=VERTEX_POINT ( 'NONE', #72268 ) ;
#39653=CARTESIAN_POINT ( 'NONE',  ( 21.68437500061451573, 4.119189519843966529, 2.378215178124999607 ) ) ;
#39660=ORIENTED_EDGE ( 'NONE', *, *, #5302, .T. ) ;
#39672=CARTESIAN_POINT ( 'NONE',  ( 15.54375000122903394, 5.773502691896255534, 3.535250795749688894E-16 ) ) ;
#39681=CARTESIAN_POINT ( 'NONE',  ( 45.00000000000000000, 0.000000000000000000, 4.999999999999998224 ) ) ;
#39689=CARTESIAN_POINT ( 'NONE',  ( 26.78437500061451360, -4.119189519843968306, 2.378215178124996054 ) ) ;
#39694=CARTESIAN_POINT ( 'NONE',  ( 26.09999999999999787, -4.330127018922190985, -2.500000000000001332 ) ) ;
#39703=CARTESIAN_POINT ( 'NONE',  ( 12.13125000122903430, -4.330127018922194537, 2.499999999999995559 ) ) ;
#39707=CARTESIAN_POINT ( 'NONE',  ( 19.17187500061451289, 5.824947211148865298E-16, -4.756430356249998326 ) ) ;
#39713=DIRECTION ( 'NONE',  ( 0.000000000000000000, 0.000000000000000000, 1.000000000000000000 ) ) ;
#39715=EDGE_CURVE ( 'NONE', #45665, #66820, #44929, .T. ) ;
#39719=CARTESIAN_POINT ( 'NONE',  ( 13.65937500061451537, -5.492252693125287522, -1.008910452111647106E-15 ) ) ;
#39725=ORIENTED_EDGE ( 'NONE', *, *, #23556, .F. ) ;
#39743=CARTESIAN_POINT ( 'NONE',  ( 29.59687500061451360, 4.119189519843966529, -2.378215178124998275 ) ) ;
#39745=CARTESIAN_POINT ( 'NONE',  ( 13.02187500061451608, 2.746126346562645981, -4.756430356249997438 ) ) ;
#39755=DIRECTION ( 'NONE',  ( -1.000000000000000000, -0.000000000000000000, -0.000000000000000000 ) ) ;
#39762=CARTESIAN_POINT ( 'NONE',  ( 16.05000000000000071, 0.000000000000000000, 4.999999999999998224 ) ) ;
#39763=CARTESIAN_POINT ( 'NONE',  ( 24.16875000122903216, 2.886751345948126879, 4.999999999999999112 ) ) ;
#39766=ORIENTED_EDGE ( 'NONE', *, *, #43656, .F. ) ;
#39787=FACE_OUTER_BOUND ( 'NONE', #12848, .T. ) ;
#39809=CARTESIAN_POINT ( 'NONE',  ( 18.38437500061451502, 5.492252693125287522, 3.363034840372157021E-16 ) ) ;
#39827=CARTESIAN_POINT ( 'NONE',  ( 19.65937500061451360, -4.119189519843965641, -2.378215178125001383 ) ) ;
#39842=LINE ( 'NONE', #17998, #66570 ) ;
#39850=CARTESIAN_POINT ( 'NONE',  ( 8.109375000614518214, 4.119189519843966529, -2.378215178124998275 ) ) ;
#39854=EDGE_CURVE ( 'NONE', #61742, #4282, #57439, .T. ) ;
#39870=CARTESIAN_POINT ( 'NONE',  ( 17.90625000122903288, 0.000000000000000000, 4.999999999999998224 ) ) ;
#39871=CARTESIAN_POINT ( 'NONE',  ( 10.35937500061451644, 4.119189519843966529, -2.378215178124998275 ) ) ;
#39876=VECTOR ( 'NONE', #29024, 1000.000000000000000 ) ;
#39891=CARTESIAN_POINT ( 'NONE',  ( 18.04687500061451644, 0.000000000000000000, 4.756430356249998326 ) ) ;
#39894=CARTESIAN_POINT ( 'NONE',  ( 26.40937500061451360, 2.746126346562645981, -4.756430356249997438 ) ) ;
#39900=CARTESIAN_POINT ( 'NONE',  ( 21.03749999999999787, -2.886751345948102898, 5.000000000000044409 ) ) ;
#39901=CARTESIAN_POINT ( 'NONE',  ( 21.67500000000000071, 6.123233995736764310E-16, -4.999999999999998224 ) ) ;
#39902=CYLINDRICAL_SURFACE ( 'NONE', #36026, 4.999999999999998224 ) ;
#39908=CARTESIAN_POINT ( 'NONE',  ( 27.98437500061451289, 4.119189519843966529, 2.378215178124999607 ) ) ;
#39914=CARTESIAN_POINT ( 'NONE',  ( 45.00000000000000000, 6.123233995736764310E-16, -4.999999999999998224 ) ) ;
#39917=ORIENTED_EDGE ( 'NONE', *, *, #48306, .T. ) ;
#39927=CARTESIAN_POINT ( 'NONE',  ( 15.23437500061451644, 5.824947211148865298E-16, -4.756430356249998326 ) ) ;
#39935=ADVANCED_FACE ( 'NONE', ( #51186 ), #46368, .T. ) ;
#39958=CARTESIAN_POINT ( 'NONE',  ( 16.02187500061451786, -5.492252693125287522, -1.008910452111647106E-15 ) ) ;
#39964=CARTESIAN_POINT ( 'NONE',  ( 18.97499999999999787, 6.123233995736764310E-16, -4.999999999999998224 ) ) ;
#39968=CARTESIAN_POINT ( 'NONE',  ( 24.53437500061451715, -2.746126346562641984, -4.756430356249999214 ) ) ;
#39977=CARTESIAN_POINT ( 'NONE',  ( 24.00937500061451502, -5.492252693125287522, -1.008910452111647106E-15 ) ) ;
#39979=CARTESIAN_POINT ( 'NONE',  ( 10.39687500061451608, 0.000000000000000000, 4.756430356249998326 ) ) ;
#39984=CARTESIAN_POINT ( 'NONE',  ( 8.081250001229031810, -4.330127018922194537, 2.499999999999995559 ) ) ;
#39988=ORIENTED_EDGE ( 'NONE', *, *, #14507, .T. ) ;
#39990=CARTESIAN_POINT ( 'NONE',  ( 15.34687500061451537, 0.000000000000000000, 4.756430356249998326 ) ) ;
#40000=CARTESIAN_POINT ( 'NONE',  ( 18.75000000000000000, 0.000000000000000000, 4.999999999999998224 ) ) ;
#40011=CARTESIAN_POINT ( 'NONE',  ( 22.39687500061451075, -2.746126346562641984, -4.756430356249999214 ) ) ;
#40023=DIRECTION ( 'NONE',  ( -1.000000000000000000, -0.000000000000000000, -0.000000000000000000 ) ) ;
#40032=CARTESIAN_POINT ( 'NONE',  ( 16.51875000122903359, 2.886751345948126879, 4.999999999999999112 ) ) ;
#40034=DIRECTION ( 'NONE',  ( -1.000000000000000000, -0.000000000000000000, -0.000000000000000000 ) ) ;
#40043=( BOUNDED_CURVE ( )  B_SPLINE_CURVE ( 2, ( #26246, #15146, #71681, #37683, #43606, #3358, #38796 ),
 .UNSPECIFIED., .F., .F. ) 
 B_SPLINE_CURVE_WITH_KNOTS ( ( 3, 2, 2, 3 ),
 ( 0.4200000000000000955, 0.4233333333333334503, 0.4266666666666668051, 0.4300000000000001044 ),
 .UNSPECIFIED. ) 
 CURVE ( )  GEOMETRIC_REPRESENTATION_ITEM ( )  RATIONAL_B_SPLINE_CURVE ( ( 0.9999999999999955591, 0.8660254037844431485, 1.000000000000000000, 0.8660254037844387076, 1.000000000000000000, 0.8660254037844342667, 1.000000000000004441 ) ) 
 REPRESENTATION_ITEM ( '' )  );
#40050=CARTESIAN_POINT ( 'NONE',  ( 24.23437500061451644, 5.824947211148865298E-16, -4.756430356249998326 ) ) ;
#40055=CARTESIAN_POINT ( 'NONE',  ( 27.75000000000000000, 0.000000000000000000, 4.999999999999998224 ) ) ;
#40063=CARTESIAN_POINT ( 'NONE',  ( 8.906250001229031099, 0.000000000000000000, 4.999999999999998224 ) ) ;
#40067=CARTESIAN_POINT ( 'NONE',  ( 19.58437500061451786, -2.746126346562641984, -4.756430356249999214 ) ) ;
#40070=ORIENTED_EDGE ( 'NONE', *, *, #2651, .F. ) ;
#40078=CARTESIAN_POINT ( 'NONE',  ( 13.28437500061451537, -2.746126346562642428, -4.756430356249999214 ) ) ;
#40079=ORIENTED_EDGE ( 'NONE', *, *, #51734, .F. ) ;
#40085=ORIENTED_EDGE ( 'NONE', *, *, #67290, .F. ) ;
#40099=CARTESIAN_POINT ( 'NONE',  ( 28.24687500061451573, -2.746126346562641984, -4.756430356249999214 ) ) ;
#40102=CARTESIAN_POINT ( 'NONE',  ( 29.52187500061451431, 5.824947211148865298E-16, -4.756430356249998326 ) ) ;
#40103=CARTESIAN_POINT ( 'NONE',  ( 13.73437500061451821, -4.119189519843968306, 2.378215178124996054 ) ) ;
#40119=CARTESIAN_POINT ( 'NONE',  ( 23.19375000122902719, 5.773502691896255534, 3.535250795749688894E-16 ) ) ;
#40122=ORIENTED_EDGE ( 'NONE', *, *, #55670, .T. ) ;
#40128=CARTESIAN_POINT ( 'NONE',  ( 28.87499999999999645, 6.123233995736764310E-16, -4.999999999999998224 ) ) ;
#40150=CARTESIAN_POINT ( 'NONE',  ( 7.875000000000000000, 4.330127018922191873, 2.499999999999999556 ) ) ;
#40163=ORIENTED_EDGE ( 'NONE', *, *, #38317, .F. ) ;
#40166=CARTESIAN_POINT ( 'NONE',  ( 19.09687500061451360, -4.119189519843965641, -2.378215178125001383 ) ) ;
#40182=CARTESIAN_POINT ( 'NONE',  ( 18.90937500061451360, 4.119189519843966529, -2.378215178124998275 ) ) ;
#40192=CYLINDRICAL_SURFACE ( 'NONE', #59570, 4.999999999999998224 ) ;
#40193=ORIENTED_EDGE ( 'NONE', *, *, #55155, .F. ) ;
#40212=ORIENTED_EDGE ( 'NONE', *, *, #40242, .T. ) ;
#40224=CARTESIAN_POINT ( 'NONE',  ( 8.334375000614516082, -4.119189519843968306, 2.378215178124996054 ) ) ;
#40225=LINE ( 'NONE', #6965, #37068 ) ;
#40242=EDGE_CURVE ( 'NONE', #31518, #44291, #43480, .T. ) ;
#40245=CARTESIAN_POINT ( 'NONE',  ( 17.10937500061451644, 2.746126346562643317, 4.756430356249998326 ) ) ;
#40248=CARTESIAN_POINT ( 'NONE',  ( 27.34687500061451360, 4.119189519843966529, -2.378215178124998275 ) ) ;
#40262=CARTESIAN_POINT ( 'NONE',  ( 26.07187500061451857, 2.746126346562645981, -4.756430356249997438 ) ) ;
#40268=CARTESIAN_POINT ( 'NONE',  ( 24.65625000122903288, 0.000000000000000000, 4.999999999999998224 ) ) ;
#40280=CARTESIAN_POINT ( 'NONE',  ( 14.67187500061451821, -5.492252693125287522, -1.008910452111647106E-15 ) ) ;
#40309=CARTESIAN_POINT ( 'NONE',  ( 16.77187500061451786, 2.746126346562643317, 4.756430356249998326 ) ) ;
#40316=CARTESIAN_POINT ( 'NONE',  ( 16.31250000000000000, 2.886751345948129099, -4.999999999999998224 ) ) ;
#40319=CARTESIAN_POINT ( 'NONE',  ( 29.80312500061451431, 0.000000000000000000, 4.999999999999998224 ) ) ;
#40320=CARTESIAN_POINT ( 'NONE',  ( 26.22187500061451360, -4.119189519843968306, 2.378215178124996054 ) ) ;
#40326=EDGE_CURVE ( 'NONE', #8225, #9764, #68058, .T. ) ;
#40328=CARTESIAN_POINT ( 'NONE',  ( 25.69687500061451502, 0.000000000000000000, 4.756430356249998326 ) ) ;
#40330=CARTESIAN_POINT ( 'NONE',  ( 11.97187500061451537, 5.824947211148865298E-16, -4.756430356249998326 ) ) ;
#40338=CARTESIAN_POINT ( 'NONE',  ( 16.01249999999999929, 2.886751345948126879, 4.999999999999998224 ) ) ;
#40341=CARTESIAN_POINT ( 'NONE',  ( 12.15937500061451360, 2.746126346562643317, 4.756430356249998326 ) ) ;
#40360=CARTESIAN_POINT ( 'NONE',  ( 11.40000000000000036, 4.330127018922192761, -2.499999999999997780 ) ) ;
#40362=CARTESIAN_POINT ( 'NONE',  ( 22.95937500061451431, 4.119189519843966529, -2.378215178124998275 ) ) ;
#40383=CARTESIAN_POINT ( 'NONE',  ( 16.70625000122903359, -4.330127018922190985, -2.500000000000001332 ) ) ;
#40399=CARTESIAN_POINT ( 'NONE',  ( 23.25937500061451857, -4.119189519843965641, -2.378215178125001383 ) ) ;
#40406=CARTESIAN_POINT ( 'NONE',  ( 24.11249999999999716, 2.886751345948126879, 4.999999999999999112 ) ) ;
#40416=CARTESIAN_POINT ( 'NONE',  ( 9.468750001229032875, -5.773502691896255534, -1.060575238724906372E-15 ) ) ;
#40417=CARTESIAN_POINT ( 'NONE',  ( 8.925000000000002487, -4.330127018922194537, 2.499999999999995559 ) ) ;
#40419=CARTESIAN_POINT ( 'NONE',  ( 17.70937500061451431, -5.492252693125287522, -1.008910452111647106E-15 ) ) ;
#40430=CARTESIAN_POINT ( 'NONE',  ( 9.834375000614514306, 5.492252693125287522, 3.363034840372157021E-16 ) ) ;
#40444=CARTESIAN_POINT ( 'NONE',  ( 10.23750000000000071, -2.886751345948129988, 4.999999999999997335 ) ) ;
#40453=CARTESIAN_POINT ( 'NONE',  ( 28.69687500061451502, -2.746126346562641984, -4.756430356249999214 ) ) ;
#40456=CARTESIAN_POINT ( 'NONE',  ( 27.23437500061450933, -2.746126346562641984, -4.756430356249999214 ) ) ;
#40457=CARTESIAN_POINT ( 'NONE',  ( 12.53437500061451537, 5.824947211148865298E-16, -4.756430356249998326 ) ) ;
#40475=CARTESIAN_POINT ( 'NONE',  ( 24.09375000122903288, 5.773502691896255534, 3.535250795749688894E-16 ) ) ;
#40524=CARTESIAN_POINT ( 'NONE',  ( 19.13437500061451502, -2.746126346562642428, -4.756430356249999214 ) ) ;
#40532=FACE_OUTER_BOUND ( 'NONE', #61776, .T. ) ;
#40540=FACE_OUTER_BOUND ( 'NONE', #31884, .T. ) ;
#40541=CARTESIAN_POINT ( 'NONE',  ( 20.18437500061451573, 5.824947211148865298E-16, -4.756430356249998326 ) ) ;
#40553=VERTEX_POINT ( 'NONE', #12504 ) ;
#40559=CARTESIAN_POINT ( 'NONE',  ( 29.53125000122903288, 4.330127018922191873, 2.499999999999999556 ) ) ;
#40563=DIRECTION ( 'NONE',  ( -1.000000000000000000, -0.000000000000000000, -0.000000000000000000 ) ) ;
#40580=EDGE_CURVE ( 'NONE', #26527, #31980, #38287, .T. ) ;
#40585=CARTESIAN_POINT ( 'NONE',  ( 10.09687500061451715, -2.746126346562646425, 4.756430356249996549 ) ) ;
#40594=FACE_OUTER_BOUND ( 'NONE', #36423, .T. ) ;
#40602=( BOUNDED_CURVE ( )  B_SPLINE_CURVE ( 2, ( #42176, #42540, #25917, #65431, #31083, #14457, #3015 ),
 .UNSPECIFIED., .F., .F. ) 
 B_SPLINE_CURVE_WITH_KNOTS ( ( 3, 2, 2, 3 ),
 ( 0.3099999999999999978, 0.3133333333333333526, 0.3166666666666665964, 0.3199999999999999512 ),
 .UNSPECIFIED. ) 
 CURVE ( )  GEOMETRIC_REPRESENTATION_ITEM ( )  RATIONAL_B_SPLINE_CURVE ( ( 1.000000000000000000, 0.8660254037844387076, 1.000000000000000000, 0.8660254037844387076, 1.000000000000000000, 0.8660254037844409281, 0.9999999999999977796 ) ) 
 REPRESENTATION_ITEM ( '' )  );
#40605=CARTESIAN_POINT ( 'NONE',  ( 18.27187500061451431, 5.824947211148865298E-16, -4.756430356249998326 ) ) ;
#40608=CARTESIAN_POINT ( 'NONE',  ( 26.37187500061451573, 5.824947211148865298E-16, -4.756430356249998326 ) ) ;
#40625=CARTESIAN_POINT ( 'NONE',  ( 26.37187500061451217, -5.492252693125287522, -1.008910452111647106E-15 ) ) ;
#40631=DIRECTION ( 'NONE',  ( -1.000000000000000000, -0.000000000000000000, -0.000000000000000000 ) ) ;
#40643=CARTESIAN_POINT ( 'NONE',  ( 15.68437500061451573, 5.824947211148865298E-16, -4.756430356249998326 ) ) ;
#40656=VERTEX_POINT ( 'NONE', #2872 ) ;
#40663=( BOUNDED_CURVE ( )  B_SPLINE_CURVE ( 2, ( #8050, #53480, #70474, #53854, #3246, #36122, #20211 ),
 .UNSPECIFIED., .F., .F. ) 
 B_SPLINE_CURVE_WITH_KNOTS ( ( 3, 2, 2, 3 ),
 ( 0.5300000000000000266, 0.5333333333333333259, 0.5366666666666667362, 0.5400000000000001465 ),
 .UNSPECIFIED. ) 
 CURVE ( )  GEOMETRIC_REPRESENTATION_ITEM ( )  RATIONAL_B_SPLINE_CURVE ( ( 1.000000000000000000, 0.8660254037844387076, 1.000000000000000000, 0.8660254037844387076, 1.000000000000000000, 0.8660254037844342667, 1.000000000000004441 ) ) 
 REPRESENTATION_ITEM ( '' )  );
#40669=VERTEX_POINT ( 'NONE', #42036 ) ;
#40674=CARTESIAN_POINT ( 'NONE',  ( 15.83437500061451608, 4.119189519843966529, 2.378215178124999607 ) ) ;
#40677=( BOUNDED_CURVE ( )  B_SPLINE_CURVE ( 2, ( #62257, #35261, #6106, #51899, #24537, #12009, #63339, #58142, #1297, #7548, #57428, #51541, #51175, #18619, #68892, #18249, #34532, #34900, #46722, #29720, #11654, #40822, #12725, #69257, #6832, #57783, #579, #57062, #2026, #23449, #23807, #40453, #34169, #45642, #46358, #942, #7192, #41184, #68532, #63693, #29004, #13084, #35622, #40099, #17893, #30082, #6469, #23084, #52620, #18977, #68174, #17537, #2377, #64788, #65525, #20073, #71069, #65153, #14179, #59235, #64056, #13436, #26369, #31547, #3107, #35986, #20444, #47440, #54087, #54449, #36713, #48542, #71440, #24895, #30810, #14543, #53343, #8643, #2741, #64424, #30452, #31172, #25260, #69972, #42629, #3848, #53715, #25636, #42994, #48909, #8280, #41538, #37079, #58505, #48174, #7915, #13816, #59603, #37453, #70698, #59972, #9017, #3485, #26003, #14911, #9381, #31913, #52981, #19342, #41897, #36356, #47807, #58870, #70336, #19713, #42265, #55183, #10475, #21547, #27843, #38175, #55905, #32642, #66628, #39286, #72168, #55543, #60699, #60333, #11203, #21180, #33730, #15274, #4578, #4939, #5297, #44474, #28201, #10112, #56276, #33369, #61077, #33004, #37813, #43732, #61800, #27108, #72530, #27473, #50374, #50005, #22281, #71810, #49641, #16366, #15634, #9742, #21918, #50730, #67005, #38921, #5665, #66256, #20815, #72899, #10833, #61440, #44102, #16005, #32276, #65894, #43370, #44833, #67368, #54810, #16731, #26744, #4216, #49277, #38554, #7104, #45908, #29633, #51808, #40362, #11922, #56975, #28912, #62881, #6019, #68439, #62525, #28554, #1211, #12997, #23360, #12277, #52171, #7463, #40011, #133, #29989, #34809, #57699, #63607, #57340, #34447, #12640, #17453, #58054, #68806, #40731, #6745, #18162, #1573, #29278, #67720, #63246, #39653, #51089, #6379, #23717, #485, #24082, #51450, #46267, #853, #46629, #17802, #35175, #69171, #18531, #35533, #41096, #22638, #62172, #45188, #22995, #11569, #17093, #34084, #56625, #45555, #68086, #3018, #59890, #69885, #14825, #65069, #24807, #53254, #14461, #19990, #52531, #25549, #42911, #59517, #70251, #2653, #9295, #58784, #65434, #13728, #47712, #30722, #42543, #37367, #25171, #8930, #1939, #35892, #41805, #48092, #64336, #19623, #36270, #2291, #41450, #31460, #8194, #42180, #53626, #24445, #64705, #14089, #54003, #46993, #19250, #69529, #70616, #18888, #36629, #63968, #47352, #36994, #48460, #59150, #70984, #8559, #31087, #13351, #3399, #25920, #20360, #58416, #7829, #30365, #52894, #43648, #43286, #66537, #60246, #61355, #66172, #21460, #32559, #38840, #49194, #27026, #15548, #4852, #50290, #10023, #15917, #71727, #71353, #22197, #32194, #44751, #26285, #38091, #38465, #66916, #55460, #39200, #21097, #67285, #44391, #4130, #55097, #16285, #60991, #60614, #10390, #32922, #72442, #4497, #27386, #48822, #26660, #16644, #49557, #72078, #44015, #3761, #15188, #49918, #21826, #10752, #33283, #55822, #5210, #27751, #72814, #61714, #9660, #31828, #54366, #20727, #65806, #37726, #54727, #51363, #45823, #45102, #34358, #35092, #62801, #40643, #34721, #56890, #45465, #5579, #56186, #69087, #1128, #68359, #28116, #63162, #17004, #39927, #765, #39561, #6295, #399, #62086, #12194, #23998, #28824, #23273, #12557, #17720, #6665, #67997, #18448, #40280, #68722, #1492, #57251, #51001, #23637, #28466, #41013, #29193, #51727, #46183, #18082, #57617, #7020, #50645, #29551, #17370, #11113, #52087, #46546, #33642, #49, #22554, #67638, #11479, #34002, #56539, #5932, #22907, #62441, #11839, #8839, #41723, #25087, #30278, #29910, #52450, #36182, #2934, #70900, #2211, #70163, #2567, #47269, #58331, #58700, #7742, #42098, #19540, #57972, #30638, #64620, #69803, #14007, #36545, #31005, #64250, #20272, #19169, #8110, #13638, #53170, #47630, #19910, #59065, #8470, #7379, #63880, #31375, #52810, #53538, #25463, #48007, #70535, #64985, #41370, #42463, #14376, #12915, #36911, #59431, #1856, #53916, #24363, #3309, #13271, #63528, #25836, #48373, #35448, #35809, #24726, #46910, #69449, #18806, #32839, #4770, #71261, #60903, #9574, #27303, #20641, #26199, #32476, #15464, #49837, #21377, #9938, #54639, #26569, #49110, #37641, #38009, #60164, #43931, #49469, #55009, #72002, #71639, #66457, #15834, #10306, #66086, #38379, #37280, #15105, #55738, #4044, #60531, #21012, #14738, #48738, #26944, #32106, #55376, #72361, #21742, #44303, #66832, #16204, #38755, #43199, #43564, #61276, #4415, #59802, #10669, #50205, #33199, #5132, #3675, #27666, #72730, #42824, #65348, #9208, #65719, #31743, #54281, #67201, #6942, #12118, #56809, #16563, #1049, #28035, #34642, #35011, #67917, #29114, #52010, #5496, #11400, #45746, #33919, #39850, #50922, #62363, #50564, #17288, #56462, #73091, #23192, #57541, #45381, #11760, #23558, #29473, #61999, #22114, #68282, #39114, #34277, #44671, #45023, #17643 ),
 .UNSPECIFIED., .F., .F. ) 
 B_SPLINE_CURVE_WITH_KNOTS ( ( 3, 2, 2, 2, 2, 2, 2, 2, 2, 2, 2, 2, 2, 2, 2, 2, 2, 2, 2, 2, 2, 2, 2, 2, 2, 2, 2, 2, 2, 2, 2, 2, 2, 2, 2, 2, 2, 2, 2, 2, 2, 2, 2, 2, 2, 2, 2, 2, 2, 2, 2, 2, 2, 2, 2, 2, 2, 2, 2, 2, 2, 2, 2, 2, 2, 2, 2, 2, 2, 2, 2, 2, 2, 2, 2, 2, 2, 2, 2, 2, 2, 2, 2, 2, 2, 2, 2, 2, 2, 2, 2, 2, 2, 2, 2, 2, 2, 2, 2, 2, 2, 2, 2, 2, 2, 2, 2, 2, 2, 2, 2, 2, 2, 2, 2, 2, 2, 2, 2, 2, 2, 2, 2, 2, 2, 2, 2, 2, 2, 2, 2, 2, 2, 2, 2, 2, 2, 2, 2, 2, 2, 2, 2, 2, 2, 2, 2, 2, 2, 2, 2, 2, 2, 2, 2, 2, 2, 2, 2, 2, 2, 2, 2, 2, 2, 2, 2, 2, 2, 2, 2, 2, 2, 2, 2, 2, 2, 2, 2, 2, 2, 2, 2, 2, 2, 2, 2, 2, 2, 2, 2, 2, 2, 2, 2, 2, 2, 2, 2, 2, 2, 2, 2, 2, 2, 2, 2, 2, 2, 2, 2, 2, 2, 2, 2, 2, 2, 2, 2, 2, 2, 2, 2, 2, 2, 2, 2, 2, 2, 2, 2, 2, 2, 2, 2, 2, 2, 2, 2, 2, 2, 2, 2, 2, 2, 2, 2, 2, 2, 2, 2, 2, 2, 2, 2, 2, 2, 2, 2, 2, 2, 2, 2, 2, 2, 2, 2, 2, 2, 2, 2, 2, 2, 2, 2, 2, 2, 2, 2, 2, 2, 2, 2, 2, 2, 2, 2, 2, 2, 2, 2, 2, 2, 2, 2, 2, 2, 2, 2, 2, 3 ),
 ( 0.000000000000000000, 0.003333333333333333547, 0.006666666666666667095, 0.01000000000000000021, 0.01333333333333333419, 0.01666666666666666644, 0.02000000000000000042, 0.02333333333333333440, 0.02666666666666666838, 0.02999999999999999889, 0.03333333333333333287, 0.03666666666666666685, 0.04000000000000000083, 0.04333333333333333481, 0.04666666666666666879, 0.05000000000000000278, 0.05333333333333333676, 0.05666666666666666380, 0.05999999999999999778, 0.06333333333333333870, 0.06666666666666666574, 0.07000000000000000666, 0.07333333333333333370, 0.07666666666666666075, 0.08000000000000000167, 0.08333333333333332871, 0.08666666666666666963, 0.08999999999999999667, 0.09333333333333333759, 0.09666666666666666463, 0.1000000000000000056, 0.1033333333333333326, 0.1066666666666666735, 0.1100000000000000006, 0.1133333333333333276, 0.1166666666666666685, 0.1199999999999999956, 0.1233333333333333365, 0.1266666666666666774, 0.1300000000000000044, 0.1333333333333333315, 0.1366666666666666585, 0.1400000000000000133, 0.1433333333333333404, 0.1466666666666666674, 0.1499999999999999944, 0.1533333333333333215, 0.1566666666666666763, 0.1600000000000000033, 0.1633333333333333304, 0.1666666666666666574, 0.1700000000000000122, 0.1733333333333333393, 0.1766666666666666663, 0.1799999999999999933, 0.1833333333333333204, 0.1866666666666666752, 0.1900000000000000022, 0.1933333333333333293, 0.1966666666666666563, 0.2000000000000000111, 0.2033333333333333381, 0.2066666666666666652, 0.2099999999999999922, 0.2133333333333333470, 0.2166666666666666741, 0.2200000000000000011, 0.2233333333333333282, 0.2266666666666666552, 0.2300000000000000100, 0.2333333333333333370, 0.2366666666666666641, 0.2399999999999999911, 0.2433333333333333459, 0.2466666666666666730, 0.2500000000000000000, 0.2533333333333333548, 0.2566666666666666541, 0.2600000000000000089, 0.2633333333333333082, 0.2666666666666666630, 0.2700000000000000178, 0.2733333333333333171, 0.2766666666666666718, 0.2800000000000000266, 0.2833333333333333259, 0.2866666666666666807, 0.2899999999999999800, 0.2933333333333333348, 0.2966666666666666896, 0.2999999999999999889, 0.3033333333333333437, 0.3066666666666666430, 0.3099999999999999978, 0.3133333333333333526, 0.3166666666666666519, 0.3200000000000000067, 0.3233333333333333059, 0.3266666666666666607, 0.3300000000000000155, 0.3333333333333333148, 0.3366666666666666696, 0.3400000000000000244, 0.3433333333333333237, 0.3466666666666666785, 0.3499999999999999778, 0.3533333333333333326, 0.3566666666666666874, 0.3599999999999999867, 0.3633333333333333415, 0.3666666666666666408, 0.3699999999999999956, 0.3733333333333333504, 0.3766666666666666496, 0.3800000000000000044, 0.3833333333333333592, 0.3866666666666666585, 0.3900000000000000133, 0.3933333333333333126, 0.3966666666666666674, 0.4000000000000000222, 0.4033333333333333215, 0.4066666666666666763, 0.4099999999999999756, 0.4133333333333333304, 0.4166666666666666852, 0.4199999999999999845, 0.4233333333333333393, 0.4266666666666666941, 0.4299999999999999933, 0.4333333333333333481, 0.4366666666666666474, 0.4400000000000000022, 0.4433333333333333570, 0.4466666666666666563, 0.4500000000000000111, 0.4533333333333333104, 0.4566666666666666652, 0.4600000000000000200, 0.4633333333333333193, 0.4666666666666666741, 0.4699999999999999734, 0.4733333333333333282, 0.4766666666666666829, 0.4799999999999999822, 0.4833333333333333370, 0.4866666666666666918, 0.4899999999999999911, 0.4933333333333333459, 0.4966666666666666452, 0.5000000000000000000, 0.5033333333333332993, 0.5066666666666667096, 0.5100000000000000089, 0.5133333333333333082, 0.5166666666666667185, 0.5200000000000000178, 0.5233333333333333171, 0.5266666666666666163, 0.5300000000000000266, 0.5333333333333333259, 0.5366666666666666252, 0.5400000000000000355, 0.5433333333333333348, 0.5466666666666666341, 0.5500000000000000444, 0.5533333333333333437, 0.5566666666666666430, 0.5600000000000000533, 0.5633333333333333526, 0.5666666666666666519, 0.5699999999999999512, 0.5733333333333333615, 0.5766666666666666607, 0.5799999999999999600, 0.5833333333333333703, 0.5866666666666666696, 0.5899999999999999689, 0.5933333333333333792, 0.5966666666666666785, 0.5999999999999999778, 0.6033333333333333881, 0.6066666666666666874, 0.6099999999999999867, 0.6133333333333332860, 0.6166666666666666963, 0.6199999999999999956, 0.6233333333333332948, 0.6266666666666667052, 0.6300000000000000044, 0.6333333333333333037, 0.6366666666666667140, 0.6400000000000000133, 0.6433333333333333126, 0.6466666666666666119, 0.6500000000000000222, 0.6533333333333333215, 0.6566666666666666208, 0.6600000000000000311, 0.6633333333333333304, 0.6666666666666666297, 0.6700000000000000400, 0.6733333333333333393, 0.6766666666666666385, 0.6800000000000000488, 0.6833333333333333481, 0.6866666666666666474, 0.6899999999999999467, 0.6933333333333333570, 0.6966666666666666563, 0.6999999999999999556, 0.7033333333333333659, 0.7066666666666666652, 0.7099999999999999645, 0.7133333333333333748, 0.7166666666666666741, 0.7199999999999999734, 0.7233333333333333837, 0.7266666666666666829, 0.7299999999999999822, 0.7333333333333332815, 0.7366666666666666918, 0.7399999999999999911, 0.7433333333333332904, 0.7466666666666667007, 0.7500000000000000000, 0.7533333333333332993, 0.7566666666666667096, 0.7600000000000000089, 0.7633333333333333082, 0.7666666666666667185, 0.7700000000000000178, 0.7733333333333333171, 0.7766666666666666163, 0.7800000000000000266, 0.7833333333333333259, 0.7866666666666666252, 0.7900000000000000355, 0.7933333333333333348, 0.7966666666666666341, 0.8000000000000000444, 0.8033333333333333437, 0.8066666666666666430, 0.8100000000000000533, 0.8133333333333333526, 0.8166666666666666519, 0.8199999999999999512, 0.8233333333333333615, 0.8266666666666666607, 0.8299999999999999600, 0.8333333333333333703, 0.8366666666666666696, 0.8399999999999999689, 0.8433333333333333792, 0.8466666666666666785, 0.8499999999999999778, 0.8533333333333333881, 0.8566666666666666874, 0.8599999999999999867, 0.8633333333333332860, 0.8666666666666666963, 0.8699999999999999956, 0.8733333333333332948, 0.8766666666666667052, 0.8800000000000000044, 0.8833333333333333037, 0.8866666666666667140, 0.8900000000000000133, 0.8933333333333333126, 0.8966666666666666119, 0.9000000000000000222, 0.9033333333333333215, 0.9066666666666666208, 0.9100000000000000311, 0.9133333333333333304, 0.9166666666666666297, 0.9200000000000000400, 0.9233333333333333393, 0.9266666666666666385, 0.9300000000000000488, 0.9333333333333333481, 0.9366666666666666474, 0.9399999999999999467, 0.9433333333333333570, 0.9466666666666666563, 0.9499999999999999556, 0.9533333333333333659, 0.9566666666666666652, 0.9599999999999999645, 0.9633333333333333748, 0.9666666666666666741, 0.9699999999999999734, 0.9733333333333333837, 0.9766666666666666829, 0.9799999999999999822, 0.9833333333333332815, 0.9866666666666666918, 0.9899999999999999911, 0.9933333333333332904, 0.9966666666666667007, 1.000000000000000000 ),
 .UNSPECIFIED. ) 
 CURVE ( )  GEOMETRIC_REPRESENTATION_ITEM ( )  RATIONAL_B_SPLINE_CURVE ( ( 1.000000000000000000, 0.8660254037844387076, 1.000000000000000000, 0.8660254037844387076, 1.000000000000000000, 0.8660254037844387076, 1.000000000000000000, 0.8660254037844387076, 1.000000000000000000, 0.8660254037844387076, 1.000000000000000000, 0.8660254037844387076, 1.000000000000000000, 0.8660254037844387076, 1.000000000000000000, 0.8660254037844387076, 1.000000000000000000, 0.8660254037844387076, 1.000000000000000000, 0.8660254037844387076, 1.000000000000000000, 0.8660254037844387076, 1.000000000000000000, 0.8660254037844387076, 1.000000000000000000, 0.8660254037844387076, 1.000000000000000000, 0.8660254037844387076, 1.000000000000000000, 0.8660254037844387076, 1.000000000000000000, 0.8660254037844387076, 1.000000000000000000, 0.8660254037844387076, 1.000000000000000000, 0.8660254037844387076, 1.000000000000000000, 0.8660254037844387076, 1.000000000000000000, 0.8660254037844387076, 1.000000000000000000, 0.8660254037844387076, 1.000000000000000000, 0.8660254037844387076, 1.000000000000000000, 0.8660254037844387076, 1.000000000000000000, 0.8660254037844387076, 1.000000000000000000, 0.8660254037844387076, 1.000000000000000000, 0.8660254037844387076, 1.000000000000000000, 0.8660254037844387076, 1.000000000000000000, 0.8660254037844387076, 1.000000000000000000, 0.8660254037844387076, 1.000000000000000000, 0.8660254037844387076, 1.000000000000000000, 0.8660254037844387076, 1.000000000000000000, 0.8660254037844387076, 1.000000000000000000, 0.8660254037844387076, 1.000000000000000000, 0.8660254037844387076, 1.000000000000000000, 0.8660254037844387076, 1.000000000000000000, 0.8660254037844387076, 1.000000000000000000, 0.8660254037844387076, 1.000000000000000000, 0.8660254037844387076, 1.000000000000000000, 0.8660254037844387076, 1.000000000000000000, 0.8660254037844387076, 1.000000000000000000, 0.8660254037844387076, 1.000000000000000000, 0.8660254037844387076, 1.000000000000000000, 0.8660254037844387076, 1.000000000000000000, 0.8660254037844387076, 1.000000000000000000, 0.8660254037844387076, 1.000000000000000000, 0.8660254037844387076, 1.000000000000000000, 0.8660254037844387076, 1.000000000000000000, 0.8660254037844387076, 1.000000000000000000, 0.8660254037844387076, 1.000000000000000000, 0.8660254037844387076, 1.000000000000000000, 0.8660254037844387076, 1.000000000000000000, 0.8660254037844387076, 1.000000000000000000, 0.8660254037844387076, 1.000000000000000000, 0.8660254037844387076, 1.000000000000000000, 0.8660254037844387076, 1.000000000000000000, 0.8660254037844387076, 1.000000000000000000, 0.8660254037844387076, 1.000000000000000000, 0.8660254037844387076, 1.000000000000000000, 0.8660254037844387076, 1.000000000000000000, 0.8660254037844387076, 1.000000000000000000, 0.8660254037844387076, 1.000000000000000000, 0.8660254037844387076, 1.000000000000000000, 0.8660254037844387076, 1.000000000000000000, 0.8660254037844387076, 1.000000000000000000, 0.8660254037844387076, 1.000000000000000000, 0.8660254037844387076, 1.000000000000000000, 0.8660254037844387076, 1.000000000000000000, 0.8660254037844387076, 1.000000000000000000, 0.8660254037844387076, 1.000000000000000000, 0.8660254037844387076, 1.000000000000000000, 0.8660254037844387076, 1.000000000000000000, 0.8660254037844387076, 1.000000000000000000, 0.8660254037844387076, 1.000000000000000000, 0.8660254037844387076, 1.000000000000000000, 0.8660254037844387076, 1.000000000000000000, 0.8660254037844387076, 1.000000000000000000, 0.8660254037844387076, 1.000000000000000000, 0.8660254037844387076, 1.000000000000000000, 0.8660254037844387076, 1.000000000000000000, 0.8660254037844387076, 1.000000000000000000, 0.8660254037844387076, 1.000000000000000000, 0.8660254037844387076, 1.000000000000000000, 0.8660254037844387076, 1.000000000000000000, 0.8660254037844387076, 1.000000000000000000, 0.8660254037844387076, 1.000000000000000000, 0.8660254037844387076, 1.000000000000000000, 0.8660254037844387076, 1.000000000000000000, 0.8660254037844387076, 1.000000000000000000, 0.8660254037844387076, 1.000000000000000000, 0.8660254037844387076, 1.000000000000000000, 0.8660254037844387076, 1.000000000000000000, 0.8660254037844387076, 1.000000000000000000, 0.8660254037844387076, 1.000000000000000000, 0.8660254037844387076, 1.000000000000000000, 0.8660254037844387076, 1.000000000000000000, 0.8660254037844387076, 1.000000000000000000, 0.8660254037844387076, 1.000000000000000000, 0.8660254037844387076, 1.000000000000000000, 0.8660254037844387076, 1.000000000000000000, 0.8660254037844387076, 1.000000000000000000, 0.8660254037844387076, 1.000000000000000000, 0.8660254037844387076, 1.000000000000000000, 0.8660254037844387076, 1.000000000000000000, 0.8660254037844387076, 1.000000000000000000, 0.8660254037844387076, 1.000000000000000000, 0.8660254037844387076, 1.000000000000000000, 0.8660254037844387076, 1.000000000000000000, 0.8660254037844387076, 1.000000000000000000, 0.8660254037844387076, 1.000000000000000000, 0.8660254037844387076, 1.000000000000000000, 0.8660254037844387076, 1.000000000000000000, 0.8660254037844387076, 1.000000000000000000, 0.8660254037844387076, 1.000000000000000000, 0.8660254037844387076, 1.000000000000000000, 0.8660254037844387076, 1.000000000000000000, 0.8660254037844387076, 1.000000000000000000, 0.8660254037844387076, 1.000000000000000000, 0.8660254037844387076, 1.000000000000000000, 0.8660254037844387076, 1.000000000000000000, 0.8660254037844387076, 1.000000000000000000, 0.8660254037844387076, 1.000000000000000000, 0.8660254037844387076, 1.000000000000000000, 0.8660254037844387076, 1.000000000000000000, 0.8660254037844387076, 1.000000000000000000, 0.8660254037844387076, 1.000000000000000000, 0.8660254037844387076, 1.000000000000000000, 0.8660254037844387076, 1.000000000000000000, 0.8660254037844387076, 1.000000000000000000, 0.8660254037844387076, 1.000000000000000000, 0.8660254037844387076, 1.000000000000000000, 0.8660254037844387076, 1.000000000000000000, 0.8660254037844387076, 1.000000000000000000, 0.8660254037844387076, 1.000000000000000000, 0.8660254037844387076, 1.000000000000000000, 0.8660254037844387076, 1.000000000000000000, 0.8660254037844387076, 1.000000000000000000, 0.8660254037844387076, 1.000000000000000000, 0.8660254037844387076, 1.000000000000000000, 0.8660254037844387076, 1.000000000000000000, 0.8660254037844387076, 1.000000000000000000, 0.8660254037844387076, 1.000000000000000000, 0.8660254037844387076, 1.000000000000000000, 0.8660254037844387076, 1.000000000000000000, 0.8660254037844387076, 1.000000000000000000, 0.8660254037844387076, 1.000000000000000000, 0.8660254037844387076, 1.000000000000000000, 0.8660254037844387076, 1.000000000000000000, 0.8660254037844387076, 1.000000000000000000, 0.8660254037844387076, 1.000000000000000000, 0.8660254037844387076, 1.000000000000000000, 0.8660254037844387076, 1.000000000000000000, 0.8660254037844387076, 1.000000000000000000, 0.8660254037844387076, 1.000000000000000000, 0.8660254037844387076, 1.000000000000000000, 0.8660254037844387076, 1.000000000000000000, 0.8660254037844387076, 1.000000000000000000, 0.8660254037844387076, 1.000000000000000000, 0.8660254037844387076, 1.000000000000000000, 0.8660254037844387076, 1.000000000000000000, 0.8660254037844387076, 1.000000000000000000, 0.8660254037844387076, 1.000000000000000000, 0.8660254037844387076, 1.000000000000000000, 0.8660254037844387076, 1.000000000000000000, 0.8660254037844387076, 1.000000000000000000, 0.8660254037844387076, 1.000000000000000000, 0.8660254037844387076, 1.000000000000000000, 0.8660254037844387076, 1.000000000000000000, 0.8660254037844387076, 1.000000000000000000, 0.8660254037844387076, 1.000000000000000000, 0.8660254037844387076, 1.000000000000000000, 0.8660254037844387076, 1.000000000000000000, 0.8660254037844387076, 1.000000000000000000, 0.8660254037844387076, 1.000000000000000000, 0.8660254037844387076, 1.000000000000000000, 0.8660254037844387076, 1.000000000000000000, 0.8660254037844387076, 1.000000000000000000, 0.8660254037844387076, 1.000000000000000000, 0.8660254037844387076, 1.000000000000000000, 0.8660254037844387076, 1.000000000000000000, 0.8660254037844387076, 1.000000000000000000, 0.8660254037844387076, 1.000000000000000000, 0.8660254037844387076, 1.000000000000000000, 0.8660254037844387076, 1.000000000000000000, 0.8660254037844387076, 1.000000000000000000, 0.8660254037844387076, 1.000000000000000000, 0.8660254037844387076, 1.000000000000000000, 0.8660254037844387076, 1.000000000000000000, 0.8660254037844387076, 1.000000000000000000, 0.8660254037844387076, 1.000000000000000000, 0.8660254037844387076, 1.000000000000000000, 0.8660254037844387076, 1.000000000000000000, 0.8660254037844387076, 1.000000000000000000, 0.8660254037844387076, 1.000000000000000000, 0.8660254037844387076, 1.000000000000000000, 0.8660254037844387076, 1.000000000000000000, 0.8660254037844387076, 1.000000000000000000, 0.8660254037844387076, 1.000000000000000000, 0.8660254037844387076, 1.000000000000000000, 0.8660254037844387076, 1.000000000000000000, 0.8660254037844387076, 1.000000000000000000, 0.8660254037844387076, 1.000000000000000000, 0.8660254037844387076, 1.000000000000000000, 0.8660254037844387076, 1.000000000000000000, 0.8660254037844387076, 1.000000000000000000, 0.8660254037844387076, 1.000000000000000000, 0.8660254037844387076, 1.000000000000000000, 0.8660254037844387076, 1.000000000000000000, 0.8660254037844387076, 1.000000000000000000, 0.8660254037844387076, 1.000000000000000000, 0.8660254037844387076, 1.000000000000000000, 0.8660254037844387076, 1.000000000000000000, 0.8660254037844387076, 1.000000000000000000, 0.8660254037844387076, 1.000000000000000000, 0.8660254037844387076, 1.000000000000000000, 0.8660254037844387076, 1.000000000000000000, 0.8660254037844387076, 1.000000000000000000, 0.8660254037844387076, 1.000000000000000000, 0.8660254037844387076, 1.000000000000000000, 0.8660254037844387076, 1.000000000000000000, 0.8660254037844387076, 1.000000000000000000, 0.8660254037844387076, 1.000000000000000000, 0.8660254037844387076, 1.000000000000000000, 0.8660254037844387076, 1.000000000000000000, 0.8660254037844387076, 1.000000000000000000, 0.8660254037844387076, 1.000000000000000000, 0.8660254037844387076, 1.000000000000000000, 0.8660254037844387076, 1.000000000000000000, 0.8660254037844387076, 1.000000000000000000, 0.8660254037844387076, 1.000000000000000000, 0.8660254037844387076, 1.000000000000000000, 0.8660254037844387076, 1.000000000000000000, 0.8660254037844387076, 1.000000000000000000, 0.8660254037844387076, 1.000000000000000000, 0.8660254037844387076, 1.000000000000000000, 0.8660254037844387076, 1.000000000000000000, 0.8660254037844387076, 1.000000000000000000, 0.8660254037844387076, 1.000000000000000000, 0.8660254037844387076, 1.000000000000000000, 0.8660254037844387076, 1.000000000000000000, 0.8660254037844387076, 1.000000000000000000, 0.8660254037844387076, 1.000000000000000000, 0.8660254037844387076, 1.000000000000000000, 0.8660254037844387076, 1.000000000000000000, 0.8660254037844387076, 1.000000000000000000, 0.8660254037844387076, 1.000000000000000000, 0.8660254037844387076, 1.000000000000000000, 0.8660254037844387076, 1.000000000000000000, 0.8660254037844387076, 1.000000000000000000, 0.8660254037844387076, 1.000000000000000000, 0.8660254037844387076, 1.000000000000000000, 0.8660254037844387076, 1.000000000000000000, 0.8660254037844387076, 1.000000000000000000, 0.8660254037844387076, 1.000000000000000000, 0.8660254037844387076, 1.000000000000000000, 0.8660254037844387076, 1.000000000000000000, 0.8660254037844387076, 1.000000000000000000, 0.8660254037844387076, 1.000000000000000000, 0.8660254037844387076, 1.000000000000000000, 0.8660254037844387076, 1.000000000000000000, 0.8660254037844387076, 1.000000000000000000, 0.8660254037844387076, 1.000000000000000000, 0.8660254037844387076, 1.000000000000000000, 0.8660254037844387076, 1.000000000000000000, 0.8660254037844387076, 1.000000000000000000, 0.8660254037844387076, 1.000000000000000000, 0.8660254037844387076, 1.000000000000000000, 0.8660254037844387076, 1.000000000000000000, 0.8660254037844387076, 1.000000000000000000, 0.8660254037844387076, 1.000000000000000000, 0.8660254037844387076, 1.000000000000000000, 0.8660254037844387076, 1.000000000000000000, 0.8660254037844387076, 1.000000000000000000, 0.8660254037844387076, 1.000000000000000000, 0.8660254037844387076, 1.000000000000000000, 0.8660254037844387076, 1.000000000000000000, 0.8660254037844387076, 1.000000000000000000, 0.8660254037844387076, 1.000000000000000000, 0.8660254037844387076, 1.000000000000000000, 0.8660254037844387076, 1.000000000000000000, 0.8660254037844387076, 1.000000000000000000, 0.8660254037844387076, 1.000000000000000000, 0.8660254037844387076, 1.000000000000000000, 0.8660254037844387076, 1.000000000000000000, 0.8660254037844387076, 1.000000000000000000, 0.8660254037844387076, 1.000000000000000000, 0.8660254037844387076, 1.000000000000000000, 0.8660254037844387076, 1.000000000000000000, 0.8660254037844387076, 1.000000000000000000, 0.8660254037844387076, 1.000000000000000000, 0.8660254037844387076, 1.000000000000000000, 0.8660254037844387076, 1.000000000000000000, 0.8660254037844387076, 1.000000000000000000, 0.8660254037844387076, 1.000000000000000000, 0.8660254037844387076, 1.000000000000000000, 0.8660254037844387076, 1.000000000000000000, 0.8660254037844387076, 1.000000000000000000, 0.8660254037844387076, 1.000000000000000000, 0.8660254037844387076, 1.000000000000000000, 0.8660254037844387076, 1.000000000000000000, 0.8660254037844387076, 1.000000000000000000 ) ) 
 REPRESENTATION_ITEM ( '' )  );
#40682=CARTESIAN_POINT ( 'NONE',  ( 17.10000000000000142, -4.330127018922190985, -2.500000000000001332 ) ) ;
#40685=AXIS2_PLACEMENT_3D ( 'NONE', #5165, #16594, #39147 ) ;
#40687=CARTESIAN_POINT ( 'NONE',  ( 22.92187500061451644, 4.119189519843966529, 2.378215178124999607 ) ) ;
#40694=CARTESIAN_POINT ( 'NONE',  ( 24.90937500061451004, -5.492252693125287522, -1.008910452111647106E-15 ) ) ;
#40697=CARTESIAN_POINT ( 'NONE',  ( 11.70937500061451608, 2.746126346562643317, 4.756430356249998326 ) ) ;
#40700=VERTEX_POINT ( 'NONE', #3614 ) ;
#40705=CARTESIAN_POINT ( 'NONE',  ( 29.69999999999999574, -4.330127018922190985, -2.500000000000001332 ) ) ;
#40706=CARTESIAN_POINT ( 'NONE',  ( 15.90000000000000036, 4.330127018922192761, -2.499999999999997780 ) ) ;
#40709=CARTESIAN_POINT ( 'NONE',  ( 12.90937500061451537, 2.746126346562645981, -4.756430356249997438 ) ) ;
#40721=AXIS2_PLACEMENT_3D ( 'NONE', #68631, #18718, #46823 ) ;
#40722=VERTEX_POINT ( 'NONE', #13949 ) ;
#40728=CARTESIAN_POINT ( 'NONE',  ( 12.16875000122903394, -5.773502691896255534, -1.060575238724906372E-15 ) ) ;
#40731=CARTESIAN_POINT ( 'NONE',  ( 21.94687500061451502, -2.746126346562641984, -4.756430356249999214 ) ) ;
#40749=CARTESIAN_POINT ( 'NONE',  ( 21.26249999999999574, 2.886751345948129099, -4.999999999999997335 ) ) ;
#40752=CARTESIAN_POINT ( 'NONE',  ( 17.04375000122903216, -2.886751345948129988, 4.999999999999997335 ) ) ;
#40761=CARTESIAN_POINT ( 'NONE',  ( 10.80000000000000071, -4.330127018922190985, -2.500000000000001332 ) ) ;
#40769=CARTESIAN_POINT ( 'NONE',  ( 22.92187500061451644, 2.746126346562645981, -4.756430356249997438 ) ) ;
#40774=CARTESIAN_POINT ( 'NONE',  ( 24.89999999999999858, 4.330127018922192761, -2.499999999999997780 ) ) ;
#40778=CARTESIAN_POINT ( 'NONE',  ( 12.88125000122903430, 4.330127018922191873, 2.499999999999999556 ) ) ;
#40780=CARTESIAN_POINT ( 'NONE',  ( 24.60000000000000142, 0.000000000000000000, 4.999999999999998224 ) ) ;
#40785=CARTESIAN_POINT ( 'NONE',  ( 10.18125000122903323, 4.330127018922191873, 2.499999999999999556 ) ) ;
#40788=CARTESIAN_POINT ( 'NONE',  ( 18.19687500061451502, -4.119189519843965641, -2.378215178125001383 ) ) ;
#40790=AXIS2_PLACEMENT_3D ( 'NONE', #32980, #28177, #4914 ) ;
#40800=CARTESIAN_POINT ( 'NONE',  ( 11.59687500061451537, 4.119189519843966529, -2.378215178124998275 ) ) ;
#40806=EDGE_LOOP ( 'NONE', ( #66995, #34438, #39917, #25454 ) ) ;
#40813=CARTESIAN_POINT ( 'NONE',  ( 9.449999999999999289, -4.330127018922190985, -2.500000000000001332 ) ) ;
#40822=CARTESIAN_POINT ( 'NONE',  ( 29.07187500061451502, -5.492252693125287522, -1.008910452111647106E-15 ) ) ;
#40824=CARTESIAN_POINT ( 'NONE',  ( 28.58437500061451431, -2.746126346562641984, -4.756430356249999214 ) ) ;
#40825=CARTESIAN_POINT ( 'NONE',  ( 13.95937500061451786, 4.119189519843966529, -2.378215178124998275 ) ) ;
#40842=CARTESIAN_POINT ( 'NONE',  ( 22.85625000122903216, 0.000000000000000000, 4.999999999999998224 ) ) ;
#40851=( BOUNDED_CURVE ( )  B_SPLINE_CURVE ( 2, ( #33056, #67419, #49695, #50424, #38975, #39339, #33781 ),
 .UNSPECIFIED., .F., .F. ) 
 B_SPLINE_CURVE_WITH_KNOTS ( ( 3, 2, 2, 3 ),
 ( 0.6900000000000000577, 0.6933333333333334680, 0.6966666666666668783, 0.7000000000000001776 ),
 .UNSPECIFIED. ) 
 CURVE ( )  GEOMETRIC_REPRESENTATION_ITEM ( )  RATIONAL_B_SPLINE_CURVE ( ( 0.9999999999999955591, 0.8660254037844431485, 1.000000000000000000, 0.8660254037844387076, 1.000000000000000000, 0.8660254037844298258, 1.000000000000008882 ) ) 
 REPRESENTATION_ITEM ( '' )  );
#40868=CARTESIAN_POINT ( 'NONE',  ( 14.69999999999999929, 0.000000000000000000, 4.999999999999998224 ) ) ;
#40877=VECTOR ( 'NONE', #45055, 1000.000000000000000 ) ;
#40889=( BOUNDED_CURVE ( )  B_SPLINE_CURVE ( 2, ( #35249, #34521, #13070, #7180, #18964, #41524, #35972 ),
 .UNSPECIFIED., .F., .F. ) 
 B_SPLINE_CURVE_WITH_KNOTS ( ( 3, 2, 2, 3 ),
 ( 0.9100000000000000311, 0.9133333333333333304, 0.9166666666666667407, 0.9200000000000001510 ),
 .UNSPECIFIED. ) 
 CURVE ( )  GEOMETRIC_REPRESENTATION_ITEM ( )  RATIONAL_B_SPLINE_CURVE ( ( 1.000000000000000000, 0.8660254037844387076, 1.000000000000000000, 0.8660254037844387076, 1.000000000000000000, 0.8660254037844342667, 1.000000000000004441 ) ) 
 REPRESENTATION_ITEM ( '' )  );
#40891=EDGE_CURVE ( 'NONE', #9764, #72010, #40663, .T. ) ;
#40892=ORIENTED_EDGE ( 'NONE', *, *, #56668, .T. ) ;
#40895=CARTESIAN_POINT ( 'NONE',  ( 18.57187500061451857, -4.119189519843968306, 2.378215178124996054 ) ) ;
#40897=ADVANCED_FACE ( 'NONE', ( #70103 ), #37217, .T. ) ;
#40913=CARTESIAN_POINT ( 'NONE',  ( 11.26875000122903181, -5.773502691896255534, -1.060575238724906372E-15 ) ) ;
#40914=CARTESIAN_POINT ( 'NONE',  ( 20.89687500061452141, -2.746126346562646425, 4.756430356249996549 ) ) ;
#40935=DIRECTION ( 'NONE',  ( -1.000000000000000000, -0.000000000000000000, -0.000000000000000000 ) ) ;
#40943=CARTESIAN_POINT ( 'NONE',  ( 45.00000000000000000, 0.000000000000000000, 0.000000000000000000 ) ) ;
#40946=EDGE_LOOP ( 'NONE', ( #65492, #34893, #10986, #70681 ) ) ;
#40947=ORIENTED_EDGE ( 'NONE', *, *, #37794, .T. ) ;
#40957=CARTESIAN_POINT ( 'NONE',  ( 10.20937500061451786, -4.119189519843965641, -2.378215178125001383 ) ) ;
#40959=CARTESIAN_POINT ( 'NONE',  ( 20.34375000122903643, -2.886751345948098013, -5.000000000000047073 ) ) ;
#40976=CARTESIAN_POINT ( 'NONE',  ( 18.60937500061451289, -5.492252693125287522, -1.008910452111647106E-15 ) ) ;
#40979=CARTESIAN_POINT ( 'NONE',  ( 25.84687500061451360, -4.119189519843965641, -2.378215178125001383 ) ) ;
#40986=CARTESIAN_POINT ( 'NONE',  ( 21.88125000122903074, 4.330127018922191873, 2.499999999999999556 ) ) ;
#40994=CARTESIAN_POINT ( 'NONE',  ( 26.55937500061451573, 4.119189519843966529, -2.378215178124998275 ) ) ;
#40998=CARTESIAN_POINT ( 'NONE',  ( 45.00000000000000000, 6.123233995736764310E-16, -4.999999999999998224 ) ) ;
#41013=CARTESIAN_POINT ( 'NONE',  ( 14.40937500061451715, 4.119189519843966529, -2.378215178124998275 ) ) ;
#41025=CARTESIAN_POINT ( 'NONE',  ( 34.99999999999999289, -2.499999999999999556, 3.499999999999999556 ) ) ;
#41026=ORIENTED_EDGE ( 'NONE', *, *, #17437, .T. ) ;
#41040=ORIENTED_EDGE ( 'NONE', *, *, #43153, .T. ) ;
#41044=CARTESIAN_POINT ( 'NONE',  ( 15.27187500061451786, 2.746126346562645981, -4.756430356249997438 ) ) ;
#41051=CARTESIAN_POINT ( 'NONE',  ( 18.33749999999999858, -2.886751345948129988, 4.999999999999997335 ) ) ;
#41055=CARTESIAN_POINT ( 'NONE',  ( 23.48437500061451289, -2.746126346562646425, 4.756430356249996549 ) ) ;
#41062=CARTESIAN_POINT ( 'NONE',  ( 24.57187500061451502, 5.824947211148865298E-16, -4.756430356249998326 ) ) ;
#41064=CARTESIAN_POINT ( 'NONE',  ( 11.55937500061451573, 2.746126346562645981, -4.756430356249997438 ) ) ;
#41076=CARTESIAN_POINT ( 'NONE',  ( 11.67187500061451644, 4.119189519843966529, 2.378215178124999607 ) ) ;
#41079=EDGE_CURVE ( 'NONE', #36820, #16786, #33525, .T. ) ;
#41096=CARTESIAN_POINT ( 'NONE',  ( 21.12187500061451573, 2.746126346562645981, -4.756430356249997438 ) ) ;
#41103=ORIENTED_EDGE ( 'NONE', *, *, #56240, .T. ) ;
#41113=CARTESIAN_POINT ( 'NONE',  ( 21.30000000000000071, 4.330127018922192761, -2.499999999999997780 ) ) ;
#41127=( BOUNDED_CURVE ( )  B_SPLINE_CURVE ( 2, ( #37535, #54170, #31998, #30893, #8728, #26090, #25353 ),
 .UNSPECIFIED., .F., .F. ) 
 B_SPLINE_CURVE_WITH_KNOTS ( ( 3, 2, 2, 3 ),
 ( 0.5999999999999999778, 0.6033333333333334991, 0.6066666666666667984, 0.6100000000000002087 ),
 .UNSPECIFIED. ) 
 CURVE ( )  GEOMETRIC_REPRESENTATION_ITEM ( )  RATIONAL_B_SPLINE_CURVE ( ( 1.000000000000000000, 0.8660254037844387076, 1.000000000000000000, 0.8660254037844387076, 1.000000000000000000, 0.8660254037844298258, 1.000000000000008882 ) ) 
 REPRESENTATION_ITEM ( '' )  );
#41132=CARTESIAN_POINT ( 'NONE',  ( 22.54687500061451999, 5.492252693125287522, 3.363034840372157021E-16 ) ) ;
#41138=CARTESIAN_POINT ( 'NONE',  ( 25.12499999999999645, -4.330127018922194537, 2.499999999999995559 ) ) ;
#41148=CARTESIAN_POINT ( 'NONE',  ( 9.881250001229032520, -4.330127018922194537, 2.499999999999995559 ) ) ;
#41151=CARTESIAN_POINT ( 'NONE',  ( 18.08437500061451075, -2.746126346562646425, 4.756430356249996549 ) ) ;
#41154=ORIENTED_EDGE ( 'NONE', *, *, #25568, .T. ) ;
#41162=CARTESIAN_POINT ( 'NONE',  ( 9.796875000614514661, 4.119189519843966529, -2.378215178124998275 ) ) ;
#41168=ADVANCED_FACE ( 'NONE', ( #47900 ), #58596, .T. ) ;
#41170=CARTESIAN_POINT ( 'NONE',  ( 19.83750000000000213, -2.886751345948126435, -5.000000000000000000 ) ) ;
#41173=CARTESIAN_POINT ( 'NONE',  ( 28.35937500061451644, 2.746126346562643317, 4.756430356249998326 ) ) ;
#41176=CARTESIAN_POINT ( 'NONE',  ( 10.98750000000000071, 5.773502691896255534, 3.535250795749688894E-16 ) ) ;
#41184=CARTESIAN_POINT ( 'NONE',  ( 28.47187500061451715, 2.746126346562643317, 4.756430356249998326 ) ) ;
#41186=CARTESIAN_POINT ( 'NONE',  ( 28.50937500061451502, -5.492252693125287522, -1.008910452111647106E-15 ) ) ;
#41187=CARTESIAN_POINT ( 'NONE',  ( 10.62187500061451928, -5.492252693125287522, -1.008910452111647106E-15 ) ) ;
#41202=CARTESIAN_POINT ( 'NONE',  ( 23.60625000122903216, 4.330127018922192761, -2.499999999999997780 ) ) ;
#41240=CARTESIAN_POINT ( 'NONE',  ( 28.08749999999999858, 5.773502691896255534, 3.535250795749688401E-16 ) ) ;
#41251=CARTESIAN_POINT ( 'NONE',  ( 17.74687500061451928, -4.119189519843965641, -2.378215178125001383 ) ) ;
#41267=CARTESIAN_POINT ( 'NONE',  ( 8.343750001229034652, 5.773502691896255534, 3.535250795749688401E-16 ) ) ;
#41270=CARTESIAN_POINT ( 'NONE',  ( 19.24687500061452283, -2.746126346562642428, -4.756430356249999214 ) ) ;
#41273=( BOUNDED_CURVE ( )  B_SPLINE_CURVE ( 2, ( #28562, #22646, #72177, #4587, #45196, #33377, #21557 ),
 .UNSPECIFIED., .F., .F. ) 
 B_SPLINE_CURVE_WITH_KNOTS ( ( 3, 2, 2, 3 ),
 ( 0.1200000000000000788, 0.1233333333333334059, 0.1266666666666667329, 0.1300000000000000322 ),
 .UNSPECIFIED. ) 
 CURVE ( )  GEOMETRIC_REPRESENTATION_ITEM ( )  RATIONAL_B_SPLINE_CURVE ( ( 0.9999999999999966693, 0.8660254037844420383, 1.000000000000000000, 0.8660254037844387076, 1.000000000000000000, 0.8660254037844375974, 1.000000000000001110 ) ) 
 REPRESENTATION_ITEM ( '' )  );
#41282=DIRECTION ( 'NONE',  ( -1.000000000000000000, -0.000000000000000000, -0.000000000000000000 ) ) ;
#41283=ORIENTED_EDGE ( 'NONE', *, *, #10973, .F. ) ;
#41289=CARTESIAN_POINT ( 'NONE',  ( 20.90625000122903288, 4.330127018922192761, -2.499999999999997780 ) ) ;
#41292=CARTESIAN_POINT ( 'NONE',  ( 45.00000000000000000, 0.000000000000000000, 0.000000000000000000 ) ) ;
#41313=CARTESIAN_POINT ( 'NONE',  ( 28.03125000122903288, 6.123233995736764310E-16, -4.999999999999998224 ) ) ;
#41314=CARTESIAN_POINT ( 'NONE',  ( 28.61249999999999716, 2.886751345948126879, 4.999999999999999112 ) ) ;
#41321=CARTESIAN_POINT ( 'NONE',  ( 28.93125000122903145, 6.123233995736764310E-16, -4.999999999999998224 ) ) ;
#41324=CARTESIAN_POINT ( 'NONE',  ( 15.46875000122903110, 2.886751345948129099, -4.999999999999997335 ) ) ;
#41327=EDGE_CURVE ( 'NONE', #12847, #45106, #42356, .T. ) ;
#41334=CARTESIAN_POINT ( 'NONE',  ( 15.94687500061451502, -4.119189519843965641, -2.378215178125001383 ) ) ;
#41337=CARTESIAN_POINT ( 'NONE',  ( 25.28437500061451360, -2.746126346562646425, 4.756430356249996549 ) ) ;
#41344=CARTESIAN_POINT ( 'NONE',  ( 28.21875000122902932, 2.886751345948148195, 4.999999999999962697 ) ) ;
#41352=CARTESIAN_POINT ( 'NONE',  ( 28.20937500061451786, -4.119189519843965641, -2.378215178125001383 ) ) ;
#41355=CARTESIAN_POINT ( 'NONE',  ( 25.27499999999999858, 6.123233995736764310E-16, -4.999999999999998224 ) ) ;
#41361=ORIENTED_EDGE ( 'NONE', *, *, #64577, .T. ) ;
#41370=CARTESIAN_POINT ( 'NONE',  ( 11.85937500061451644, 0.000000000000000000, 4.756430356249998326 ) ) ;
#41383=ORIENTED_EDGE ( 'NONE', *, *, #35460, .F. ) ;
#41396=EDGE_CURVE ( 'NONE', #47145, #19210, #45845, .T. ) ;
#41400=CARTESIAN_POINT ( 'NONE',  ( 15.49687500061451750, -2.746126346562646425, 4.756430356249996549 ) ) ;
#41406=CARTESIAN_POINT ( 'NONE',  ( 18.52499999999999858, 6.123233995736764310E-16, -4.999999999999998224 ) ) ;
#41410=CARTESIAN_POINT ( 'NONE',  ( 22.50937500061451502, 2.746126346562643317, 4.756430356249998326 ) ) ;
#41413=DIRECTION ( 'NONE',  ( -1.000000000000000000, -0.000000000000000000, -0.000000000000000000 ) ) ;
#41418=CARTESIAN_POINT ( 'NONE',  ( 25.39687500061451431, -4.119189519843965641, -2.378215178125001383 ) ) ;
#41420=CARTESIAN_POINT ( 'NONE',  ( 7.884375000614516793, -2.746126346562641984, -4.756430356249999214 ) ) ;
#41423=ORIENTED_EDGE ( 'NONE', *, *, #60032, .T. ) ;
#41425=CARTESIAN_POINT ( 'NONE',  ( 9.956250001229033586, -4.330127018922190985, -2.500000000000001332 ) ) ;
#41429=CARTESIAN_POINT ( 'NONE',  ( 29.77499999999999858, 6.123233995736764310E-16, -4.999999999999998224 ) ) ;
#41432=CARTESIAN_POINT ( 'NONE',  ( 11.70937500061451608, 2.746126346562643317, 4.756430356249998326 ) ) ;
#41448=CARTESIAN_POINT ( 'NONE',  ( 11.32500000000000107, 6.123233995736764310E-16, -4.999999999999998224 ) ) ;
#41450=CARTESIAN_POINT ( 'NONE',  ( 19.47187500061451360, 2.746126346562643317, 4.756430356249998326 ) ) ;
#41467=CARTESIAN_POINT ( 'NONE',  ( 28.49999999999999645, 4.330127018922192761, -2.499999999999997780 ) ) ;
#41471=CARTESIAN_POINT ( 'NONE',  ( 45.00000000000000000, 0.000000000000000000, 0.000000000000000000 ) ) ;
#41481=ORIENTED_EDGE ( 'NONE', *, *, #55095, .T. ) ;
#41484=CARTESIAN_POINT ( 'NONE',  ( 24.38437500061451502, 4.119189519843966529, 2.378215178124999607 ) ) ;
#41490=CARTESIAN_POINT ( 'NONE',  ( 24.63749999999999574, -2.886751345948129988, 4.999999999999997335 ) ) ;
#41496=PRODUCT_DEFINITION_FORMATION_WITH_SPECIFIED_SOURCE ( 'ANY', '', #9598, .NOT_KNOWN. ) ;
#41499=CARTESIAN_POINT ( 'NONE',  ( 10.59375000122903465, 5.773502691896255534, 3.535250795749688894E-16 ) ) ;
#41502=CARTESIAN_POINT ( 'NONE',  ( 15.23437500061451644, 5.492252693125287522, 3.363034840372157021E-16 ) ) ;
#41509=DIRECTION ( 'NONE',  ( -1.000000000000000000, -0.000000000000000000, -0.000000000000000000 ) ) ;
#41515=CARTESIAN_POINT ( 'NONE',  ( 10.32187500061451679, 4.119189519843966529, 2.378215178124999607 ) ) ;
#41524=CARTESIAN_POINT ( 'NONE',  ( 8.943750001229032520, -2.886751345948074920, 5.000000000000092371 ) ) ;
#41526=CARTESIAN_POINT ( 'NONE',  ( 27.79687500061451289, 4.119189519843966529, -2.378215178124998275 ) ) ;
#41529=CARTESIAN_POINT ( 'NONE',  ( 8.512499999999999289, -5.773502691896255534, -1.060575238724906372E-15 ) ) ;
#41532=ORIENTED_EDGE ( 'NONE', *, *, #27801, .F. ) ;
#41535=EDGE_CURVE ( 'NONE', #45117, #67338, #8729, .T. ) ;
#41538=CARTESIAN_POINT ( 'NONE',  ( 26.44687500061451502, -2.746126346562641984, -4.756430356249999214 ) ) ;
#41540=CARTESIAN_POINT ( 'NONE',  ( 27.30937500061451217, 2.746126346562645981, -4.756430356249997438 ) ) ;
#41541=CARTESIAN_POINT ( 'NONE',  ( 10.05937500061451750, 0.000000000000000000, 4.756430356249998326 ) ) ;
#41556=CARTESIAN_POINT ( 'NONE',  ( 20.71875000122903288, -5.773502691896255534, -1.060575238724906372E-15 ) ) ;
#41588=CARTESIAN_POINT ( 'NONE',  ( 19.44375000122903430, -2.886751345948126435, -5.000000000000000000 ) ) ;
#41603=VERTEX_POINT ( 'NONE', #65239 ) ;
#41607=CARTESIAN_POINT ( 'NONE',  ( 15.87187500061451573, -4.119189519843968306, 2.378215178124996054 ) ) ;
#41623=CYLINDRICAL_SURFACE ( 'NONE', #56384, 4.999999999999998224 ) ;
#41625=CARTESIAN_POINT ( 'NONE',  ( 18.12187500061451573, 2.746126346562643317, 4.756430356249998326 ) ) ;
#41629=EDGE_CURVE ( 'NONE', #58973, #54880, #14628, .T. ) ;
#41636=DIRECTION ( 'NONE',  ( -1.000000000000000000, -0.000000000000000000, -0.000000000000000000 ) ) ;
#41643=CARTESIAN_POINT ( 'NONE',  ( 27.50625000122903074, -4.330127018922190985, -2.500000000000001332 ) ) ;
#41647=CARTESIAN_POINT ( 'NONE',  ( 14.92500000000000071, 6.123233995736764310E-16, -4.999999999999998224 ) ) ;
#41655=ORIENTED_EDGE ( 'NONE', *, *, #41965, .T. ) ;
#41668=CARTESIAN_POINT ( 'NONE',  ( 7.546875000614517326, -2.746126346562642428, -4.756430356249999214 ) ) ;
#41674=CARTESIAN_POINT ( 'NONE',  ( 28.70625000122903003, 0.000000000000000000, 4.999999999999998224 ) ) ;
#41686=CARTESIAN_POINT ( 'NONE',  ( 14.93437500061451573, -2.746126346562646425, 4.756430356249996549 ) ) ;
#41689=CARTESIAN_POINT ( 'NONE',  ( 22.77187500061451431, 5.824947211148865298E-16, -4.756430356249998326 ) ) ;
#41704=CARTESIAN_POINT ( 'NONE',  ( 24.04687500061451644, -2.746126346562646425, 4.756430356249996549 ) ) ;
#41708=CARTESIAN_POINT ( 'NONE',  ( 18.89999999999999858, -4.330127018922190985, -2.500000000000001332 ) ) ;
#41723=CARTESIAN_POINT ( 'NONE',  ( 13.47187500061451537, 2.746126346562645981, -4.756430356249997438 ) ) ;
#41736=VERTEX_POINT ( 'NONE', #37902 ) ;
#41753=CARTESIAN_POINT ( 'NONE',  ( 13.54687500061451999, 5.492252693125287522, 3.363034840372157021E-16 ) ) ;
#41759=CARTESIAN_POINT ( 'NONE',  ( 14.92500000000000071, 6.123233995736764310E-16, -4.999999999999998224 ) ) ;
#41762=AXIS2_PLACEMENT_3D ( 'NONE', #32412, #9516, #54219 ) ;
#41764=CARTESIAN_POINT ( 'NONE',  ( 22.17187500061451644, -4.119189519843968306, 2.378215178124996054 ) ) ;
#41765=ORIENTED_EDGE ( 'NONE', *, *, #17437, .F. ) ;
#41772=CARTESIAN_POINT ( 'NONE',  ( 21.49687500061451573, 4.119189519843966529, -2.378215178124998275 ) ) ;
#41774=CARTESIAN_POINT ( 'NONE',  ( 7.621875000614515727, 4.119189519843966529, 2.378215178124999607 ) ) ;
#41784=CARTESIAN_POINT ( 'NONE',  ( 11.10937500061451821, 2.746126346562645981, -4.756430356249997438 ) ) ;
#41803=DIRECTION ( 'NONE',  ( 0.000000000000000000, 0.000000000000000000, 1.000000000000000000 ) ) ;
#41805=CARTESIAN_POINT ( 'NONE',  ( 19.69687500061451857, -2.746126346562641984, -4.756430356249999214 ) ) ;
#41825=EDGE_CURVE ( 'NONE', #44291, #3324, #48213, .T. ) ;
#41837=VECTOR ( 'NONE', #36343, 1000.000000000000000 ) ;
#41842=CARTESIAN_POINT ( 'NONE',  ( 20.40937500061451715, 0.000000000000000000, 4.756430356249998326 ) ) ;
#41849=CARTESIAN_POINT ( 'NONE',  ( 25.23749999999999716, -2.886751345948125991, -5.000000000000000000 ) ) ;
#41851=LINE ( 'NONE', #20030, #50233 ) ;
#41853=CARTESIAN_POINT ( 'NONE',  ( 11.83125000122903181, 6.123233995736764310E-16, -4.999999999999998224 ) ) ;
#41856=CARTESIAN_POINT ( 'NONE',  ( 18.16875000122903216, 2.886751345948129099, -4.999999999999997335 ) ) ;
#41858=CARTESIAN_POINT ( 'NONE',  ( 7.743750001229034119, -2.886751345948125991, -5.000000000000000000 ) ) ;
#41860=CARTESIAN_POINT ( 'NONE',  ( 15.72187500061451537, 4.119189519843966529, 2.378215178124999607 ) ) ;
#41863=ORIENTED_EDGE ( 'NONE', *, *, #48670, .T. ) ;
#41873=CARTESIAN_POINT ( 'NONE',  ( 10.39687500061451608, 0.000000000000000000, 4.756430356249998326 ) ) ;
#41879=VECTOR ( 'NONE', #10638, 1000.000000000000227 ) ;
#41880=ORIENTED_EDGE ( 'NONE', *, *, #17845, .F. ) ;
#41885=CARTESIAN_POINT ( 'NONE',  ( 29.55937500061451217, 2.746126346562645981, -4.756430356249997438 ) ) ;
#41888=CARTESIAN_POINT ( 'NONE',  ( 8.400000000000000355, 0.000000000000000000, 4.999999999999998224 ) ) ;
#41892=ORIENTED_EDGE ( 'NONE', *, *, #45595, .F. ) ;
#41897=CARTESIAN_POINT ( 'NONE',  ( 25.77187500061451431, 2.746126346562643317, 4.756430356249998326 ) ) ;
#41899=CARTESIAN_POINT ( 'NONE',  ( 10.88437500061451679, 4.119189519843966529, 2.378215178124999607 ) ) ;
#41917=CARTESIAN_POINT ( 'NONE',  ( 21.31875000122903430, 2.886751345948129099, -4.999999999999998224 ) ) ;
#41932=CARTESIAN_POINT ( 'NONE',  ( 29.67187500061451644, 2.746126346562645981, -4.756430356249997438 ) ) ;
#41940=VECTOR ( 'NONE', #25980, 1000.000000000000000 ) ;
#41965=EDGE_CURVE ( 'NONE', #66756, #67375, #53381, .T. ) ;
#41969=( BOUNDED_CURVE ( )  B_SPLINE_CURVE ( 2, ( #60655, #33327, #20772, #72123, #66961, #55139, #16327 ),
 .UNSPECIFIED., .F., .T. ) 
 B_SPLINE_CURVE_WITH_KNOTS ( ( 3, 2, 2, 3 ),
 ( 0.4700000000000001399, 0.4733333333333334392, 0.4766666666666666829, 0.4799999999999999267 ),
 .UNSPECIFIED. ) 
 CURVE ( )  GEOMETRIC_REPRESENTATION_ITEM ( )  RATIONAL_B_SPLINE_CURVE ( ( 0.9999999999999933387, 0.8660254037844453689, 1.000000000000000000, 0.8660254037844387076, 1.000000000000000000, 0.8660254037844409281, 0.9999999999999977796 ) ) 
 REPRESENTATION_ITEM ( '' )  );
#41971=CARTESIAN_POINT ( 'NONE',  ( 25.83749999999999503, 5.773502691896255534, 3.535250795749688401E-16 ) ) ;
#41974=CARTESIAN_POINT ( 'NONE',  ( 16.58437500061451431, 5.492252693125287522, 3.363034840372157021E-16 ) ) ;
#41983=ORIENTED_EDGE ( 'NONE', *, *, #40580, .T. ) ;
#41990=CARTESIAN_POINT ( 'NONE',  ( 25.96875000122903998, 2.886751345948113556, 5.000000000000023093 ) ) ;
#41992=CARTESIAN_POINT ( 'NONE',  ( 45.00000000000000000, 6.123233995736764310E-16, -4.999999999999998224 ) ) ;
#41995=CARTESIAN_POINT ( 'NONE',  ( 16.65937500061452070, 4.119189519843966529, -2.378215178124998275 ) ) ;
#42012=CARTESIAN_POINT ( 'NONE',  ( 29.38125000122903074, 6.123233995736764310E-16, -4.999999999999998224 ) ) ;
#42025=EDGE_LOOP ( 'NONE', ( #13742, #53655, #44991, #66280 ) ) ;
#42036=CARTESIAN_POINT ( 'NONE',  ( 20.32499999999999929, 6.123233995736764310E-16, -4.999999999999998224 ) ) ;
#42038=CARTESIAN_POINT ( 'NONE',  ( 7.509375000614517681, -4.119189519843965641, -2.378215178125001383 ) ) ;
#42044=FACE_OUTER_BOUND ( 'NONE', #42255, .T. ) ;
#42047=FACE_OUTER_BOUND ( 'NONE', #70463, .T. ) ;
#42057=CARTESIAN_POINT ( 'NONE',  ( 15.87187500061451573, -4.119189519843968306, 2.378215178124996054 ) ) ;
#42060=CARTESIAN_POINT ( 'NONE',  ( 23.22187500061451360, 5.824947211148865298E-16, -4.756430356249998326 ) ) ;
#42064=CARTESIAN_POINT ( 'NONE',  ( 45.00000000000000000, 6.123233995736764310E-16, -4.999999999999998224 ) ) ;
#42067=VECTOR ( 'NONE', #36166, 1000.000000000000000 ) ;
#42077=CARTESIAN_POINT ( 'NONE',  ( 25.88437500061451502, -4.119189519843968306, 2.378215178124996054 ) ) ;
#42080=DIRECTION ( 'NONE',  ( -1.000000000000000000, -0.000000000000000000, -0.000000000000000000 ) ) ;
#42088=CIRCLE ( 'NONE', #65387, 4.999999999999998224 ) ;
#42089=ORIENTED_EDGE ( 'NONE', *, *, #68503, .T. ) ;
#42098=CARTESIAN_POINT ( 'NONE',  ( 12.90937500061451537, -4.119189519843965641, -2.378215178125001383 ) ) ;
#42121=ORIENTED_EDGE ( 'NONE', *, *, #63109, .F. ) ;
#42124=CARTESIAN_POINT ( 'NONE',  ( 13.32187500061451502, -5.492252693125287522, -1.008910452111647106E-15 ) ) ;
#42131=CARTESIAN_POINT ( 'NONE',  ( 15.29999999999999893, -4.330127018922190985, -2.500000000000001332 ) ) ;
#42135=CARTESIAN_POINT ( 'NONE',  ( 24.27187500061451431, 4.119189519843966529, 2.378215178124999607 ) ) ;
#42139=CARTESIAN_POINT ( 'NONE',  ( 45.00000000000000000, 0.000000000000000000, 4.999999999999998224 ) ) ;
#42143=CARTESIAN_POINT ( 'NONE',  ( 21.38437500061451502, -2.746126346562642428, -4.756430356249999214 ) ) ;
#42145=CARTESIAN_POINT ( 'NONE',  ( 9.346875000614517148, 4.119189519843966529, -2.378215178124998275 ) ) ;
#42149=CARTESIAN_POINT ( 'NONE',  ( 9.843750001229032875, -2.886751345948130876, 4.999999999999996447 ) ) ;
#42156=CARTESIAN_POINT ( 'NONE',  ( 8.334375000614516082, -2.746126346562642428, -4.756430356249999214 ) ) ;
#42176=CARTESIAN_POINT ( 'NONE',  ( 23.02499999999999858, 6.123233995736764310E-16, -4.999999999999998224 ) ) ;
#42180=CARTESIAN_POINT ( 'NONE',  ( 19.35937500061451644, 4.119189519843966529, -2.378215178124998275 ) ) ;
#42213=CARTESIAN_POINT ( 'NONE',  ( 22.09687500061451715, 5.492252693125287522, 3.363034840372157021E-16 ) ) ;
#42219=CARTESIAN_POINT ( 'NONE',  ( 22.38749999999999929, -2.886751345948129988, 4.999999999999997335 ) ) ;
#42229=CARTESIAN_POINT ( 'NONE',  ( 28.58437500061451431, -2.746126346562642428, -4.756430356249999214 ) ) ;
#42231=CARTESIAN_POINT ( 'NONE',  ( 15.98437500061451821, -2.746126346562641984, -4.756430356249999214 ) ) ;
#42242=CARTESIAN_POINT ( 'NONE',  ( 16.59375000122903643, -2.886751345948074920, 5.000000000000092371 ) ) ;
#42243=CARTESIAN_POINT ( 'NONE',  ( 8.109375000614516438, 2.746126346562643317, 4.756430356249998326 ) ) ;
#42254=CARTESIAN_POINT ( 'NONE',  ( 28.69687500061451502, 4.119189519843966529, -2.378215178124998275 ) ) ;
#42255=EDGE_LOOP ( 'NONE', ( #61343, #38989, #65273, #19082 ) ) ;
#42258=CARTESIAN_POINT ( 'NONE',  ( 7.537500000000002309, -2.886751345948129988, 4.999999999999997335 ) ) ;
#42265=CARTESIAN_POINT ( 'NONE',  ( 25.54687500061451644, -2.746126346562641984, -4.756430356249999214 ) ) ;
#42267=CARTESIAN_POINT ( 'NONE',  ( 10.80937500061451928, 4.119189519843966529, -2.378215178124998275 ) ) ;
#42284=CARTESIAN_POINT ( 'NONE',  ( 21.05625000122903145, 0.000000000000000000, 4.999999999999998224 ) ) ;
#42299=CARTESIAN_POINT ( 'NONE',  ( 29.52187500061451431, -5.492252693125287522, -1.008910452111647106E-15 ) ) ;
#42319=CARTESIAN_POINT ( 'NONE',  ( 16.40625000122903643, 4.330127018922192761, -2.499999999999997780 ) ) ;
#42326=CARTESIAN_POINT ( 'NONE',  ( 27.97500000000000142, 6.123233995736764310E-16, -4.999999999999998224 ) ) ;
#42332=( BOUNDED_CURVE ( )  B_SPLINE_CURVE ( 3, ( #52301, #13481, #46042, #29412 ),
 .UNSPECIFIED., .F., .F. ) 
 B_SPLINE_CURVE_WITH_KNOTS ( ( 4, 4 ),
 ( 1.570796326794896780, 3.141592653589793116 ),
 .UNSPECIFIED. ) 
 CURVE ( )  GEOMETRIC_REPRESENTATION_ITEM ( )  RATIONAL_B_SPLINE_CURVE ( ( 1.000000000000000000, 0.8047378541243650485, 0.8047378541243650485, 1.000000000000000000 ) ) 
 REPRESENTATION_ITEM ( '' )  );
#42336=CARTESIAN_POINT ( 'NONE',  ( 11.62500000000000000, -4.330127018922194537, 2.499999999999995559 ) ) ;
#42339=CARTESIAN_POINT ( 'NONE',  ( 17.33437500061451431, -2.746126346562642428, -4.756430356249999214 ) ) ;
#42355=CARTESIAN_POINT ( 'NONE',  ( 26.00625000122903074, 0.000000000000000000, 4.999999999999998224 ) ) ;
#42356=LINE ( 'NONE', #25727, #24214 ) ;
#42357=CARTESIAN_POINT ( 'NONE',  ( 14.08125000122903181, 6.123233995736764310E-16, -4.999999999999998224 ) ) ;
#42360=CARTESIAN_POINT ( 'NONE',  ( 16.50937500061451502, -4.119189519843965641, -2.378215178125001383 ) ) ;
#42370=CARTESIAN_POINT ( 'NONE',  ( 45.00000000000000000, 6.123233995736764310E-16, -4.999999999999998224 ) ) ;
#42371=ORIENTED_EDGE ( 'NONE', *, *, #66440, .T. ) ;
#42374=DIRECTION ( 'NONE',  ( -1.000000000000000000, -0.000000000000000000, -0.000000000000000000 ) ) ;
#42378=CARTESIAN_POINT ( 'NONE',  ( 27.43125000122903145, -4.330127018922194537, 2.499999999999995559 ) ) ;
#42380=FACE_OUTER_BOUND ( 'NONE', #308, .T. ) ;
#42382=CARTESIAN_POINT ( 'NONE',  ( 45.00000000000000000, 0.000000000000000000, 0.000000000000000000 ) ) ;
#42390=VERTEX_POINT ( 'NONE', #1274 ) ;
#42400=( BOUNDED_CURVE ( )  B_SPLINE_CURVE ( 2, ( #60872, #5822, #10275, #32807, #55345, #4739, #27273 ),
 .UNSPECIFIED., .F., .F. ) 
 B_SPLINE_CURVE_WITH_KNOTS ( ( 3, 2, 2, 3 ),
 ( 0.1400000000000000133, 0.1433333333333333404, 0.1466666666666666674, 0.1499999999999999944 ),
 .UNSPECIFIED. ) 
 CURVE ( )  GEOMETRIC_REPRESENTATION_ITEM ( )  RATIONAL_B_SPLINE_CURVE ( ( 1.000000000000000000, 0.8660254037844387076, 1.000000000000000000, 0.8660254037844387076, 1.000000000000000000, 0.8660254037844387076, 1.000000000000000000 ) ) 
 REPRESENTATION_ITEM ( '' )  );
#42403=CARTESIAN_POINT ( 'NONE',  ( 28.87499999999999645, 6.123233995736764310E-16, -4.999999999999998224 ) ) ;
#42410=ADVANCED_FACE ( 'NONE', ( #46335 ), #69592, .T. ) ;
#42423=CARTESIAN_POINT ( 'NONE',  ( 14.63437500061451502, -2.746126346562642428, -4.756430356249999214 ) ) ;
#42426=CARTESIAN_POINT ( 'NONE',  ( 23.97187500061451715, -4.119189519843968306, 2.378215178124996054 ) ) ;
#42431=CARTESIAN_POINT ( 'NONE',  ( 15.45000000000000107, 4.330127018922192761, -2.499999999999997780 ) ) ;
#42435=CARTESIAN_POINT ( 'NONE',  ( 23.64375000122903359, 5.773502691896255534, 3.535250795749688401E-16 ) ) ;
#42436=CARTESIAN_POINT ( 'NONE',  ( 13.76250000000000107, 2.886751345948126879, 4.999999999999999112 ) ) ;
#42443=CARTESIAN_POINT ( 'NONE',  ( 25.43437500061451573, -4.119189519843968306, 2.378215178124996054 ) ) ;
#42447=CARTESIAN_POINT ( 'NONE',  ( 45.00000000000000000, 0.000000000000000000, 0.000000000000000000 ) ) ;
#42453=ORIENTED_EDGE ( 'NONE', *, *, #40242, .F. ) ;
#42463=CARTESIAN_POINT ( 'NONE',  ( 11.82187500061451857, 2.746126346562643317, 4.756430356249998326 ) ) ;
#42476=VERTEX_POINT ( 'NONE', #35961 ) ;
#42492=CARTESIAN_POINT ( 'NONE',  ( 14.97187500061451892, 2.746126346562643317, 4.756430356249998326 ) ) ;
#42499=CARTESIAN_POINT ( 'NONE',  ( 15.93750000000000000, 5.773502691896255534, 3.535250795749688894E-16 ) ) ;
#42501=DIRECTION ( 'NONE',  ( -1.000000000000000000, -0.000000000000000000, -0.000000000000000000 ) ) ;
#42509=CARTESIAN_POINT ( 'NONE',  ( 21.98437500061451644, 5.492252693125287522, 3.363034840372157021E-16 ) ) ;
#42511=CARTESIAN_POINT ( 'NONE',  ( 8.559375000614515727, 2.746126346562643317, 4.756430356249998326 ) ) ;
#42521=CARTESIAN_POINT ( 'NONE',  ( 9.459375000614519635, 2.746126346562643317, 4.756430356249998326 ) ) ;
#42540=CARTESIAN_POINT ( 'NONE',  ( 22.98750000000000071, -2.886751345948126435, -5.000000000000000000 ) ) ;
#42543=CARTESIAN_POINT ( 'NONE',  ( 19.92187500061451644, 2.746126346562643317, 4.756430356249998326 ) ) ;
#42575=CARTESIAN_POINT ( 'NONE',  ( 20.93437500061451573, -4.119189519843968306, 2.378215178124996054 ) ) ;
#42583=CARTESIAN_POINT ( 'NONE',  ( 23.28750000000000142, -2.886751345948129988, 4.999999999999997335 ) ) ;
#42586=CARTESIAN_POINT ( 'NONE',  ( 8.849999999999999645, 0.000000000000000000, 4.999999999999998224 ) ) ;
#42589=CARTESIAN_POINT ( 'NONE',  ( 19.51875000122903359, 2.886751345948129099, -4.999999999999997335 ) ) ;
#42594=CARTESIAN_POINT ( 'NONE',  ( 7.481250001229032165, 4.330127018922191873, 2.499999999999999556 ) ) ;
#42596=CARTESIAN_POINT ( 'NONE',  ( 16.62187500061451573, 4.119189519843966529, 2.378215178124999607 ) ) ;
#42606=CARTESIAN_POINT ( 'NONE',  ( 9.159375000614517148, -5.492252693125287522, -1.008910452111647106E-15 ) ) ;
#42611=( BOUNDED_CURVE ( )  B_SPLINE_CURVE ( 2, ( #61418, #10452, #108, #51065, #10811, #32981, #33346 ),
 .UNSPECIFIED., .F., .F. ) 
 B_SPLINE_CURVE_WITH_KNOTS ( ( 3, 2, 2, 3 ),
 ( 0.5000000000000001110, 0.5033333333333334103, 0.5066666666666667096, 0.5100000000000000089 ),
 .UNSPECIFIED. ) 
 CURVE ( )  GEOMETRIC_REPRESENTATION_ITEM ( )  RATIONAL_B_SPLINE_CURVE ( ( 0.9999999999999955591, 0.8660254037844431485, 1.000000000000000000, 0.8660254037844387076, 1.000000000000000000, 0.8660254037844387076, 1.000000000000000000 ) ) 
 REPRESENTATION_ITEM ( '' )  );
#42612=VERTEX_POINT ( 'NONE', #54425 ) ;
#42616=CARTESIAN_POINT ( 'NONE',  ( 19.85625000122902861, -4.330127018922190985, -2.500000000000001332 ) ) ;
#42618=CARTESIAN_POINT ( 'NONE',  ( 28.58437500061451431, -2.746126346562642428, -4.756430356249999214 ) ) ;
#42629=CARTESIAN_POINT ( 'NONE',  ( 26.70937500061451431, 0.000000000000000000, 4.756430356249998326 ) ) ;
#42631=CARTESIAN_POINT ( 'NONE',  ( 10.84687500061451892, 5.492252693125287522, 3.363034840372157021E-16 ) ) ;
#42649=CARTESIAN_POINT ( 'NONE',  ( 20.00625000122903430, 4.330127018922192761, -2.499999999999997780 ) ) ;
#42664=CARTESIAN_POINT ( 'NONE',  ( 28.54687500061451644, -2.746126346562646425, 4.756430356249996549 ) ) ;
#42665=EDGE_CURVE ( 'NONE', #1656, #42390, #104, .T. ) ;
#42683=CARTESIAN_POINT ( 'NONE',  ( 45.00000000000000000, 0.000000000000000000, 4.999999999999998224 ) ) ;
#42695=ORIENTED_EDGE ( 'NONE', *, *, #36009, .F. ) ;
#42698=ORIENTED_EDGE ( 'NONE', *, *, #30396, .T. ) ;
#42702=CARTESIAN_POINT ( 'NONE',  ( 17.55937500061451573, 2.746126346562643317, 4.756430356249998326 ) ) ;
#42707=CARTESIAN_POINT ( 'NONE',  ( 18.30000000000000071, 0.000000000000000000, 4.999999999999998224 ) ) ;
#42711=EDGE_LOOP ( 'NONE', ( #67927, #63759, #47260, #7248 ) ) ;
#42718=DIRECTION ( 'NONE',  ( -1.000000000000000000, -0.000000000000000000, -0.000000000000000000 ) ) ;
#42722=CARTESIAN_POINT ( 'NONE',  ( 18.38437500061451857, 5.824947211148865298E-16, -4.756430356249998326 ) ) ;
#42741=CARTESIAN_POINT ( 'NONE',  ( 28.44375000122902719, -2.886751345948125991, -5.000000000000000000 ) ) ;
#42766=CARTESIAN_POINT ( 'NONE',  ( 29.58749999999999858, -2.886751345948129988, 4.999999999999997335 ) ) ;
#42783=CARTESIAN_POINT ( 'NONE',  ( 15.34687500061451537, 0.000000000000000000, 4.756430356249998326 ) ) ;
#42787=CARTESIAN_POINT ( 'NONE',  ( 24.60937500061451644, 2.746126346562645981, -4.756430356249997438 ) ) ;
#42796=CARTESIAN_POINT ( 'NONE',  ( 8.456250001229033586, 0.000000000000000000, 4.999999999999998224 ) ) ;
#42797=CARTESIAN_POINT ( 'NONE',  ( 12.90000000000000213, 0.000000000000000000, 4.999999999999998224 ) ) ;
#42804=CARTESIAN_POINT ( 'NONE',  ( 25.69687500061451502, 5.492252693125287522, 3.363034840372157021E-16 ) ) ;
#42814=CARTESIAN_POINT ( 'NONE',  ( 7.106250001229032165, 0.000000000000000000, 4.999999999999998224 ) ) ;
#42824=CARTESIAN_POINT ( 'NONE',  ( 8.934375000614517504, 5.824947211148865298E-16, -4.756430356249998326 ) ) ;
#42828=EDGE_CURVE ( 'NONE', #53311, #23511, #14888, .T. ) ;
#42854=CARTESIAN_POINT ( 'NONE',  ( 14.29687500061451821, -2.746126346562642428, -4.756430356249999214 ) ) ;
#42862=CARTESIAN_POINT ( 'NONE',  ( 14.28750000000000142, -2.886751345948129988, 4.999999999999997335 ) ) ;
#42864=CARTESIAN_POINT ( 'NONE',  ( 34.99999999999999289, 0.000000000000000000, 4.999999999999998224 ) ) ;
#42868=EDGE_CURVE ( 'NONE', #31980, #26340, #37788, .T. ) ;
#42875=CARTESIAN_POINT ( 'NONE',  ( 22.35937500061451644, 2.746126346562645981, -4.756430356249997438 ) ) ;
#42877=CARTESIAN_POINT ( 'NONE',  ( 9.046875000614514661, 0.000000000000000000, 4.756430356249998326 ) ) ;
#42888=CARTESIAN_POINT ( 'NONE',  ( 9.871875000614517504, 4.119189519843966529, 2.378215178124999607 ) ) ;
#42911=CARTESIAN_POINT ( 'NONE',  ( 20.29687500061451289, 5.492252693125287522, 3.363034840372157021E-16 ) ) ;
#42942=CARTESIAN_POINT ( 'NONE',  ( 21.64687500061451786, 5.492252693125287522, 3.363034840372157021E-16 ) ) ;
#42948=CARTESIAN_POINT ( 'NONE',  ( 22.27499999999999858, 4.330127018922191873, 2.499999999999999556 ) ) ;
#42958=CARTESIAN_POINT ( 'NONE',  ( 7.406250001229033764, 4.330127018922192761, -2.499999999999997780 ) ) ;
#42960=CARTESIAN_POINT ( 'NONE',  ( 15.27187500061451608, 4.119189519843966529, 2.378215178124999607 ) ) ;
#42966=CARTESIAN_POINT ( 'NONE',  ( 25.98750000000000426, -2.886751345948157965, 4.999999999999948486 ) ) ;
#42970=CARTESIAN_POINT ( 'NONE',  ( 7.996875000614515727, 4.119189519843966529, -2.378215178124998275 ) ) ;
#42976=ORIENTED_EDGE ( 'NONE', *, *, #50505, .T. ) ;
#42982=CARTESIAN_POINT ( 'NONE',  ( 16.14375000122903359, -2.886751345948130876, 4.999999999999996447 ) ) ;
#42983=VERTEX_POINT ( 'NONE', #8620 ) ;
#42986=CARTESIAN_POINT ( 'NONE',  ( 8.775000000000002132, 4.330127018922191873, 2.499999999999999556 ) ) ;
#42994=CARTESIAN_POINT ( 'NONE',  ( 26.55937500061451573, 4.119189519843966529, -2.378215178124998275 ) ) ;
#42996=CARTESIAN_POINT ( 'NONE',  ( 8.521875000614516082, 2.746126346562645981, -4.756430356249997438 ) ) ;
#43015=CARTESIAN_POINT ( 'NONE',  ( 21.16875000122903216, -5.773502691896255534, -1.060575238724906372E-15 ) ) ;
#43023=CARTESIAN_POINT ( 'NONE',  ( 23.23125000122903216, 4.330127018922191873, 2.499999999999999556 ) ) ;
#43030=CARTESIAN_POINT ( 'NONE',  ( 29.10937500061451644, -4.119189519843965641, -2.378215178125001383 ) ) ;
#43054=ORIENTED_EDGE ( 'NONE', *, *, #7959, .T. ) ;
#43069=CARTESIAN_POINT ( 'NONE',  ( 14.07187500061451679, -4.119189519843968306, 2.378215178124996054 ) ) ;
#43071=( BOUNDED_CURVE ( )  B_SPLINE_CURVE ( 2, ( #14594, #65574, #25316, #53769, #59286, #19767, #47862 ),
 .UNSPECIFIED., .F., .F. ) 
 B_SPLINE_CURVE_WITH_KNOTS ( ( 3, 2, 2, 3 ),
 ( 0.2999999999999999889, 0.3033333333333333437, 0.3066666666666666430, 0.3099999999999999978 ),
 .UNSPECIFIED. ) 
 CURVE ( )  GEOMETRIC_REPRESENTATION_ITEM ( )  RATIONAL_B_SPLINE_CURVE ( ( 1.000000000000000000, 0.8660254037844387076, 1.000000000000000000, 0.8660254037844387076, 1.000000000000000000, 0.8660254037844387076, 1.000000000000000000 ) ) 
 REPRESENTATION_ITEM ( '' )  );
#43078=ORIENTED_EDGE ( 'NONE', *, *, #51591, .T. ) ;
#43084=DIRECTION ( 'NONE',  ( 0.000000000000000000, 0.000000000000000000, 1.000000000000000000 ) ) ;
#43087=CARTESIAN_POINT ( 'NONE',  ( 17.82187500061451502, -5.492252693125287522, -1.008910452111647106E-15 ) ) ;
#43096=EDGE_CURVE ( 'NONE', #32613, #39358, #62499, .T. ) ;
#43102=CARTESIAN_POINT ( 'NONE',  ( 24.46875000122903643, 2.886751345948129099, -4.999999999999997335 ) ) ;
#43106=CARTESIAN_POINT ( 'NONE',  ( 28.06875000122903074, 2.886751345948129099, -4.999999999999998224 ) ) ;
#43108=DIRECTION ( 'NONE',  ( 0.4999999999999975575, 0.000000000000000000, 0.8660254037844400399 ) ) ;
#43132=CARTESIAN_POINT ( 'NONE',  ( 26.55000000000000071, -4.330127018922190985, -2.500000000000001332 ) ) ;
#43142=ADVANCED_FACE ( 'NONE', ( #11897 ), #6354, .T. ) ;
#43151=APPLICATION_CONTEXT ( 'automotive_design' ) ;
#43153=EDGE_CURVE ( 'NONE', #41603, #8225, #68485, .T. ) ;
#43155=AXIS2_PLACEMENT_3D ( 'NONE', #10086, #15976, #32616 ) ;
#43156=CARTESIAN_POINT ( 'NONE',  ( 13.84687500061451715, 4.119189519843966529, -2.378215178124998275 ) ) ;
#43160=CARTESIAN_POINT ( 'NONE',  ( 24.12187500061451573, 5.824947211148865298E-16, -4.756430356249998326 ) ) ;
#43164=CARTESIAN_POINT ( 'NONE',  ( 23.96249999999999858, 2.886751345948101122, -5.000000000000046185 ) ) ;
#43171=CARTESIAN_POINT ( 'NONE',  ( 13.53749999999999964, -2.886751345948125991, -5.000000000000000000 ) ) ;
#43178=CARTESIAN_POINT ( 'NONE',  ( 24.30937500061451573, 4.119189519843966529, -2.378215178124998275 ) ) ;
#43181=DIRECTION ( 'NONE',  ( -1.000000000000000000, -0.000000000000000000, -0.000000000000000000 ) ) ;
#43195=CARTESIAN_POINT ( 'NONE',  ( 28.55625000122903145, 4.330127018922192761, -2.499999999999997780 ) ) ;
#43199=CARTESIAN_POINT ( 'NONE',  ( 9.384375000614518569, 5.824947211148865298E-16, -4.756430356249998326 ) ) ;
#43208=AXIS2_PLACEMENT_3D ( 'NONE', #33750, #40034, #34107 ) ;
#43224=ORIENTED_EDGE ( 'NONE', *, *, #27906, .T. ) ;
#43227=CARTESIAN_POINT ( 'NONE',  ( 14.40937500061451715, 4.119189519843966529, -2.378215178124998275 ) ) ;
#43235=CARTESIAN_POINT ( 'NONE',  ( 14.51250000000000107, 2.886751345948129099, -4.999999999999998224 ) ) ;
#43240=ADVANCED_FACE ( 'NONE', ( #22612 ), #461, .T. ) ;
#43245=EDGE_CURVE ( 'NONE', #61968, #28919, #62145, .T. ) ;
#43248=CARTESIAN_POINT ( 'NONE',  ( 19.02187500061451431, -4.119189519843968306, 2.378215178124996054 ) ) ;
#43262=CARTESIAN_POINT ( 'NONE',  ( 10.50937500061451502, -5.492252693125287522, -1.008910452111647106E-15 ) ) ;
#43269=CARTESIAN_POINT ( 'NONE',  ( 45.00000000000000000, 6.123233995736764310E-16, -4.999999999999998224 ) ) ;
#43273=VERTEX_POINT ( 'NONE', #11540 ) ;
#43282=CARTESIAN_POINT ( 'NONE',  ( 14.23125000122903394, 4.330127018922191873, 2.499999999999999556 ) ) ;
#43284=EDGE_CURVE ( 'NONE', #15624, #35381, #68932, .T. ) ;
#43286=CARTESIAN_POINT ( 'NONE',  ( 18.27187500061451431, -5.492252693125287522, -1.008910452111647106E-15 ) ) ;
#43306=VECTOR ( 'NONE', #51975, 1000.000000000000000 ) ;
#43318=CARTESIAN_POINT ( 'NONE',  ( 22.05937500061451573, 4.119189519843966529, -2.378215178124998275 ) ) ;
#43324=CARTESIAN_POINT ( 'NONE',  ( 22.61250000000000071, 2.886751345948129099, -4.999999999999998224 ) ) ;
#43330=CARTESIAN_POINT ( 'NONE',  ( 11.83125000122903181, 6.123233995736764310E-16, -4.999999999999998224 ) ) ;
#43335=CARTESIAN_POINT ( 'NONE',  ( 7.293750001229033053, -2.886751345948125991, -5.000000000000000000 ) ) ;
#43337=CARTESIAN_POINT ( 'NONE',  ( 14.74687500061451573, 4.119189519843966529, -2.378215178124998275 ) ) ;
#43348=DIRECTION ( 'NONE',  ( -1.000000000000000000, -0.000000000000000000, -0.000000000000000000 ) ) ;
#43349=CARTESIAN_POINT ( 'NONE',  ( 8.334375000614516082, -2.746126346562642428, -4.756430356249999214 ) ) ;
#43370=CARTESIAN_POINT ( 'NONE',  ( 23.44687500061451502, 5.492252693125287522, 3.363034840372157021E-16 ) ) ;
#43372=CARTESIAN_POINT ( 'NONE',  ( 7.509375000614517681, -4.119189519843965641, -2.378215178125001383 ) ) ;
#43389=CARTESIAN_POINT ( 'NONE',  ( 17.56875000122903074, -5.773502691896255534, -1.060575238724906372E-15 ) ) ;
#43391=CARTESIAN_POINT ( 'NONE',  ( 21.31875000122903430, 2.886751345948129099, -4.999999999999997335 ) ) ;
#43392=ORIENTED_EDGE ( 'NONE', *, *, #17585, .T. ) ;
#43404=CARTESIAN_POINT ( 'NONE',  ( 27.94687500061451502, 5.492252693125287522, 3.363034840372157021E-16 ) ) ;
#43413=EDGE_CURVE ( 'NONE', #44627, #4916, #61377, .T. ) ;
#43418=EDGE_CURVE ( 'NONE', #16810, #32393, #2888, .T. ) ;
#43428=ORIENTED_EDGE ( 'NONE', *, *, #55179, .T. ) ;
#43443=CARTESIAN_POINT ( 'NONE',  ( 13.17187500061451466, -4.119189519843968306, 2.378215178124996054 ) ) ;
#43460=CARTESIAN_POINT ( 'NONE',  ( 14.67187500061451821, -5.492252693125287522, -1.008910452111647106E-15 ) ) ;
#43477=CARTESIAN_POINT ( 'NONE',  ( 26.30625000122903145, 4.330127018922192761, -2.499999999999997780 ) ) ;
#43479=FACE_OUTER_BOUND ( 'NONE', #14761, .T. ) ;
#43480=( BOUNDED_CURVE ( )  B_SPLINE_CURVE ( 2, ( #39498, #44324, #67579, #66854, #72751, #33578, #11051 ),
 .UNSPECIFIED., .F., .F. ) 
 B_SPLINE_CURVE_WITH_KNOTS ( ( 3, 2, 2, 3 ),
 ( 0.5600000000000000533, 0.5633333333333333526, 0.5666666666666667629, 0.5700000000000000622 ),
 .UNSPECIFIED. ) 
 CURVE ( )  GEOMETRIC_REPRESENTATION_ITEM ( )  RATIONAL_B_SPLINE_CURVE ( ( 1.000000000000000000, 0.8660254037844387076, 1.000000000000000000, 0.8660254037844387076, 1.000000000000000000, 0.8660254037844342667, 1.000000000000004441 ) ) 
 REPRESENTATION_ITEM ( '' )  );
#43498=( BOUNDED_CURVE ( )  B_SPLINE_CURVE ( 2, ( #51825, #1228, #29650, #17819, #41467, #23734, #18548 ),
 .UNSPECIFIED., .F., .F. ) 
 B_SPLINE_CURVE_WITH_KNOTS ( ( 3, 2, 2, 3 ),
 ( 0.06000000000000003941, 0.06333333333333336645, 0.06666666666666667962, 0.07000000000000000666 ),
 .UNSPECIFIED. ) 
 CURVE ( )  GEOMETRIC_REPRESENTATION_ITEM ( )  RATIONAL_B_SPLINE_CURVE ( ( 0.9999999999999983347, 0.8660254037844403729, 1.000000000000000000, 0.8660254037844387076, 1.000000000000000000, 0.8660254037844387076, 1.000000000000000000 ) ) 
 REPRESENTATION_ITEM ( '' )  );
#43511=( BOUNDED_CURVE ( )  B_SPLINE_CURVE ( 2, ( #47550, #52366, #70079, #30197, #24284, #18727, #12835 ),
 .UNSPECIFIED., .F., .F. ) 
 B_SPLINE_CURVE_WITH_KNOTS ( ( 3, 2, 2, 3 ),
 ( 0.9500000000000000666, 0.9533333333333334769, 0.9566666666666666652, 0.9599999999999999645 ),
 .UNSPECIFIED. ) 
 CURVE ( )  GEOMETRIC_REPRESENTATION_ITEM ( )  RATIONAL_B_SPLINE_CURVE ( ( 0.9999999999999955591, 0.8660254037844431485, 1.000000000000000000, 0.8660254037844387076, 1.000000000000000000, 0.8660254037844387076, 1.000000000000000000 ) ) 
 REPRESENTATION_ITEM ( '' )  );
#43526=CARTESIAN_POINT ( 'NONE',  ( 20.25937500061451502, 2.746126346562643317, 4.756430356249998326 ) ) ;
#43536=CARTESIAN_POINT ( 'NONE',  ( 12.97499999999999964, -4.330127018922194537, 2.499999999999995559 ) ) ;
#43543=CARTESIAN_POINT ( 'NONE',  ( 23.52187500061451786, 2.746126346562643317, 4.756430356249998326 ) ) ;
#43564=CARTESIAN_POINT ( 'NONE',  ( 9.346875000614517148, -2.746126346562641984, -4.756430356249999214 ) ) ;
#43566=EDGE_CURVE ( 'NONE', #46196, #6912, #22749, .T. ) ;
#43590=CARTESIAN_POINT ( 'NONE',  ( 10.69687500061451679, -2.746126346562642428, -4.756430356249999214 ) ) ;
#43606=CARTESIAN_POINT ( 'NONE',  ( 20.00625000122903430, 4.330127018922192761, -2.499999999999997780 ) ) ;
#43610=CARTESIAN_POINT ( 'NONE',  ( 19.43437500061451573, -2.746126346562646425, 4.756430356249996549 ) ) ;
#43613=CARTESIAN_POINT ( 'NONE',  ( 13.93125000122903323, -4.330127018922194537, 2.499999999999995559 ) ) ;
#43627=CARTESIAN_POINT ( 'NONE',  ( 10.28437500061451892, 5.492252693125287522, 3.363034840372157021E-16 ) ) ;
#43648=CARTESIAN_POINT ( 'NONE',  ( 18.30937500061451928, -4.119189519843965641, -2.378215178125001383 ) ) ;
#43656=EDGE_CURVE ( 'NONE', #56819, #35566, #35511, .T. ) ;
#43681=CARTESIAN_POINT ( 'NONE',  ( 19.69687500061451857, -2.746126346562642428, -4.756430356249999214 ) ) ;
#43687=CARTESIAN_POINT ( 'NONE',  ( 21.86250000000000071, 2.886751345948126879, 4.999999999999999112 ) ) ;
#43690=CARTESIAN_POINT ( 'NONE',  ( 24.13125000122903074, 4.330127018922191873, 2.499999999999999556 ) ) ;
#43699=CARTESIAN_POINT ( 'NONE',  ( 26.63437500061451146, -2.746126346562646425, 4.756430356249996549 ) ) ;
#43701=CARTESIAN_POINT ( 'NONE',  ( 13.95937500061451431, 2.746126346562643317, 4.756430356249998326 ) ) ;
#43711=CARTESIAN_POINT ( 'NONE',  ( 7.771875000614516082, -4.119189519843968306, 2.378215178124996054 ) ) ;
#43712=ORIENTED_EDGE ( 'NONE', *, *, #55693, .T. ) ;
#43732=CARTESIAN_POINT ( 'NONE',  ( 24.45937500061451786, 0.000000000000000000, 4.756430356249998326 ) ) ;
#43734=CARTESIAN_POINT ( 'NONE',  ( 8.746875000614515727, -2.746126346562646425, 4.756430356249996549 ) ) ;
#43752=CARTESIAN_POINT ( 'NONE',  ( 17.75625000122903074, 4.330127018922192761, -2.499999999999997780 ) ) ;
#43769=CARTESIAN_POINT ( 'NONE',  ( 29.33437500061451431, 4.119189519843966529, 2.378215178124999607 ) ) ;
#43777=CARTESIAN_POINT ( 'NONE',  ( 7.443750001229033408, 5.773502691896255534, 3.535250795749688401E-16 ) ) ;
#43783=CARTESIAN_POINT ( 'NONE',  ( 11.90625000122903465, 4.330127018922192761, -2.499999999999997780 ) ) ;
#43787=CARTESIAN_POINT ( 'NONE',  ( 20.14687500061451786, 4.119189519843966529, -2.378215178124998275 ) ) ;
#43797=ADVANCED_FACE ( 'NONE', ( #71063 ), #20438, .T. ) ;
#43806=CARTESIAN_POINT ( 'NONE',  ( 12.26249999999999751, 2.886751345948073588, -5.000000000000094147 ) ) ;
#43807=CARTESIAN_POINT ( 'NONE',  ( 14.55937500061451750, -5.492252693125287522, -1.008910452111647106E-15 ) ) ;
#43814=ORIENTED_EDGE ( 'NONE', *, *, #25568, .F. ) ;
#43826=CARTESIAN_POINT ( 'NONE',  ( 14.97187500061451892, 2.746126346562643317, 4.756430356249998326 ) ) ;
#43839=CARTESIAN_POINT ( 'NONE',  ( 24.54375000122903216, 5.773502691896255534, 3.535250795749688401E-16 ) ) ;
#43843=CARTESIAN_POINT ( 'NONE',  ( 24.69375000122903074, -2.886751345948129988, 4.999999999999997335 ) ) ;
#43857=CARTESIAN_POINT ( 'NONE',  ( 10.44375000122903252, -2.886751345948237457, -4.999999999999807265 ) ) ;
#43894=CARTESIAN_POINT ( 'NONE',  ( 21.00937500061451857, 2.746126346562645981, -4.756430356249997438 ) ) ;
#43903=CARTESIAN_POINT ( 'NONE',  ( 12.11250000000000249, -5.773502691896255534, -1.060575238724906372E-15 ) ) ;
#43910=CARTESIAN_POINT ( 'NONE',  ( 22.80937500061451573, -4.119189519843965641, -2.378215178125001383 ) ) ;
#43931=CARTESIAN_POINT ( 'NONE',  ( 10.39687500061451786, 5.492252693125287522, 3.363034840372157021E-16 ) ) ;
#43942=ORIENTED_EDGE ( 'NONE', *, *, #31318, .F. ) ;
#43945=DIRECTION ( 'NONE',  ( 0.000000000000000000, 0.000000000000000000, 1.000000000000000000 ) ) ;
#43958=CARTESIAN_POINT ( 'NONE',  ( 12.53437500061451537, 5.824947211148865298E-16, -4.756430356249998326 ) ) ;
#43977=CARTESIAN_POINT ( 'NONE',  ( 19.77187500061451786, 4.119189519843966529, 2.378215178124999607 ) ) ;
#43980=CARTESIAN_POINT ( 'NONE',  ( 14.68125000122903323, 4.330127018922191873, 2.499999999999999556 ) ) ;
#43994=CARTESIAN_POINT ( 'NONE',  ( 29.67187500061451644, 2.746126346562645981, -4.756430356249997438 ) ) ;
#43999=CARTESIAN_POINT ( 'NONE',  ( 19.20000000000000284, 0.000000000000000000, 4.999999999999998224 ) ) ;
#44001=DIRECTION ( 'NONE',  ( 0.000000000000000000, 0.000000000000000000, 1.000000000000000000 ) ) ;
#44003=EDGE_LOOP ( 'NONE', ( #40163, #71832, #46173, #62322 ) ) ;
#44015=CARTESIAN_POINT ( 'NONE',  ( 16.62187500061451573, 2.746126346562645981, -4.756430356249997438 ) ) ;
#44019=ORIENTED_EDGE ( 'NONE', *, *, #71436, .T. ) ;
#44048=CARTESIAN_POINT ( 'NONE',  ( 19.62187500061451573, -5.492252693125287522, -1.008910452111647106E-15 ) ) ;
#44054=CARTESIAN_POINT ( 'NONE',  ( 20.73750000000000071, -2.886751345948125991, -5.000000000000000000 ) ) ;
#44056=CARTESIAN_POINT ( 'NONE',  ( 20.58749999999999858, -2.886751345948074920, 5.000000000000092371 ) ) ;
#44062=EDGE_CURVE ( 'NONE', #27832, #48021, #62876, .T. ) ;
#44064=CARTESIAN_POINT ( 'NONE',  ( 26.82187500061451502, 5.824947211148865298E-16, -4.756430356249998326 ) ) ;
#44066=CARTESIAN_POINT ( 'NONE',  ( 12.72187500061451537, -4.119189519843968306, 2.378215178124996054 ) ) ;
#44076=CARTESIAN_POINT ( 'NONE',  ( 20.60625000122902861, 0.000000000000000000, 4.999999999999998224 ) ) ;
#44102=CARTESIAN_POINT ( 'NONE',  ( 23.59687500061451715, -2.746126346562646425, 4.756430356249996549 ) ) ;
#44104=CARTESIAN_POINT ( 'NONE',  ( 8.446875000614518569, -2.746126346562642428, -4.756430356249999214 ) ) ;
#44111=CARTESIAN_POINT ( 'NONE',  ( 20.02500000000000213, 4.330127018922191873, 2.499999999999999556 ) ) ;
#44122=CARTESIAN_POINT ( 'NONE',  ( 18.09375000122903288, -2.886751345948125991, -5.000000000000000000 ) ) ;
#44124=FACE_OUTER_BOUND ( 'NONE', #19101, .T. ) ;
#44138=CARTESIAN_POINT ( 'NONE',  ( 26.44687500061451502, -2.746126346562642428, -4.756430356249999214 ) ) ;
#44143=( BOUNDED_CURVE ( )  B_SPLINE_CURVE ( 2, ( #15072, #37609, #8806, #37247, #42431, #64952, #14344 ),
 .UNSPECIFIED., .F., .F. ) 
 B_SPLINE_CURVE_WITH_KNOTS ( ( 3, 2, 2, 3 ),
 ( 0.6400000000000001243, 0.6433333333333334236, 0.6466666666666666119, 0.6500000000000000222 ),
 .UNSPECIFIED. ) 
 CURVE ( )  GEOMETRIC_REPRESENTATION_ITEM ( )  RATIONAL_B_SPLINE_CURVE ( ( 0.9999999999999955591, 0.8660254037844431485, 1.000000000000000000, 0.8660254037844387076, 1.000000000000000000, 0.8660254037844387076, 1.000000000000000000 ) ) 
 REPRESENTATION_ITEM ( '' )  );
#44147=CARTESIAN_POINT ( 'NONE',  ( 9.899999999999998579, -4.330127018922190985, -2.500000000000001332 ) ) ;
#44153=CARTESIAN_POINT ( 'NONE',  ( 10.70625000122903536, 0.000000000000000000, 4.999999999999998224 ) ) ;
#44157=CARTESIAN_POINT ( 'NONE',  ( 20.33437500061451786, -2.746126346562646425, 4.756430356249996549 ) ) ;
#44161=ORIENTED_EDGE ( 'NONE', *, *, #46859, .T. ) ;
#44162=CARTESIAN_POINT ( 'NONE',  ( 10.51875000122903181, 2.886751345948018077, -5.000000000000190070 ) ) ;
#44169=VERTEX_POINT ( 'NONE', #16985 ) ;
#44178=CARTESIAN_POINT ( 'NONE',  ( 12.98437500061451289, 5.492252693125287522, 3.363034840372157021E-16 ) ) ;
#44194=CARTESIAN_POINT ( 'NONE',  ( 28.95937500061451431, -5.492252693125287522, -1.008910452111647106E-15 ) ) ;
#44195=CARTESIAN_POINT ( 'NONE',  ( 14.33437500061451786, 5.824947211148865298E-16, -4.756430356249998326 ) ) ;
#44213=CARTESIAN_POINT ( 'NONE',  ( 25.03125000122903288, 4.330127018922191873, 2.499999999999999556 ) ) ;
#44253=CARTESIAN_POINT ( 'NONE',  ( 29.00625000122903074, 4.330127018922192761, -2.499999999999997780 ) ) ;
#44261=CARTESIAN_POINT ( 'NONE',  ( 22.05937500061451217, 2.746126346562643317, 4.756430356249998326 ) ) ;
#44271=CARTESIAN_POINT ( 'NONE',  ( 11.25000000000000000, -4.330127018922190985, -2.500000000000001332 ) ) ;
#44279=CARTESIAN_POINT ( 'NONE',  ( 22.62187500061451573, 2.746126346562643317, 4.756430356249998326 ) ) ;
#44291=VERTEX_POINT ( 'NONE', #39543 ) ;
#44303=CARTESIAN_POINT ( 'NONE',  ( 9.534375000614517148, 4.119189519843966529, 2.378215178124999607 ) ) ;
#44324=CARTESIAN_POINT ( 'NONE',  ( 17.36250000000000071, 2.886751345948126879, 4.999999999999998224 ) ) ;
#44326=CARTESIAN_POINT ( 'NONE',  ( 10.50937500061451679, 0.000000000000000000, 4.756430356249998326 ) ) ;
#44330=VECTOR ( 'NONE', #16628, 1000.000000000000000 ) ;
#44347=CYLINDRICAL_SURFACE ( 'NONE', #15480, 4.999999999999998224 ) ;
#44348=( BOUNDED_CURVE ( )  B_SPLINE_CURVE ( 3, ( #11321, #5776, #56021, #16477 ),
 .UNSPECIFIED., .F., .F. ) 
 B_SPLINE_CURVE_WITH_KNOTS ( ( 4, 4 ),
 ( 1.570796326794896780, 3.141592653589793116 ),
 .UNSPECIFIED. ) 
 CURVE ( )  GEOMETRIC_REPRESENTATION_ITEM ( )  RATIONAL_B_SPLINE_CURVE ( ( 1.000000000000000000, 0.8047378541243650485, 0.8047378541243650485, 1.000000000000000000 ) ) 
 REPRESENTATION_ITEM ( '' )  );
#44351=CARTESIAN_POINT ( 'NONE',  ( 20.74687500061451217, 0.000000000000000000, 4.756430356249998326 ) ) ;
#44354=CARTESIAN_POINT ( 'NONE',  ( 14.11875000122903323, 2.886751345948129099, -4.999999999999998224 ) ) ;
#44356=CARTESIAN_POINT ( 'NONE',  ( 7.584375000614516082, 5.492252693125287522, 3.363034840372157021E-16 ) ) ;
#44361=DIRECTION ( 'NONE',  ( -1.000000000000000000, -0.000000000000000000, -0.000000000000000000 ) ) ;
#44368=CARTESIAN_POINT ( 'NONE',  ( 29.82187500061451502, 2.746126346562643317, 4.756430356249998326 ) ) ;
#44374=DIRECTION ( 'NONE',  ( -1.000000000000000000, -0.000000000000000000, -0.000000000000000000 ) ) ;
#44391=CARTESIAN_POINT ( 'NONE',  ( 17.22187500061451715, 2.746126346562643317, 4.756430356249998326 ) ) ;
#44395=ORIENTED_EDGE ( 'NONE', *, *, #18491, .F. ) ;
#44422=CARTESIAN_POINT ( 'NONE',  ( 18.00937500061451502, 4.119189519843966529, -2.378215178124998275 ) ) ;
#44428=CARTESIAN_POINT ( 'NONE',  ( 20.10000000000000142, 0.000000000000000000, 4.999999999999998224 ) ) ;
#44432=CARTESIAN_POINT ( 'NONE',  ( 25.28437500061451360, -2.746126346562646425, 4.756430356249996549 ) ) ;
#44433=CARTESIAN_POINT ( 'NONE',  ( 16.78125000122903288, 6.123233995736764310E-16, -4.999999999999998224 ) ) ;
#44438=CARTESIAN_POINT ( 'NONE',  ( 26.67187500061451289, -4.119189519843968306, 2.378215178124996054 ) ) ;
#44440=CARTESIAN_POINT ( 'NONE',  ( 13.99687500061451395, 0.000000000000000000, 4.756430356249998326 ) ) ;
#44466=CARTESIAN_POINT ( 'NONE',  ( 25.63125000122903074, -4.330127018922194537, 2.499999999999995559 ) ) ;
#44474=CARTESIAN_POINT ( 'NONE',  ( 24.75937500061451502, 4.119189519843966529, -2.378215178124998275 ) ) ;
#44476=CARTESIAN_POINT ( 'NONE',  ( 8.334375000614516082, -4.119189519843968306, 2.378215178124996054 ) ) ;
#44481=ORIENTED_EDGE ( 'NONE', *, *, #17040, .T. ) ;
#44493=CARTESIAN_POINT ( 'NONE',  ( 18.69375000122903430, 5.773502691896255534, 3.535250795749688894E-16 ) ) ;
#44496=ORIENTED_EDGE ( 'NONE', *, *, #24962, .F. ) ;
#44509=CARTESIAN_POINT ( 'NONE',  ( 25.95937500061451431, -4.119189519843965641, -2.378215178125001383 ) ) ;
#44515=CARTESIAN_POINT ( 'NONE',  ( 28.19999999999999929, 0.000000000000000000, 4.999999999999998224 ) ) ;
#44523=CARTESIAN_POINT ( 'NONE',  ( 8.812500000000000000, 2.886751345948238789, 4.999999999999807265 ) ) ;
#44525=CARTESIAN_POINT ( 'NONE',  ( 12.65625000122903110, -4.330127018922190985, -2.500000000000001332 ) ) ;
#44529=CARTESIAN_POINT ( 'NONE',  ( 21.12187500061451217, 4.119189519843966529, 2.378215178124999607 ) ) ;
#44541=CARTESIAN_POINT ( 'NONE',  ( 11.85937500061451821, -5.492252693125287522, -1.008910452111647106E-15 ) ) ;
#44542=ORIENTED_EDGE ( 'NONE', *, *, #5151, .F. ) ;
#44547=CARTESIAN_POINT ( 'NONE',  ( 21.13125000122903074, -4.330127018922194537, 2.499999999999995559 ) ) ;
#44562=CARTESIAN_POINT ( 'NONE',  ( 13.53750000000000142, -2.886751345948126435, -5.000000000000000000 ) ) ;
#44565=CARTESIAN_POINT ( 'NONE',  ( 28.84687500061451360, 0.000000000000000000, 4.756430356249998326 ) ) ;
#44566=CARTESIAN_POINT ( 'NONE',  ( 14.52187500061451608, 2.746126346562643317, 4.756430356249998326 ) ) ;
#44567=CYLINDRICAL_SURFACE ( 'NONE', #30056, 4.999999999999998224 ) ;
#44583=CARTESIAN_POINT ( 'NONE',  ( 26.45625000122903003, 0.000000000000000000, 4.999999999999998224 ) ) ;
#44585=DIRECTION ( 'NONE',  ( -1.000000000000000000, -0.000000000000000000, -0.000000000000000000 ) ) ;
#44592=ADVANCED_FACE ( 'NONE', ( #57602 ), #69786, .T. ) ;
#44597=CARTESIAN_POINT ( 'NONE',  ( 13.66875000122902861, 2.886751345948018077, -5.000000000000190070 ) ) ;
#44600=EDGE_CURVE ( 'NONE', #35381, #1565, #53521, .T. ) ;
#44624=EDGE_CURVE ( 'NONE', #26527, #55366, #13255, .T. ) ;
#44627=VERTEX_POINT ( 'NONE', #63513 ) ;
#44630=ORIENTED_EDGE ( 'NONE', *, *, #18715, .F. ) ;
#44633=CARTESIAN_POINT ( 'NONE',  ( 22.13437500061451502, -2.746126346562646425, 4.756430356249996549 ) ) ;
#44642=CARTESIAN_POINT ( 'NONE',  ( 11.28749999999999787, -2.886751345948125991, -5.000000000000000000 ) ) ;
#44648=CARTESIAN_POINT ( 'NONE',  ( 22.23750000000000071, 5.773502691896255534, 3.535250795749688401E-16 ) ) ;
#44649=CARTESIAN_POINT ( 'NONE',  ( 23.22187500061451715, -5.492252693125287522, -1.008910452111647106E-15 ) ) ;
#44652=CARTESIAN_POINT ( 'NONE',  ( 20.10000000000000142, 0.000000000000000000, 4.999999999999998224 ) ) ;
#44671=CARTESIAN_POINT ( 'NONE',  ( 7.434375000614519280, -4.119189519843968306, 2.378215178124996054 ) ) ;
#44692=CARTESIAN_POINT ( 'NONE',  ( 12.49687500061451573, -2.746126346562642428, -4.756430356249999214 ) ) ;
#44701=DIRECTION ( 'NONE',  ( 0.000000000000000000, 0.000000000000000000, 1.000000000000000000 ) ) ;
#44709=CARTESIAN_POINT ( 'NONE',  ( 19.54687500061451289, -4.119189519843965641, -2.378215178125001383 ) ) ;
#44712=CARTESIAN_POINT ( 'NONE',  ( 14.56875000122903252, 2.886751345948129099, -4.999999999999998224 ) ) ;
#44716=CARTESIAN_POINT ( 'NONE',  ( 27.03750000000000142, -2.886751345948139758, -4.999999999999975131 ) ) ;
#44721=CARTESIAN_POINT ( 'NONE',  ( 19.48125000122903216, 6.123233995736764310E-16, -4.999999999999998224 ) ) ;
#44728=CARTESIAN_POINT ( 'NONE',  ( 29.63437500061451502, 5.824947211148865298E-16, -4.756430356249998326 ) ) ;
#44737=CARTESIAN_POINT ( 'NONE',  ( 15.11249999999999893, 2.886751345948126879, 4.999999999999998224 ) ) ;
#44751=CARTESIAN_POINT ( 'NONE',  ( 17.55937500061451573, 4.119189519843966529, -2.378215178124998275 ) ) ;
#44765=VERTEX_POINT ( 'NONE', #52071 ) ;
#44780=EDGE_CURVE ( 'NONE', #24228, #49807, #35793, .T. ) ;
#44784=CARTESIAN_POINT ( 'NONE',  ( 18.64687500061451786, -2.746126346562646425, 4.756430356249996549 ) ) ;
#44785=CARTESIAN_POINT ( 'NONE',  ( 14.64375000122903359, 5.773502691896255534, 3.535250795749688401E-16 ) ) ;
#44790=CARTESIAN_POINT ( 'NONE',  ( 19.16250000000000142, 2.886751345948126879, 4.999999999999999112 ) ) ;
#44793=CARTESIAN_POINT ( 'NONE',  ( 24.64687500061451431, 4.119189519843966529, -2.378215178124998275 ) ) ;
#44800=CARTESIAN_POINT ( 'NONE',  ( 27.30937500061451217, 2.746126346562645981, -4.756430356249997438 ) ) ;
#44802=CARTESIAN_POINT ( 'NONE',  ( 14.40937500061451537, 2.746126346562643317, 4.756430356249998326 ) ) ;
#44811=CARTESIAN_POINT ( 'NONE',  ( 20.75625000122903430, -4.330127018922190985, -2.500000000000001332 ) ) ;
#44833=CARTESIAN_POINT ( 'NONE',  ( 23.40937500061451715, 4.119189519843966529, -2.378215178124998275 ) ) ;
#44851=CARTESIAN_POINT ( 'NONE',  ( 18.43125000122903501, -4.330127018922194537, 2.499999999999995559 ) ) ;
#44854=ORIENTED_EDGE ( 'NONE', *, *, #66541, .F. ) ;
#44868=CARTESIAN_POINT ( 'NONE',  ( 24.83437500061451431, 4.119189519843966529, 2.378215178124999607 ) ) ;
#44874=CARTESIAN_POINT ( 'NONE',  ( 27.00000000000000000, -4.330127018922190985, -2.500000000000001332 ) ) ;
#44882=CARTESIAN_POINT ( 'NONE',  ( 12.95625000122903359, 0.000000000000000000, 4.999999999999998224 ) ) ;
#44886=CARTESIAN_POINT ( 'NONE',  ( 21.38437500061451502, -2.746126346562641984, -4.756430356249999214 ) ) ;
#44889=ORIENTED_EDGE ( 'NONE', *, *, #2122, .F. ) ;
#44892=DIRECTION ( 'NONE',  ( 0.000000000000000000, 0.000000000000000000, 1.000000000000000000 ) ) ;
#44893=CARTESIAN_POINT ( 'NONE',  ( 20.51249999999999574, 2.886751345948182834, 4.999999999999902300 ) ) ;
#44897=CARTESIAN_POINT ( 'NONE',  ( 12.68437500061451750, -2.746126346562646425, 4.756430356249996549 ) ) ;
#44906=CARTESIAN_POINT ( 'NONE',  ( 10.98750000000000071, 5.773502691896255534, 3.535250795749688401E-16 ) ) ;
#44911=ORIENTED_EDGE ( 'NONE', *, *, #55095, .F. ) ;
#44917=CARTESIAN_POINT ( 'NONE',  ( 29.32499999999999929, 6.123233995736764310E-16, -4.999999999999998224 ) ) ;
#44918=CARTESIAN_POINT ( 'NONE',  ( 13.42499999999999893, -4.330127018922194537, 2.499999999999995559 ) ) ;
#44921=CARTESIAN_POINT ( 'NONE',  ( 14.14687500061451786, -2.746126346562646425, 4.756430356249996549 ) ) ;
#44929=LINE ( 'NONE', #35994, #71385 ) ;
#44936=CARTESIAN_POINT ( 'NONE',  ( 45.00000000000000000, 6.123233995736764310E-16, -4.999999999999998224 ) ) ;
#44937=CARTESIAN_POINT ( 'NONE',  ( 26.49375000122903145, -2.886751345948129988, 4.999999999999997335 ) ) ;
#44942=DIRECTION ( 'NONE',  ( 0.000000000000000000, 1.000000000000000000, -0.000000000000000000 ) ) ;
#44946=EDGE_CURVE ( 'NONE', #61283, #40700, #20358, .T. ) ;
#44982=CARTESIAN_POINT ( 'NONE',  ( 21.87187500061451573, 5.824947211148865298E-16, -4.756430356249998326 ) ) ;
#44991=ORIENTED_EDGE ( 'NONE', *, *, #2783, .F. ) ;
#44993=CARTESIAN_POINT ( 'NONE',  ( 10.31250000000000355, -5.773502691896255534, -1.060575238724906372E-15 ) ) ;
#44998=DIRECTION ( 'NONE',  ( 0.000000000000000000, 0.000000000000000000, 1.000000000000000000 ) ) ;
#44999=CARTESIAN_POINT ( 'NONE',  ( 22.73437500061451644, -4.119189519843968306, 2.378215178124996054 ) ) ;
#45018=CARTESIAN_POINT ( 'NONE',  ( 18.37500000000000355, -4.330127018922194537, 2.499999999999995559 ) ) ;
#45023=CARTESIAN_POINT ( 'NONE',  ( 7.396875000614519635, -2.746126346562646425, 4.756430356249996549 ) ) ;
#45045=CARTESIAN_POINT ( 'NONE',  ( 11.07187500061451679, -5.492252693125287522, -1.008910452111647106E-15 ) ) ;
#45055=DIRECTION ( 'NONE',  ( -1.000000000000000000, -0.000000000000000000, -0.000000000000000000 ) ) ;
#45063=CARTESIAN_POINT ( 'NONE',  ( 18.64687500061451431, -4.119189519843965641, -2.378215178125001383 ) ) ;
#45066=CARTESIAN_POINT ( 'NONE',  ( 15.20625000122903181, 0.000000000000000000, 4.999999999999998224 ) ) ;
#45080=CARTESIAN_POINT ( 'NONE',  ( 7.884375000614518569, -2.746126346562642428, -4.756430356249999214 ) ) ;
#45099=DIRECTION ( 'NONE',  ( 1.000000000000000000, -0.000000000000000000, -0.000000000000000000 ) ) ;
#45102=CARTESIAN_POINT ( 'NONE',  ( 15.83437500061451608, 4.119189519843966529, 2.378215178124999607 ) ) ;
#45106=VERTEX_POINT ( 'NONE', #9190 ) ;
#45117=VERTEX_POINT ( 'NONE', #4396 ) ;
#45125=EDGE_CURVE ( 'NONE', #52599, #6077, #30299, .T. ) ;
#45129=CARTESIAN_POINT ( 'NONE',  ( 14.47499999999999964, 6.123233995736764310E-16, -4.999999999999998224 ) ) ;
#45131=ORIENTED_EDGE ( 'NONE', *, *, #46580, .F. ) ;
#45134=CARTESIAN_POINT ( 'NONE',  ( 18.57187500061451857, 2.746126346562643317, 4.756430356249998326 ) ) ;
#45136=DIRECTION ( 'NONE',  ( 0.000000000000000000, 8.673617379884035472E-17, 1.000000000000000000 ) ) ;
#45141=CARTESIAN_POINT ( 'NONE',  ( 18.86249999999999716, -5.773502691896255534, -1.060575238724906372E-15 ) ) ;
#45145=CARTESIAN_POINT ( 'NONE',  ( 26.29687500061451644, -4.119189519843965641, -2.378215178125001383 ) ) ;
#45153=CARTESIAN_POINT ( 'NONE',  ( 27.60937500061451644, -5.492252693125287522, -1.008910452111647106E-15 ) ) ;
#45155=CARTESIAN_POINT ( 'NONE',  ( 11.03437500061451182, -2.746126346562641984, -4.756430356249999214 ) ) ;
#45166=ORIENTED_EDGE ( 'NONE', *, *, #15334, .F. ) ;
#45179=ORIENTED_EDGE ( 'NONE', *, *, #27906, .F. ) ;
#45188=CARTESIAN_POINT ( 'NONE',  ( 21.00937500061451857, -4.119189519843965641, -2.378215178125001383 ) ) ;
#45196=CARTESIAN_POINT ( 'NONE',  ( 27.15000000000000213, 4.330127018922192761, -2.499999999999997780 ) ) ;
#45207=CARTESIAN_POINT ( 'NONE',  ( 15.69375000122903074, -2.886751345948129988, 4.999999999999997335 ) ) ;
#45223=CARTESIAN_POINT ( 'NONE',  ( 26.74687500061451573, -2.746126346562646425, 4.756430356249996549 ) ) ;
#45228=CARTESIAN_POINT ( 'NONE',  ( 28.01249999999999574, 2.886751345948129099, -4.999999999999998224 ) ) ;
#45230=CARTESIAN_POINT ( 'NONE',  ( 9.787499999999999645, -2.886751345948130876, 4.999999999999996447 ) ) ;
#45231=EDGE_CURVE ( 'NONE', #6912, #7983, #21358, .T. ) ;
#45237=CARTESIAN_POINT ( 'NONE',  ( 10.81875000122903252, -5.773502691896255534, -1.060575238724906372E-15 ) ) ;
#45241=CARTESIAN_POINT ( 'NONE',  ( 20.37187500061451217, -4.119189519843968306, 2.378215178124996054 ) ) ;
#45244=ORIENTED_EDGE ( 'NONE', *, *, #14641, .F. ) ;
#45247=DIRECTION ( 'NONE',  ( -1.000000000000000000, -0.000000000000000000, -0.000000000000000000 ) ) ;
#45253=CARTESIAN_POINT ( 'NONE',  ( 12.94687500061451502, 4.119189519843966529, -2.378215178124998275 ) ) ;
#45254=ORIENTED_EDGE ( 'NONE', *, *, #893, .T. ) ;
#45277=CARTESIAN_POINT ( 'NONE',  ( 29.14687500061451431, 4.119189519843966529, -2.378215178124998275 ) ) ;
#45278=CARTESIAN_POINT ( 'NONE',  ( 11.82187500061451679, 2.746126346562643317, 4.756430356249998326 ) ) ;
#45286=CARTESIAN_POINT ( 'NONE',  ( 14.47499999999999964, 6.123233995736764310E-16, -4.999999999999998224 ) ) ;
#45294=DIRECTION ( 'NONE',  ( -1.000000000000000000, -0.000000000000000000, -0.000000000000000000 ) ) ;
#45295=CARTESIAN_POINT ( 'NONE',  ( 22.59375000122903288, -2.886751345948125991, -5.000000000000000000 ) ) ;
#45303=CARTESIAN_POINT ( 'NONE',  ( 25.33125000122903003, 6.123233995736764310E-16, -4.999999999999998224 ) ) ;
#45320=CARTESIAN_POINT ( 'NONE',  ( 12.05625000122903145, 0.000000000000000000, 4.999999999999998224 ) ) ;
#45331=MANIFOLD_SOLID_BREP ( 'Cut-Extrude1', #38304 ) ;
#45339=EDGE_CURVE ( 'NONE', #40669, #38622, #37850, .T. ) ;
#45343=CARTESIAN_POINT ( 'NONE',  ( 19.65937500061451360, 2.746126346562645981, -4.756430356249997438 ) ) ;
#45358=CARTESIAN_POINT ( 'NONE',  ( 18.14999999999999858, 4.330127018922192761, -2.499999999999997780 ) ) ;
#45359=CARTESIAN_POINT ( 'NONE',  ( 21.00937500061451857, -4.119189519843965641, -2.378215178125001383 ) ) ;
#45369=ORIENTED_EDGE ( 'NONE', *, *, #25127, .T. ) ;
#45381=CARTESIAN_POINT ( 'NONE',  ( 7.771875000614516082, 2.746126346562643317, 4.756430356249998326 ) ) ;
#45399=EDGE_CURVE ( 'NONE', #54432, #1846, #60482, .T. ) ;
#45401=CARTESIAN_POINT ( 'NONE',  ( 17.86875000122903501, 2.886751345948126879, 4.999999999999998224 ) ) ;
#45402=CARTESIAN_POINT ( 'NONE',  ( 9.196875000614518569, -2.746126346562646425, 4.756430356249996549 ) ) ;
#45414=CARTESIAN_POINT ( 'NONE',  ( 12.73125000122903394, 6.123233995736764310E-16, -4.999999999999998224 ) ) ;
#45425=CARTESIAN_POINT ( 'NONE',  ( 17.14687500061451431, 0.000000000000000000, 4.756430356249998326 ) ) ;
#45428=CARTESIAN_POINT ( 'NONE',  ( 25.35937500061451644, -5.492252693125287522, -1.008910452111647106E-15 ) ) ;
#45437=DIRECTION ( 'NONE',  ( 0.000000000000000000, 0.000000000000000000, 1.000000000000000000 ) ) ;
#45443=CARTESIAN_POINT ( 'NONE',  ( 7.359375000614517326, -5.492252693125287522, -1.008910452111647106E-15 ) ) ;
#45465=CARTESIAN_POINT ( 'NONE',  ( 15.57187500061451857, -5.492252693125287522, -1.008910452111647106E-15 ) ) ;
#45487=AXIS2_PLACEMENT_3D ( 'NONE', #23625, #40631, #46171 ) ;
#45499=CARTESIAN_POINT ( 'NONE',  ( 16.28437500061452070, 4.119189519843966529, 2.378215178124999607 ) ) ;
#45507=CARTESIAN_POINT ( 'NONE',  ( 19.79999999999999716, -4.330127018922190985, -2.500000000000001332 ) ) ;
#45510=FACE_OUTER_BOUND ( 'NONE', #31902, .T. ) ;
#45511=CARTESIAN_POINT ( 'NONE',  ( 26.59687500061451360, 0.000000000000000000, 4.756430356249998326 ) ) ;
#45518=CARTESIAN_POINT ( 'NONE',  ( 25.54687500061451644, 4.119189519843966529, -2.378215178124998275 ) ) ;
#45520=CARTESIAN_POINT ( 'NONE',  ( 10.47187500061451715, -4.119189519843968306, 2.378215178124996054 ) ) ;
#45521=AXIS2_PLACEMENT_3D ( 'NONE', #70813, #59717, #32021 ) ;
#45526=CARTESIAN_POINT ( 'NONE',  ( 8.193750001229032520, -2.886751345948181946, -4.999999999999904077 ) ) ;
#45529=ADVANCED_FACE ( 'NONE', ( #67896 ), #22453, .T. ) ;
#45531=CARTESIAN_POINT ( 'NONE',  ( 18.05625000122903501, -4.330127018922190985, -2.500000000000001332 ) ) ;
#45532=CARTESIAN_POINT ( 'NONE',  ( 10.16250000000000320, 2.886751345948126879, 4.999999999999998224 ) ) ;
#45535=CARTESIAN_POINT ( 'NONE',  ( 13.35937500061451644, 2.746126346562645981, -4.756430356249997438 ) ) ;
#45555=CARTESIAN_POINT ( 'NONE',  ( 20.78437500061451715, 4.119189519843966529, 2.378215178124999607 ) ) ;
#45567=CARTESIAN_POINT ( 'NONE',  ( 17.30625000122903145, 4.330127018922192761, -2.499999999999997780 ) ) ;
#45575=CARTESIAN_POINT ( 'NONE',  ( 15.95625000122903181, 4.330127018922192761, -2.499999999999997780 ) ) ;
#45589=CARTESIAN_POINT ( 'NONE',  ( 25.13437500061451502, 5.824947211148865298E-16, -4.756430356249998326 ) ) ;
#45595=EDGE_CURVE ( 'NONE', #25370, #675, #38727, .T. ) ;
#45597=CARTESIAN_POINT ( 'NONE',  ( 28.08749999999999858, 5.773502691896255534, 3.535250795749688894E-16 ) ) ;
#45605=CARTESIAN_POINT ( 'NONE',  ( 9.093750001229032875, -2.886751345948125991, -5.000000000000000000 ) ) ;
#45608=CARTESIAN_POINT ( 'NONE',  ( 18.75937500061451857, 2.746126346562645981, -4.756430356249997438 ) ) ;
#45615=CARTESIAN_POINT ( 'NONE',  ( 27.86249999999999716, -5.773502691896255534, -1.060575238724906372E-15 ) ) ;
#45620=CARTESIAN_POINT ( 'NONE',  ( 13.09687500061451715, 0.000000000000000000, 4.756430356249998326 ) ) ;
#45642=CARTESIAN_POINT ( 'NONE',  ( 28.62187500061451573, -5.492252693125287522, -1.008910452111647106E-15 ) ) ;
#45644=CARTESIAN_POINT ( 'NONE',  ( 22.51875000122903003, -5.773502691896255534, -1.060575238724906372E-15 ) ) ;
#45645=CARTESIAN_POINT ( 'NONE',  ( 13.35937500061451821, -4.119189519843965641, -2.378215178125001383 ) ) ;
#45655=CARTESIAN_POINT ( 'NONE',  ( 45.00000000000000000, 0.000000000000000000, 0.000000000000000000 ) ) ;
#45662=CARTESIAN_POINT ( 'NONE',  ( 23.68125000122903145, 4.330127018922191873, 2.499999999999999556 ) ) ;
#45665=VERTEX_POINT ( 'NONE', #22094 ) ;
#45691=CARTESIAN_POINT ( 'NONE',  ( 23.81250000000000000, -5.773502691896255534, -1.060575238724906372E-15 ) ) ;
#45694=CARTESIAN_POINT ( 'NONE',  ( 26.04375000122903216, -2.886751345948143310, 4.999999999999972466 ) ) ;
#45703=EDGE_LOOP ( 'NONE', ( #60924, #60124, #28814, #57730 ) ) ;
#45709=CARTESIAN_POINT ( 'NONE',  ( 17.85937500061451644, 2.746126346562645981, -4.756430356249997438 ) ) ;
#45718=ORIENTED_EDGE ( 'NONE', *, *, #7133, .F. ) ;
#45724=CARTESIAN_POINT ( 'NONE',  ( 45.00000000000000000, 0.000000000000000000, 0.000000000000000000 ) ) ;
#45725=CARTESIAN_POINT ( 'NONE',  ( 19.69687500061451857, -2.746126346562642428, -4.756430356249999214 ) ) ;
#45746=CARTESIAN_POINT ( 'NONE',  ( 8.184375000614515727, 4.119189519843966529, 2.378215178124999607 ) ) ;
#45768=CARTESIAN_POINT ( 'NONE',  ( 8.671875000614518214, 2.746126346562643317, 4.756430356249998326 ) ) ;
#45789=CARTESIAN_POINT ( 'NONE',  ( 17.07187500061451502, 4.119189519843966529, 2.378215178124999607 ) ) ;
#45792=CARTESIAN_POINT ( 'NONE',  ( 26.33437500061451431, -2.746126346562642428, -4.756430356249999214 ) ) ;
#45796=CARTESIAN_POINT ( 'NONE',  ( 26.84999999999999787, 0.000000000000000000, 4.999999999999998224 ) ) ;
#45805=CARTESIAN_POINT ( 'NONE',  ( 28.05937500061451573, 0.000000000000000000, 4.756430356249998326 ) ) ;
#45813=ORIENTED_EDGE ( 'NONE', *, *, #14306, .T. ) ;
#45823=CARTESIAN_POINT ( 'NONE',  ( 15.87187500061451573, 2.746126346562643317, 4.756430356249998326 ) ) ;
#45827=ORIENTED_EDGE ( 'NONE', *, *, #43153, .F. ) ;
#45837=ORIENTED_EDGE ( 'NONE', *, *, #43566, .T. ) ;
#45845=( BOUNDED_CURVE ( )  B_SPLINE_CURVE ( 2, ( #70789, #8003, #20164, #20526, #14999, #36805, #8365 ),
 .UNSPECIFIED., .F., .F. ) 
 B_SPLINE_CURVE_WITH_KNOTS ( ( 3, 2, 2, 3 ),
 ( 0.8800000000000000044, 0.8833333333333333037, 0.8866666666666667140, 0.8900000000000000133 ),
 .UNSPECIFIED. ) 
 CURVE ( )  GEOMETRIC_REPRESENTATION_ITEM ( )  RATIONAL_B_SPLINE_CURVE ( ( 1.000000000000000000, 0.8660254037844387076, 1.000000000000000000, 0.8660254037844387076, 1.000000000000000000, 0.8660254037844387076, 1.000000000000000000 ) ) 
 REPRESENTATION_ITEM ( '' )  );
#45854=CARTESIAN_POINT ( 'NONE',  ( 16.84687500061451715, -2.746126346562646425, 4.756430356249996549 ) ) ;
#45855=CARTESIAN_POINT ( 'NONE',  ( 14.71875000122903288, 2.886751345948126879, 4.999999999999998224 ) ) ;
#45861=CARTESIAN_POINT ( 'NONE',  ( 18.37500000000000355, -4.330127018922194537, 2.499999999999995559 ) ) ;
#45865=CARTESIAN_POINT ( 'NONE',  ( 26.40937500061451360, 2.746126346562645981, -4.756430356249997438 ) ) ;
#45869=CARTESIAN_POINT ( 'NONE',  ( 29.92968750030725644, 0.000000000000000000, 4.878215178124998275 ) ) ;
#45873=CARTESIAN_POINT ( 'NONE',  ( 25.84687500061451360, -4.119189519843965641, -2.378215178125001383 ) ) ;
#45876=CARTESIAN_POINT ( 'NONE',  ( 10.24687500061451395, 4.119189519843966529, -2.378215178124998275 ) ) ;
#45884=CARTESIAN_POINT ( 'NONE',  ( 26.23125000122903216, 6.123233995736764310E-16, -4.999999999999998224 ) ) ;
#45885=CARTESIAN_POINT ( 'NONE',  ( 17.77499999999999858, 4.330127018922191873, 2.499999999999999556 ) ) ;
#45886=ORIENTED_EDGE ( 'NONE', *, *, #67290, .T. ) ;
#45888=CARTESIAN_POINT ( 'NONE',  ( 12.23437500061451644, -2.746126346562646425, 4.756430356249996549 ) ) ;
#45908=CARTESIAN_POINT ( 'NONE',  ( 23.07187500061452212, 2.746126346562643317, 4.756430356249998326 ) ) ;
#45915=ORIENTED_EDGE ( 'NONE', *, *, #10750, .F. ) ;
#45928=CARTESIAN_POINT ( 'NONE',  ( 17.38125000122903074, 4.330127018922191873, 2.499999999999999556 ) ) ;
#45941=ORIENTED_EDGE ( 'NONE', *, *, #3480, .T. ) ;
#45945=CARTESIAN_POINT ( 'NONE',  ( 23.78437500061451360, 5.824947211148865298E-16, -4.756430356249998326 ) ) ;
#45951=CARTESIAN_POINT ( 'NONE',  ( 24.82499999999999929, 6.123233995736764310E-16, -4.999999999999998224 ) ) ;
#45959=CARTESIAN_POINT ( 'NONE',  ( 9.731250001229033941, 4.330127018922191873, 2.499999999999999556 ) ) ;
#45963=CARTESIAN_POINT ( 'NONE',  ( 18.34687500061451360, 4.119189519843966529, -2.378215178124998275 ) ) ;
#45974=CARTESIAN_POINT ( 'NONE',  ( 10.50937500061451502, -5.492252693125287522, -1.008910452111647106E-15 ) ) ;
#45981=CARTESIAN_POINT ( 'NONE',  ( 19.76249999999999929, -5.773502691896255534, -1.060575238724906372E-15 ) ) ;
#45998=CARTESIAN_POINT ( 'NONE',  ( 28.24687500061451217, 4.119189519843966529, -2.378215178124998275 ) ) ;
#45999=CARTESIAN_POINT ( 'NONE',  ( 12.87187500061451750, -5.492252693125287522, -1.008910452111647106E-15 ) ) ;
#46012=DIRECTION ( 'NONE',  ( 1.000000000000000000, 0.000000000000000000, 0.000000000000000000 ) ) ;
#46017=CARTESIAN_POINT ( 'NONE',  ( 24.24375000122903145, -2.886751345948129988, 4.999999999999997335 ) ) ;
#46042=CARTESIAN_POINT ( 'NONE',  ( -4.999999999999998224, 2.928932188134522718, -4.999999999999998224 ) ) ;
#46047=CYLINDRICAL_SURFACE ( 'NONE', #5602, 4.999999999999998224 ) ;
#46057=CARTESIAN_POINT ( 'NONE',  ( 29.55000000000000071, 0.000000000000000000, 4.999999999999998224 ) ) ;
#46067=CARTESIAN_POINT ( 'NONE',  ( 19.84687500061451360, 0.000000000000000000, 4.756430356249998326 ) ) ;
#46084=CARTESIAN_POINT ( 'NONE',  ( 20.55937500061451573, -4.119189519843965641, -2.378215178125001383 ) ) ;
#46101=CARTESIAN_POINT ( 'NONE',  ( 20.86875000122903145, 2.886751345948129099, -4.999999999999997335 ) ) ;
#46106=CARTESIAN_POINT ( 'NONE',  ( 22.78125000122903288, 4.330127018922191873, 2.499999999999999556 ) ) ;
#46127=CARTESIAN_POINT ( 'NONE',  ( 8.596875000614518925, 5.492252693125287522, 3.363034840372157021E-16 ) ) ;
#46129=CARTESIAN_POINT ( 'NONE',  ( 23.25000000000000000, 0.000000000000000000, 4.999999999999998224 ) ) ;
#46133=EDGE_CURVE ( 'NONE', #50673, #32393, #29831, .T. ) ;
#46137=CARTESIAN_POINT ( 'NONE',  ( 15.65625000122903465, 0.000000000000000000, 4.999999999999998224 ) ) ;
#46147=CARTESIAN_POINT ( 'NONE',  ( 17.52187500061451431, 4.119189519843966529, 2.378215178124999607 ) ) ;
#46150=CARTESIAN_POINT ( 'NONE',  ( 26.97187500061451360, 4.119189519843966529, 2.378215178124999607 ) ) ;
#46154=CARTESIAN_POINT ( 'NONE',  ( 26.88749999999999929, -2.886751345948130876, 4.999999999999996447 ) ) ;
#46158=DIRECTION ( 'NONE',  ( 0.000000000000000000, 0.000000000000000000, 1.000000000000000000 ) ) ;
#46164=CARTESIAN_POINT ( 'NONE',  ( 28.28437500061451715, 5.824947211148865298E-16, -4.756430356249998326 ) ) ;
#46169=ADVANCED_FACE ( 'NONE', ( #42380 ), #12482, .T. ) ;
#46171=DIRECTION ( 'NONE',  ( 0.000000000000000000, 0.000000000000000000, 1.000000000000000000 ) ) ;
#46173=ORIENTED_EDGE ( 'NONE', *, *, #35222, .F. ) ;
#46183=CARTESIAN_POINT ( 'NONE',  ( 14.29687500061451821, -2.746126346562641984, -4.756430356249999214 ) ) ;
#46196=VERTEX_POINT ( 'NONE', #25008 ) ;
#46214=CARTESIAN_POINT ( 'NONE',  ( 16.95937500061451786, -4.119189519843965641, -2.378215178125001383 ) ) ;
#46221=CARTESIAN_POINT ( 'NONE',  ( 18.30000000000000071, 0.000000000000000000, 4.999999999999998224 ) ) ;
#46225=CARTESIAN_POINT ( 'NONE',  ( 24.12187500061451573, 5.824947211148865298E-16, -4.756430356249998326 ) ) ;
#46232=CARTESIAN_POINT ( 'NONE',  ( 25.20937500061451431, 2.746126346562643317, 4.756430356249998326 ) ) ;
#46234=CARTESIAN_POINT ( 'NONE',  ( 11.74687500061451573, 0.000000000000000000, 4.756430356249998326 ) ) ;
#46239=CARTESIAN_POINT ( 'NONE',  ( 29.38125000122903074, 6.123233995736764310E-16, -4.999999999999998224 ) ) ;
#46244=VERTEX_POINT ( 'NONE', #52727 ) ;
#46246=CARTESIAN_POINT ( 'NONE',  ( 12.60937500061451289, 2.746126346562643317, 4.756430356249998326 ) ) ;
#46267=CARTESIAN_POINT ( 'NONE',  ( 21.42187500061451644, -5.492252693125287522, -1.008910452111647106E-15 ) ) ;
#46285=CARTESIAN_POINT ( 'NONE',  ( 15.73125000122903216, -4.330127018922194537, 2.499999999999995559 ) ) ;
#46302=CARTESIAN_POINT ( 'NONE',  ( 24.04687500061451644, -2.746126346562646425, 4.756430356249996549 ) ) ;
#46306=EDGE_CURVE ( 'NONE', #23351, #829, #43511, .T. ) ;
#46309=CARTESIAN_POINT ( 'NONE',  ( 24.41250000000000142, 2.886751345948129099, -4.999999999999998224 ) ) ;
#46319=CARTESIAN_POINT ( 'NONE',  ( 22.85625000122903216, 0.000000000000000000, 4.999999999999998224 ) ) ;
#46321=CARTESIAN_POINT ( 'NONE',  ( 8.418750001229032165, 2.886751345948126879, 4.999999999999999112 ) ) ;
#46324=CARTESIAN_POINT ( 'NONE',  ( 17.33437500061451431, -2.746126346562641984, -4.756430356249999214 ) ) ;
#46331=EDGE_CURVE ( 'NONE', #53529, #23511, #25752, .T. ) ;
#46335=FACE_OUTER_BOUND ( 'NONE', #72108, .T. ) ;
#46336=CARTESIAN_POINT ( 'NONE',  ( 10.84687500061451715, 0.000000000000000000, 4.756430356249998326 ) ) ;
#46349=CARTESIAN_POINT ( 'NONE',  ( 11.77500000000000036, 6.123233995736764310E-16, -4.999999999999998224 ) ) ;
#46352=EDGE_LOOP ( 'NONE', ( #23152, #4067, #27274, #56422 ) ) ;
#46358=CARTESIAN_POINT ( 'NONE',  ( 28.58437500061451786, -4.119189519843968306, 2.378215178124996054 ) ) ;
#46360=CARTESIAN_POINT ( 'NONE',  ( 27.49687500061451573, 0.000000000000000000, 4.756430356249998326 ) ) ;
#46361=CARTESIAN_POINT ( 'NONE',  ( 13.50937500061451679, 4.119189519843966529, -2.378215178124998275 ) ) ;
#46368=CYLINDRICAL_SURFACE ( 'NONE', #59596, 4.999999999999998224 ) ;
#46377=CARTESIAN_POINT ( 'NONE',  ( 23.86875000122903501, -5.773502691896255534, -1.060575238724906372E-15 ) ) ;
#46405=ADVANCED_FACE ( 'NONE', ( #26114 ), #71178, .T. ) ;
#46410=CARTESIAN_POINT ( 'NONE',  ( 19.29375000122903927, -2.886751345948130876, 4.999999999999996447 ) ) ;
#46427=CARTESIAN_POINT ( 'NONE',  ( 19.17187500061451289, 5.824947211148865298E-16, -4.756430356249998326 ) ) ;
#46440=ADVANCED_FACE ( 'NONE', ( #43479 ), #9124, .T. ) ;
#46445=CARTESIAN_POINT ( 'NONE',  ( 19.50937500061451857, 0.000000000000000000, 4.756430356249998326 ) ) ;
#46463=CARTESIAN_POINT ( 'NONE',  ( 20.83125000122903359, 6.123233995736764310E-16, -4.999999999999998224 ) ) ;
#46464=EDGE_CURVE ( 'NONE', #56819, #44169, #71338, .T. ) ;
#46489=CARTESIAN_POINT ( 'NONE',  ( 9.871875000614517504, 2.746126346562645981, -4.756430356249997438 ) ) ;
#46491=CARTESIAN_POINT ( 'NONE',  ( 20.30625000122903145, -4.330127018922190985, -2.500000000000001332 ) ) ;
#46501=CARTESIAN_POINT ( 'NONE',  ( 9.525000000000002132, 6.123233995736764310E-16, -4.999999999999998224 ) ) ;
#46509=CARTESIAN_POINT ( 'NONE',  ( 17.55937500061451573, 2.746126346562643317, 4.756430356249998326 ) ) ;
#46512=CARTESIAN_POINT ( 'NONE',  ( 26.25937500061451502, -5.492252693125287522, -1.008910452111647106E-15 ) ) ;
#46520=FACE_OUTER_BOUND ( 'NONE', #13203, .T. ) ;
#46527=CARTESIAN_POINT ( 'NONE',  ( 26.97187500061451360, 2.746126346562645981, -4.756430356249997438 ) ) ;
#46546=CARTESIAN_POINT ( 'NONE',  ( 13.95937500061451786, 4.119189519843966529, -2.378215178124998275 ) ) ;
#46559=ORIENTED_EDGE ( 'NONE', *, *, #36894, .T. ) ;
#46574=AXIS2_PLACEMENT_3D ( 'NONE', #7591, #13126, #7958 ) ;
#46576=CARTESIAN_POINT ( 'NONE',  ( 15.34687500061451537, 5.492252693125287522, 3.363034840372157021E-16 ) ) ;
#46580=EDGE_CURVE ( 'NONE', #21751, #67801, #15384, .T. ) ;
#46584=CARTESIAN_POINT ( 'NONE',  ( 18.48750000000000071, -2.886751345948125991, -5.000000000000000000 ) ) ;
#46589=CARTESIAN_POINT ( 'NONE',  ( 23.33437500061451786, 5.492252693125287522, 3.363034840372157021E-16 ) ) ;
#46596=CARTESIAN_POINT ( 'NONE',  ( 24.12187500061451573, 5.824947211148865298E-16, -4.756430356249998326 ) ) ;
#46598=CARTESIAN_POINT ( 'NONE',  ( 10.20937500061451431, 2.746126346562645981, -4.756430356249997438 ) ) ;
#46606=CARTESIAN_POINT ( 'NONE',  ( 17.73750000000000071, 5.773502691896255534, 3.535250795749688401E-16 ) ) ;
#46609=CARTESIAN_POINT ( 'NONE',  ( 10.92187500061451644, -4.119189519843968306, 2.378215178124996054 ) ) ;
#46616=CARTESIAN_POINT ( 'NONE',  ( 0.000000000000000000, -4.999999999999999112, 0.000000000000000000 ) ) ;
#46620=AXIS2_PLACEMENT_3D ( 'NONE', #45655, #39755, #57794 ) ;
#46626=CARTESIAN_POINT ( 'NONE',  ( 12.05625000122903145, 0.000000000000000000, 4.999999999999998224 ) ) ;
#46629=CARTESIAN_POINT ( 'NONE',  ( 21.34687500061451715, -2.746126346562646425, 4.756430356249996549 ) ) ;
#46639=VECTOR ( 'NONE', #16426, 1000.000000000000000 ) ;
#46667=CARTESIAN_POINT ( 'NONE',  ( 22.95937500061451431, 4.119189519843966529, -2.378215178124998275 ) ) ;
#46670=CARTESIAN_POINT ( 'NONE',  ( 29.09999999999999787, 0.000000000000000000, 4.999999999999998224 ) ) ;
#46674=CARTESIAN_POINT ( 'NONE',  ( 24.86250000000000071, 2.886751345948129099, -4.999999999999998224 ) ) ;
#46679=CARTESIAN_POINT ( 'NONE',  ( 24.52499999999999858, 4.330127018922191873, 2.499999999999999556 ) ) ;
#46684=CARTESIAN_POINT ( 'NONE',  ( 9.393750001229035362, -2.886751345948129988, 4.999999999999997335 ) ) ;
#46687=CARTESIAN_POINT ( 'NONE',  ( 18.57187500061451857, -4.119189519843968306, 2.378215178124996054 ) ) ;
#46691=ORIENTED_EDGE ( 'NONE', *, *, #8082, .F. ) ;
#46700=CARTESIAN_POINT ( 'NONE',  ( 10.09687500061451715, -4.119189519843965641, -2.378215178125001383 ) ) ;
#46714=CARTESIAN_POINT ( 'NONE',  ( 9.975000000000001421, 6.123233995736764310E-16, -4.999999999999998224 ) ) ;
#46722=CARTESIAN_POINT ( 'NONE',  ( 29.18437500061451573, 5.824947211148865298E-16, -4.756430356249998326 ) ) ;
#46724=CARTESIAN_POINT ( 'NONE',  ( 27.75937500061451502, 2.746126346562645981, -4.756430356249997438 ) ) ;
#46725=CARTESIAN_POINT ( 'NONE',  ( 12.49687500061451573, -2.746126346562642428, -4.756430356249999214 ) ) ;
#46732=( BOUNDED_CURVE ( )  B_SPLINE_CURVE ( 2, ( #21138, #3806, #15232, #37770, #4172, #442, #28159 ),
 .UNSPECIFIED., .F., .F. ) 
 B_SPLINE_CURVE_WITH_KNOTS ( ( 3, 2, 2, 3 ),
 ( 0.4900000000000001021, 0.4933333333333334569, 0.4966666666666667562, 0.5000000000000001110 ),
 .UNSPECIFIED. ) 
 CURVE ( )  GEOMETRIC_REPRESENTATION_ITEM ( )  RATIONAL_B_SPLINE_CURVE ( ( 0.9999999999999955591, 0.8660254037844431485, 1.000000000000000000, 0.8660254037844387076, 1.000000000000000000, 0.8660254037844342667, 1.000000000000004441 ) ) 
 REPRESENTATION_ITEM ( '' )  );
#46737=( LENGTH_UNIT ( ) NAMED_UNIT ( * ) SI_UNIT ( .MILLI., .METRE. ) );
#46742=CARTESIAN_POINT ( 'NONE',  ( 24.54375000122903572, 5.773502691896255534, 3.535250795749688894E-16 ) ) ;
#46745=ORIENTED_EDGE ( 'NONE', *, *, #73012, .T. ) ;
#46750=CARTESIAN_POINT ( 'NONE',  ( 28.91250000000000497, 2.886751345948104674, -5.000000000000039968 ) ) ;
#46782=LINE ( 'NONE', #69317, #46639 ) ;
#46786=ORIENTED_EDGE ( 'NONE', *, *, #63206, .T. ) ;
#46792=CARTESIAN_POINT ( 'NONE',  ( 15.68437500061451750, 5.492252693125287522, 3.363034840372157021E-16 ) ) ;
#46808=DIRECTION ( 'NONE',  ( 0.000000000000000000, 0.000000000000000000, 1.000000000000000000 ) ) ;
#46811=CARTESIAN_POINT ( 'NONE',  ( 20.07187500061451857, -5.492252693125287522, -1.008910452111647106E-15 ) ) ;
#46823=DIRECTION ( 'NONE',  ( 0.000000000000000000, 0.000000000000000000, 1.000000000000000000 ) ) ;
#46834=CARTESIAN_POINT ( 'NONE',  ( 14.77500000000000036, -4.330127018922194537, 2.499999999999995559 ) ) ;
#46854=CARTESIAN_POINT ( 'NONE',  ( 27.80625000122903145, 0.000000000000000000, 4.999999999999998224 ) ) ;
#46855=CARTESIAN_POINT ( 'NONE',  ( 9.721875000614517148, -5.492252693125287522, -1.008910452111647106E-15 ) ) ;
#46859=EDGE_CURVE ( 'NONE', #27013, #47688, #21293, .T. ) ;
#46874=CARTESIAN_POINT ( 'NONE',  ( 14.37187500061451573, 4.119189519843966529, 2.378215178124999607 ) ) ;
#46877=CARTESIAN_POINT ( 'NONE',  ( 25.13437500061451857, 5.492252693125287522, 3.363034840372157021E-16 ) ) ;
#46885=DIRECTION ( 'NONE',  ( -1.000000000000000000, -0.000000000000000000, -0.000000000000000000 ) ) ;
#46892=CARTESIAN_POINT ( 'NONE',  ( 28.32187500061451502, 2.746126346562645981, -4.756430356249997438 ) ) ;
#46896=CYLINDRICAL_SURFACE ( 'NONE', #20808, 4.999999999999998224 ) ;
#46910=CARTESIAN_POINT ( 'NONE',  ( 11.22187500061451892, 2.746126346562645981, -4.756430356249997438 ) ) ;
#46931=VECTOR ( 'NONE', #6191, 1000.000000000000000 ) ;
#46943=CARTESIAN_POINT ( 'NONE',  ( 15.94687500061451502, -2.746126346562646425, 4.756430356249996549 ) ) ;
#46949=CARTESIAN_POINT ( 'NONE',  ( 18.14999999999999858, 4.330127018922192761, -2.499999999999997780 ) ) ;
#46953=CARTESIAN_POINT ( 'NONE',  ( 22.65937500061451004, -5.492252693125287522, -1.008910452111647106E-15 ) ) ;
#46954=VERTEX_POINT ( 'NONE', #50480 ) ;
#46957=LINE ( 'NONE', #1535, #52842 ) ;
#46961=CARTESIAN_POINT ( 'NONE',  ( 25.09687500061451360, 4.119189519843966529, -2.378215178124998275 ) ) ;
#46963=CARTESIAN_POINT ( 'NONE',  ( 9.684375000614517504, -2.746126346562641984, -4.756430356249999214 ) ) ;
#46966=ORIENTED_EDGE ( 'NONE', *, *, #7459, .F. ) ;
#46971=CARTESIAN_POINT ( 'NONE',  ( 19.34999999999999787, -4.330127018922190985, -2.500000000000001332 ) ) ;
#46972=DIRECTION ( 'NONE',  ( -1.000000000000000000, 0.000000000000000000, 0.000000000000000000 ) ) ;
#46975=CARTESIAN_POINT ( 'NONE',  ( 12.30937500061451750, -5.492252693125287522, -1.008910452111647106E-15 ) ) ;
#46991=CARTESIAN_POINT ( 'NONE',  ( 29.81249999999999645, 2.886751345948139313, -4.999999999999980460 ) ) ;
#46993=CARTESIAN_POINT ( 'NONE',  ( 19.13437500061451857, -4.119189519843968306, 2.378215178124996054 ) ) ;
#47028=CARTESIAN_POINT ( 'NONE',  ( 23.59687500061451715, -2.746126346562646425, 4.756430356249996549 ) ) ;
#47034=CARTESIAN_POINT ( 'NONE',  ( 24.03750000000000142, 5.773502691896255534, 3.535250795749688894E-16 ) ) ;
#47044=CARTESIAN_POINT ( 'NONE',  ( 8.306250001229031454, 4.330127018922192761, -2.499999999999997780 ) ) ;
#47047=CARTESIAN_POINT ( 'NONE',  ( 19.35937500061451289, 2.746126346562643317, 4.756430356249998326 ) ) ;
#47050=ORIENTED_EDGE ( 'NONE', *, *, #69367, .T. ) ;
#47059=CARTESIAN_POINT ( 'NONE',  ( 9.496875000614517504, 0.000000000000000000, 4.756430356249998326 ) ) ;
#47066=CARTESIAN_POINT ( 'NONE',  ( 10.20000000000000107, 0.000000000000000000, 4.999999999999998224 ) ) ;
#47070=CARTESIAN_POINT ( 'NONE',  ( 28.13437500061451502, -2.746126346562642428, -4.756430356249999214 ) ) ;
#47073=CARTESIAN_POINT ( 'NONE',  ( 8.699999999999999289, 4.330127018922192761, -2.499999999999997780 ) ) ;
#47083=CARTESIAN_POINT ( 'NONE',  ( 27.34687500061451360, 4.119189519843966529, -2.378215178124998275 ) ) ;
#47084=CARTESIAN_POINT ( 'NONE',  ( 10.39687500061451786, 5.492252693125287522, 3.363034840372157021E-16 ) ) ;
#47095=( NAMED_UNIT ( * ) PLANE_ANGLE_UNIT ( ) SI_UNIT ( $, .RADIAN. ) );
#47100=CARTESIAN_POINT ( 'NONE',  ( 20.90625000122903288, 4.330127018922192761, -2.499999999999997780 ) ) ;
#47115=CARTESIAN_POINT ( 'NONE',  ( 29.70937500061451431, 4.119189519843966529, -2.378215178124998275 ) ) ;
#47123=CYLINDRICAL_SURFACE ( 'NONE', #46574, 4.999999999999998224 ) ;
#47133=CARTESIAN_POINT ( 'NONE',  ( 7.724999999999999645, 6.123233995736764310E-16, -4.999999999999998224 ) ) ;
#47141=DIRECTION ( 'NONE',  ( -1.000000000000000000, -0.000000000000000000, -0.000000000000000000 ) ) ;
#47145=VERTEX_POINT ( 'NONE', #10948 ) ;
#47152=CARTESIAN_POINT ( 'NONE',  ( 15.38437500061451679, -2.746126346562646425, 4.756430356249996549 ) ) ;
#47170=CARTESIAN_POINT ( 'NONE',  ( 27.75000000000000000, 0.000000000000000000, 4.999999999999998224 ) ) ;
#47171=CARTESIAN_POINT ( 'NONE',  ( 17.52187500061451431, 2.746126346562645981, -4.756430356249997438 ) ) ;
#47181=DIRECTION ( 'NONE',  ( -1.000000000000000000, -0.000000000000000000, -0.000000000000000000 ) ) ;
#47188=FACE_OUTER_BOUND ( 'NONE', #3969, .T. ) ;
#47213=CARTESIAN_POINT ( 'NONE',  ( 28.35000000000000142, -4.330127018922190985, -2.500000000000001332 ) ) ;
#47220=CARTESIAN_POINT ( 'NONE',  ( 28.74375000122903501, -2.886751345948095349, 5.000000000000058620 ) ) ;
#47223=CARTESIAN_POINT ( 'NONE',  ( 15.61875000122903323, 2.886751345948126879, 4.999999999999998224 ) ) ;
#47231=CARTESIAN_POINT ( 'NONE',  ( 15.45937500061451608, -5.492252693125287522, -1.008910452111647106E-15 ) ) ;
#47234=CARTESIAN_POINT ( 'NONE',  ( 22.92187500061451644, 4.119189519843966529, 2.378215178124999607 ) ) ;
#47250=CARTESIAN_POINT ( 'NONE',  ( 28.13437500061451502, -4.119189519843968306, 2.378215178124996054 ) ) ;
#47253=CARTESIAN_POINT ( 'NONE',  ( 45.00000000000000000, 0.000000000000000000, 0.000000000000000000 ) ) ;
#47260=ORIENTED_EDGE ( 'NONE', *, *, #30226, .F. ) ;
#47269=CARTESIAN_POINT ( 'NONE',  ( 13.05937500061451750, 4.119189519843966529, -2.378215178124998275 ) ) ;
#47275=EDGE_CURVE ( 'NONE', #53798, #39431, #56017, .T. ) ;
#47298=CARTESIAN_POINT ( 'NONE',  ( 13.84687500061451537, -2.746126346562642428, -4.756430356249999214 ) ) ;
#47305=CARTESIAN_POINT ( 'NONE',  ( 16.64999999999999858, -4.330127018922190985, -2.500000000000001332 ) ) ;
#47309=CARTESIAN_POINT ( 'NONE',  ( 22.32187500061451502, 5.824947211148865298E-16, -4.756430356249998326 ) ) ;
#47314=EDGE_CURVE ( 'NONE', #61022, #68363, #53421, .T. ) ;
#47318=CARTESIAN_POINT ( 'NONE',  ( 22.28437500061451360, -2.746126346562642428, -4.756430356249999214 ) ) ;
#47320=CARTESIAN_POINT ( 'NONE',  ( 7.809375000614515727, -5.492252693125287522, -1.008910452111647106E-15 ) ) ;
#47327=CARTESIAN_POINT ( 'NONE',  ( 26.30625000122903145, 4.330127018922192761, -2.499999999999997780 ) ) ;
#47331=CARTESIAN_POINT ( 'NONE',  ( 12.12187500061451573, 4.119189519843966529, 2.378215178124999607 ) ) ;
#47349=CARTESIAN_POINT ( 'NONE',  ( 11.43750000000000000, 5.773502691896255534, 3.535250795749688401E-16 ) ) ;
#47352=CARTESIAN_POINT ( 'NONE',  ( 18.87187500061452283, 2.746126346562645981, -4.756430356249997438 ) ) ;
#47375=DIRECTION ( 'NONE',  ( -1.000000000000000000, -0.000000000000000000, -0.000000000000000000 ) ) ;
#47388=CARTESIAN_POINT ( 'NONE',  ( 22.43437500061451573, 5.824947211148865298E-16, -4.756430356249998326 ) ) ;
#47394=CARTESIAN_POINT ( 'NONE',  ( 23.81250000000000000, -5.773502691896255534, -1.060575238724906372E-15 ) ) ;
#47398=CARTESIAN_POINT ( 'NONE',  ( 7.106250001229032165, 0.000000000000000000, 4.999999999999998224 ) ) ;
#47399=CARTESIAN_POINT ( 'NONE',  ( 18.76875000122903003, 2.886751345948098901, 5.000000000000047073 ) ) ;
#47405=CARTESIAN_POINT ( 'NONE',  ( 29.70937500061451431, 2.746126346562643317, 4.756430356249998326 ) ) ;
#47407=CARTESIAN_POINT ( 'NONE',  ( 16.24687500061451573, 0.000000000000000000, 4.756430356249998326 ) ) ;
#47410=ORIENTED_EDGE ( 'NONE', *, *, #8310, .T. ) ;
#47419=CARTESIAN_POINT ( 'NONE',  ( 11.63437500061451502, 5.492252693125287522, 3.363034840372157021E-16 ) ) ;
#47429=CARTESIAN_POINT ( 'NONE',  ( 27.45937500061451431, 2.746126346562643317, 4.756430356249998326 ) ) ;
#47432=CARTESIAN_POINT ( 'NONE',  ( 8.025000000000000355, -4.330127018922194537, 2.499999999999995559 ) ) ;
#47440=CARTESIAN_POINT ( 'NONE',  ( 27.34687500061451360, -2.746126346562641984, -4.756430356249999214 ) ) ;
#47442=CARTESIAN_POINT ( 'NONE',  ( 9.609375000614518214, 0.000000000000000000, 4.756430356249998326 ) ) ;
#47450=LINE ( 'NONE', #30094, #1809 ) ;
#47457=CARTESIAN_POINT ( 'NONE',  ( 21.61875000122903145, -5.773502691896255534, -1.060575238724906372E-15 ) ) ;
#47475=EDGE_CURVE ( 'NONE', #17152, #27917, #69634, .T. ) ;
#47505=( BOUNDED_CURVE ( )  B_SPLINE_CURVE ( 2, ( #70477, #37585, #48315, #54581, #25406, #71203, #9877 ),
 .UNSPECIFIED., .F., .F. ) 
 B_SPLINE_CURVE_WITH_KNOTS ( ( 3, 2, 2, 3 ),
 ( 0.1300000000000000322, 0.1333333333333333592, 0.1366666666666666585, 0.1400000000000000133 ),
 .UNSPECIFIED. ) 
 CURVE ( )  GEOMETRIC_REPRESENTATION_ITEM ( )  RATIONAL_B_SPLINE_CURVE ( ( 0.9999999999999988898, 0.8660254037844398178, 1.000000000000000000, 0.8660254037844387076, 1.000000000000000000, 0.8660254037844387076, 1.000000000000000000 ) ) 
 REPRESENTATION_ITEM ( '' )  );
#47508=( GEOMETRIC_REPRESENTATION_CONTEXT ( 3 ) GLOBAL_UNCERTAINTY_ASSIGNED_CONTEXT ( ( #35121 ) ) GLOBAL_UNIT_ASSIGNED_CONTEXT ( ( #24909, #47095, #13829 ) ) REPRESENTATION_CONTEXT ( 'NONE', 'WORKASPACE' ) );
#47512=CARTESIAN_POINT ( 'NONE',  ( 16.69687500061451502, 0.000000000000000000, 4.756430356249998326 ) ) ;
#47527=CARTESIAN_POINT ( 'NONE',  ( 45.00000000000000000, -2.499999999999999556, -3.499999999999999556 ) ) ;
#47528=CARTESIAN_POINT ( 'NONE',  ( 45.00000000000000000, 0.000000000000000000, 4.999999999999998224 ) ) ;
#47532=CARTESIAN_POINT ( 'NONE',  ( 18.00937500061451502, 4.119189519843966529, -2.378215178124998275 ) ) ;
#47543=ORIENTED_EDGE ( 'NONE', *, *, #27431, .F. ) ;
#47548=CARTESIAN_POINT ( 'NONE',  ( 28.89375000122903003, -2.886751345948125991, -5.000000000000000000 ) ) ;
#47550=CARTESIAN_POINT ( 'NONE',  ( 8.625000000000000000, 6.123233995736764310E-16, -4.999999999999998224 ) ) ;
#47551=DIRECTION ( 'NONE',  ( 0.000000000000000000, 0.000000000000000000, 1.000000000000000000 ) ) ;
#47563=FACE_OUTER_BOUND ( 'NONE', #39204, .T. ) ;
#47574=CARTESIAN_POINT ( 'NONE',  ( 29.36250000000000071, 2.886751345948129099, -4.999999999999998224 ) ) ;
#47593=CARTESIAN_POINT ( 'NONE',  ( 16.24687500061451573, 0.000000000000000000, 4.756430356249998326 ) ) ;
#47596=CARTESIAN_POINT ( 'NONE',  ( 23.33437500061451786, 5.492252693125287522, 3.363034840372157021E-16 ) ) ;
#47600=CARTESIAN_POINT ( 'NONE',  ( 23.92499999999999716, 6.123233995736764310E-16, -4.999999999999998224 ) ) ;
#47603=DIRECTION ( 'NONE',  ( -1.000000000000000000, -0.000000000000000000, -0.000000000000000000 ) ) ;
#47604=DIRECTION ( 'NONE',  ( -1.000000000000000000, 0.000000000000000000, 0.000000000000000000 ) ) ;
#47611=CARTESIAN_POINT ( 'NONE',  ( 24.83437500061451431, 4.119189519843966529, 2.378215178124999607 ) ) ;
#47614=CARTESIAN_POINT ( 'NONE',  ( 25.16250000000000142, -5.773502691896255534, -1.060575238724906372E-15 ) ) ;
#47620=CARTESIAN_POINT ( 'NONE',  ( 25.14375000122903359, -2.886751345948116221, 5.000000000000021316 ) ) ;
#47630=CARTESIAN_POINT ( 'NONE',  ( 12.34687500061451892, -2.746126346562646425, 4.756430356249996549 ) ) ;
#47655=ORIENTED_EDGE ( 'NONE', *, *, #31978, .T. ) ;
#47658=CARTESIAN_POINT ( 'NONE',  ( 13.77187500061451786, -5.492252693125287522, -1.008910452111647106E-15 ) ) ;
#47659=EDGE_CURVE ( 'NONE', #24506, #53197, #68546, .T. ) ;
#47665=CARTESIAN_POINT ( 'NONE',  ( 16.16250000000000142, -5.773502691896255534, -1.060575238724906372E-15 ) ) ;
#47669=CARTESIAN_POINT ( 'NONE',  ( 22.05937500061451573, 2.746126346562643317, 4.756430356249998326 ) ) ;
#47670=CARTESIAN_POINT ( 'NONE',  ( 15.59999999999999964, 0.000000000000000000, 4.999999999999998224 ) ) ;
#47677=CARTESIAN_POINT ( 'NONE',  ( 23.07187500061451502, -4.119189519843968306, 2.378215178124996054 ) ) ;
#47679=CARTESIAN_POINT ( 'NONE',  ( 8.971875000614515372, 4.119189519843966529, 2.378215178124999607 ) ) ;
#47687=CARTESIAN_POINT ( 'NONE',  ( 8.906250001229031099, 0.000000000000000000, 4.999999999999998224 ) ) ;
#47688=VERTEX_POINT ( 'NONE', #54107 ) ;
#47690=CARTESIAN_POINT ( 'NONE',  ( 8.671875000614518214, -4.119189519843968306, 2.378215178124996054 ) ) ;
#47709=CARTESIAN_POINT ( 'NONE',  ( 14.30625000122903145, 0.000000000000000000, 4.999999999999998224 ) ) ;
#47712=CARTESIAN_POINT ( 'NONE',  ( 19.99687500061451573, -2.746126346562646425, 4.756430356249996549 ) ) ;
#47714=CARTESIAN_POINT ( 'NONE',  ( 28.70625000122903003, 0.000000000000000000, 4.999999999999998224 ) ) ;
#47718=ORIENTED_EDGE ( 'NONE', *, *, #15878, .T. ) ;
#47751=CARTESIAN_POINT ( 'NONE',  ( 20.59687500061451360, -2.746126346562642428, -4.756430356249999214 ) ) ;
#47757=CARTESIAN_POINT ( 'NONE',  ( 22.46250000000000213, -5.773502691896255534, -1.060575238724906372E-15 ) ) ;
#47761=CARTESIAN_POINT ( 'NONE',  ( 45.00000000000000000, 6.123233995736764310E-16, -4.999999999999998224 ) ) ;
#47767=CARTESIAN_POINT ( 'NONE',  ( 8.006250001229034297, 0.000000000000000000, 4.999999999999998224 ) ) ;
#47769=CARTESIAN_POINT ( 'NONE',  ( 14.97187500061451537, -4.119189519843968306, 2.378215178124996054 ) ) ;
#47781=CARTESIAN_POINT ( 'NONE',  ( 7.434375000614515727, -2.746126346562642428, -4.756430356249999214 ) ) ;
#47782=ORIENTED_EDGE ( 'NONE', *, *, #65590, .T. ) ;
#47788=VECTOR ( 'NONE', #48632, 1000.000000000000000 ) ;
#47795=CARTESIAN_POINT ( 'NONE',  ( 29.07187500061451502, 5.824947211148865298E-16, -4.756430356249998326 ) ) ;
#47799=CARTESIAN_POINT ( 'NONE',  ( 7.612500000000000711, -5.773502691896255534, -1.060575238724906372E-15 ) ) ;
#47807=CARTESIAN_POINT ( 'NONE',  ( 25.69687500061451502, 5.492252693125287522, 3.363034840372157021E-16 ) ) ;
#47809=CARTESIAN_POINT ( 'NONE',  ( 11.33437500061451608, 4.119189519843966529, 2.378215178124999607 ) ) ;
#47821=SHAPE_REPRESENTATION_RELATIONSHIP ( 'NONE' , 'NONE' ,  #25944, #10934 ) ;
#47827=CARTESIAN_POINT ( 'NONE',  ( 20.41875000122903216, 2.886751345948129099, -4.999999999999998224 ) ) ;
#47829=CYLINDRICAL_SURFACE ( 'NONE', #4292, 4.999999999999998224 ) ;
#47830=ORIENTED_EDGE ( 'NONE', *, *, #48575, .F. ) ;
#47844=CARTESIAN_POINT ( 'NONE',  ( 29.44687500061451857, -2.746126346562646425, 4.756430356249996549 ) ) ;
#47862=CARTESIAN_POINT ( 'NONE',  ( 23.02499999999999858, 6.123233995736764310E-16, -4.999999999999998224 ) ) ;
#47863=CARTESIAN_POINT ( 'NONE',  ( 11.15625000122903288, 0.000000000000000000, 4.999999999999998224 ) ) ;
#47870=DIRECTION ( 'NONE',  ( -1.000000000000000000, -0.000000000000000000, -0.000000000000000000 ) ) ;
#47871=ADVANCED_FACE ( 'NONE', ( #25283 ), #47829, .T. ) ;
#47883=CARTESIAN_POINT ( 'NONE',  ( 17.59687500061451360, 0.000000000000000000, 4.756430356249998326 ) ) ;
#47886=VECTOR ( 'NONE', #17298, 1000.000000000000000 ) ;
#47893=EDGE_LOOP ( 'NONE', ( #26864, #70926, #51059, #35317 ) ) ;
#47900=FACE_OUTER_BOUND ( 'NONE', #9894, .T. ) ;
#47903=CARTESIAN_POINT ( 'NONE',  ( 17.14687500061451786, 5.492252693125287522, 3.363034840372157021E-16 ) ) ;
#47917=DIRECTION ( 'NONE',  ( -1.000000000000000000, -0.000000000000000000, -0.000000000000000000 ) ) ;
#47921=CARTESIAN_POINT ( 'NONE',  ( 28.18125000122903145, 4.330127018922191873, 2.499999999999999556 ) ) ;
#47947=CARTESIAN_POINT ( 'NONE',  ( 29.39999999999999858, 4.330127018922192761, -2.499999999999997780 ) ) ;
#47953=( BOUNDED_CURVE ( )  B_SPLINE_CURVE ( 2, ( #23042, #34128, #44147, #33773, #72215, #45230, #72575 ),
 .UNSPECIFIED., .F., .F. ) 
 B_SPLINE_CURVE_WITH_KNOTS ( ( 3, 2, 2, 3 ),
 ( 0.8900000000000000133, 0.8933333333333333126, 0.8966666666666666119, 0.9000000000000000222 ),
 .UNSPECIFIED. ) 
 CURVE ( )  GEOMETRIC_REPRESENTATION_ITEM ( )  RATIONAL_B_SPLINE_CURVE ( ( 1.000000000000000000, 0.8660254037844387076, 1.000000000000000000, 0.8660254037844387076, 1.000000000000000000, 0.8660254037844387076, 1.000000000000000000 ) ) 
 REPRESENTATION_ITEM ( '' )  );
#47965=CARTESIAN_POINT ( 'NONE',  ( 14.89687500061451608, 0.000000000000000000, 4.756430356249998326 ) ) ;
#47968=CARTESIAN_POINT ( 'NONE',  ( 24.38437500061451502, -2.746126346562646425, 4.756430356249996549 ) ) ;
#47977=AXIS2_PLACEMENT_3D ( 'NONE', #32766, #61556, #10232 ) ;
#47979=CARTESIAN_POINT ( 'NONE',  ( 11.92500000000000071, 4.330127018922191873, 2.499999999999999556 ) ) ;
#47986=CARTESIAN_POINT ( 'NONE',  ( 23.63437500061451502, -4.119189519843968306, 2.378215178124996054 ) ) ;
#47998=ORIENTED_EDGE ( 'NONE', *, *, #57780, .T. ) ;
#48007=CARTESIAN_POINT ( 'NONE',  ( 11.97187500061451892, -5.492252693125287522, -1.008910452111647106E-15 ) ) ;
#48014=ADVANCED_FACE ( 'NONE', ( #44124 ), #16751, .T. ) ;
#48021=VERTEX_POINT ( 'NONE', #39308 ) ;
#48022=ORIENTED_EDGE ( 'NONE', *, *, #1743, .F. ) ;
#48037=CARTESIAN_POINT ( 'NONE',  ( 14.59687500061452070, -2.746126346562646425, 4.756430356249996549 ) ) ;
#48045=CARTESIAN_POINT ( 'NONE',  ( 15.00000000000000000, 4.330127018922192761, -2.499999999999997780 ) ) ;
#48048=CARTESIAN_POINT ( 'NONE',  ( 45.00000000000000000, 6.123233995736764310E-16, -4.999999999999998224 ) ) ;
#48056=CARTESIAN_POINT ( 'NONE',  ( 23.29687500061451644, 4.119189519843966529, -2.378215178124998275 ) ) ;
#48058=CARTESIAN_POINT ( 'NONE',  ( 9.609375000614514661, -5.492252693125287522, -1.008910452111647106E-15 ) ) ;
#48067=CARTESIAN_POINT ( 'NONE',  ( 9.796875000614514661, 4.119189519843966529, -2.378215178124998275 ) ) ;
#48083=EDGE_CURVE ( 'NONE', #50673, #64487, #55564, .T. ) ;
#48090=VECTOR ( 'NONE', #63803, 1000.000000000000000 ) ;
#48092=CARTESIAN_POINT ( 'NONE',  ( 19.65937500061451360, -4.119189519843965641, -2.378215178125001383 ) ) ;
#48096=VERTEX_POINT ( 'NONE', #38576 ) ;
#48123=CARTESIAN_POINT ( 'NONE',  ( 20.55937500061451573, -4.119189519843965641, -2.378215178125001383 ) ) ;
#48129=CARTESIAN_POINT ( 'NONE',  ( 21.56250000000000000, -5.773502691896255534, -1.060575238724906372E-15 ) ) ;
#48136=CARTESIAN_POINT ( 'NONE',  ( 18.20625000122903003, 4.330127018922192761, -2.499999999999997780 ) ) ;
#48137=EDGE_CURVE ( 'NONE', #50673, #24022, #68967, .T. ) ;
#48139=CARTESIAN_POINT ( 'NONE',  ( 29.74687500061451573, 0.000000000000000000, 4.756430356249998326 ) ) ;
#48141=CARTESIAN_POINT ( 'NONE',  ( 16.65937500061451715, 2.746126346562643317, 4.756430356249998326 ) ) ;
#48150=CARTESIAN_POINT ( 'NONE',  ( 7.321875000614517681, -4.119189519843968306, 2.378215178124996054 ) ) ;
#48156=VERTEX_POINT ( 'NONE', #4599 ) ;
#48162=CARTESIAN_POINT ( 'NONE',  ( 29.44687500061451146, -4.119189519843965641, -2.378215178125001383 ) ) ;
#48166=CARTESIAN_POINT ( 'NONE',  ( 7.837499999999999467, 5.773502691896255534, 3.535250795749688894E-16 ) ) ;
#48174=CARTESIAN_POINT ( 'NONE',  ( 26.33437500061451431, -4.119189519843968306, 2.378215178124996054 ) ) ;
#48176=CARTESIAN_POINT ( 'NONE',  ( 10.77187500061451786, 2.746126346562645981, -4.756430356249997438 ) ) ;
#48194=CARTESIAN_POINT ( 'NONE',  ( 21.88125000122903074, 4.330127018922191873, 2.499999999999999556 ) ) ;
#48196=CARTESIAN_POINT ( 'NONE',  ( 21.46875000122903288, 2.886751345948126879, 4.999999999999998224 ) ) ;
#48210=CARTESIAN_POINT ( 'NONE',  ( 29.14687500061451075, -2.746126346562642428, -4.756430356249999214 ) ) ;
#48213=( BOUNDED_CURVE ( )  B_SPLINE_CURVE ( 2, ( #10922, #10562, #21268, #5386, #56359, #49365, #61524 ),
 .UNSPECIFIED., .F., .F. ) 
 B_SPLINE_CURVE_WITH_KNOTS ( ( 3, 2, 2, 3 ),
 ( 0.5700000000000000622, 0.5733333333333334725, 0.5766666666666667718, 0.5800000000000000711 ),
 .UNSPECIFIED. ) 
 CURVE ( )  GEOMETRIC_REPRESENTATION_ITEM ( )  RATIONAL_B_SPLINE_CURVE ( ( 0.9999999999999955591, 0.8660254037844431485, 1.000000000000000000, 0.8660254037844387076, 1.000000000000000000, 0.8660254037844342667, 1.000000000000004441 ) ) 
 REPRESENTATION_ITEM ( '' )  );
#48219=CARTESIAN_POINT ( 'NONE',  ( 28.42499999999999716, 6.123233995736764310E-16, -4.999999999999998224 ) ) ;
#48233=FACE_OUTER_BOUND ( 'NONE', #6572, .T. ) ;
#48245=CARTESIAN_POINT ( 'NONE',  ( 11.70000000000000284, -4.330127018922190985, -2.500000000000001332 ) ) ;
#48248=CARTESIAN_POINT ( 'NONE',  ( 16.32187500061451502, -4.119189519843968306, 2.378215178124996054 ) ) ;
#48265=CARTESIAN_POINT ( 'NONE',  ( 14.10000000000000142, 4.330127018922192761, -2.499999999999997780 ) ) ;
#48269=CARTESIAN_POINT ( 'NONE',  ( 18.42187500061451644, 2.746126346562645981, -4.756430356249997438 ) ) ;
#48287=CARTESIAN_POINT ( 'NONE',  ( 28.63125000122903074, 4.330127018922191873, 2.499999999999999556 ) ) ;
#48303=EDGE_CURVE ( 'NONE', #59817, #18738, #593, .T. ) ;
#48306=EDGE_CURVE ( 'NONE', #27766, #829, #18910, .T. ) ;
#48312=DIRECTION ( 'NONE',  ( 0.000000000000000000, 0.000000000000000000, 1.000000000000000000 ) ) ;
#48313=CARTESIAN_POINT ( 'NONE',  ( 29.47499999999999787, 4.330127018922191873, 2.499999999999999556 ) ) ;
#48315=CARTESIAN_POINT ( 'NONE',  ( 26.60625000122903216, -4.330127018922190985, -2.500000000000001332 ) ) ;
#48322=CARTESIAN_POINT ( 'NONE',  ( 9.131250001229034297, 6.123233995736764310E-16, -4.999999999999998224 ) ) ;
#48332=CARTESIAN_POINT ( 'NONE',  ( 15.60937500061451644, 2.746126346562645981, -4.756430356249997438 ) ) ;
#48336=CARTESIAN_POINT ( 'NONE',  ( 23.89687500061451431, 0.000000000000000000, 4.756430356249998326 ) ) ;
#48346=CARTESIAN_POINT ( 'NONE',  ( 14.21249999999999858, 2.886751345948126879, 4.999999999999999112 ) ) ;
#48353=CARTESIAN_POINT ( 'NONE',  ( 25.02187500061451431, -5.492252693125287522, -1.008910452111647106E-15 ) ) ;
#48357=CYLINDRICAL_SURFACE ( 'NONE', #68029, 4.999999999999998224 ) ;
#48373=CARTESIAN_POINT ( 'NONE',  ( 11.37187500061451928, 2.746126346562643317, 4.756430356249998326 ) ) ;
#48387=ORIENTED_EDGE ( 'NONE', *, *, #3037, .F. ) ;
#48400=ORIENTED_EDGE ( 'NONE', *, *, #45339, .F. ) ;
#48403=CARTESIAN_POINT ( 'NONE',  ( 12.98437500061451821, 5.824947211148865298E-16, -4.756430356249998326 ) ) ;
#48412=CARTESIAN_POINT ( 'NONE',  ( 14.40000000000000036, -4.330127018922190985, -2.500000000000001332 ) ) ;
#48422=EDGE_CURVE ( 'NONE', #43273, #69475, #68462, .T. ) ;
#48424=CARTESIAN_POINT ( 'NONE',  ( 22.77187500061451431, 5.824947211148865298E-16, -4.756430356249998326 ) ) ;
#48426=CARTESIAN_POINT ( 'NONE',  ( 9.084375000614516082, -2.746126346562646425, 4.756430356249996549 ) ) ;
#48430=CARTESIAN_POINT ( 'NONE',  ( 10.03125000122903288, 6.123233995736764310E-16, -4.999999999999998224 ) ) ;
#48437=CARTESIAN_POINT ( 'NONE',  ( 10.54687500061451644, -4.119189519843965641, -2.378215178125001383 ) ) ;
#48441=( BOUNDED_CURVE ( )  B_SPLINE_CURVE ( 2, ( #20060, #69958, #42616, #8630, #9367, #53701, #20431 ),
 .UNSPECIFIED., .F., .F. ) 
 B_SPLINE_CURVE_WITH_KNOTS ( ( 3, 2, 2, 3 ),
 ( 0.4300000000000001044, 0.4333333333333334036, 0.4366666666666667029, 0.4400000000000000022 ),
 .UNSPECIFIED. ) 
 CURVE ( )  GEOMETRIC_REPRESENTATION_ITEM ( )  RATIONAL_B_SPLINE_CURVE ( ( 0.9999999999999955591, 0.8660254037844431485, 1.000000000000000000, 0.8660254037844387076, 1.000000000000000000, 0.8660254037844387076, 1.000000000000000000 ) ) 
 REPRESENTATION_ITEM ( '' )  );
#48460=CARTESIAN_POINT ( 'NONE',  ( 18.79687500061451644, -2.746126346562641984, -4.756430356249999214 ) ) ;
#48464=VERTEX_POINT ( 'NONE', #64358 ) ;
#48473=LINE ( 'NONE', #70997, #53373 ) ;
#48478=CARTESIAN_POINT ( 'NONE',  ( 20.53125000122903288, 4.330127018922191873, 2.499999999999999556 ) ) ;
#48491=CARTESIAN_POINT ( 'NONE',  ( 20.03437500061451715, -4.119189519843968306, 2.378215178124996054 ) ) ;
#48497=CARTESIAN_POINT ( 'NONE',  ( 21.30000000000000071, 4.330127018922192761, -2.499999999999997780 ) ) ;
#48502=CARTESIAN_POINT ( 'NONE',  ( 11.94375000122903430, 5.773502691896255534, 3.535250795749688401E-16 ) ) ;
#48503=CARTESIAN_POINT ( 'NONE',  ( 18.58125000122903003, 6.123233995736764310E-16, -4.999999999999998224 ) ) ;
#48505=CARTESIAN_POINT ( 'NONE',  ( 18.24375000122903501, 5.773502691896255534, 3.535250795749688401E-16 ) ) ;
#48508=CARTESIAN_POINT ( 'NONE',  ( 7.143750001229034474, -2.886751345948129988, 4.999999999999997335 ) ) ;
#48510=CARTESIAN_POINT ( 'NONE',  ( 15.75937500061451502, 2.746126346562643317, 4.756430356249998326 ) ) ;
#48513=ORIENTED_EDGE ( 'NONE', *, *, #34066, .F. ) ;
#48516=CYLINDRICAL_SURFACE ( 'NONE', #43155, 4.999999999999998224 ) ;
#48520=CARTESIAN_POINT ( 'NONE',  ( 7.584375000614516971, 5.492252693125287522, 3.363034840372157021E-16 ) ) ;
#48531=CARTESIAN_POINT ( 'NONE',  ( 29.67187500061451644, 4.119189519843966529, 2.378215178124999607 ) ) ;
#48535=CARTESIAN_POINT ( 'NONE',  ( 9.187500000000001776, 5.773502691896255534, 3.535250795749688894E-16 ) ) ;
#48542=CARTESIAN_POINT ( 'NONE',  ( 27.19687500061451857, -2.746126346562646425, 4.756430356249996549 ) ) ;
#48544=CARTESIAN_POINT ( 'NONE',  ( 10.02187500061451964, 2.746126346562643317, 4.756430356249998326 ) ) ;
#48561=CARTESIAN_POINT ( 'NONE',  ( 21.84375000122903288, 5.773502691896255534, 3.535250795749688894E-16 ) ) ;
#48570=ADVANCED_FACE ( 'NONE', ( #34469 ), #52192, .T. ) ;
#48575=EDGE_CURVE ( 'NONE', #28191, #22800, #6177, .T. ) ;
#48577=CARTESIAN_POINT ( 'NONE',  ( 29.18437500061451573, 5.824947211148865298E-16, -4.756430356249998326 ) ) ;
#48611=CARTESIAN_POINT ( 'NONE',  ( 0.000000000000000000, 0.000000000000000000, 50.00000000000000000 ) ) ;
#48614=CARTESIAN_POINT ( 'NONE',  ( 14.63437500061451502, -2.746126346562642428, -4.756430356249999214 ) ) ;
#48621=DIRECTION ( 'NONE',  ( 0.000000000000000000, 0.000000000000000000, 1.000000000000000000 ) ) ;
#48628=CARTESIAN_POINT ( 'NONE',  ( 9.581250001229033586, 6.123233995736764310E-16, -4.999999999999998224 ) ) ;
#48632=DIRECTION ( 'NONE',  ( -1.000000000000000000, -0.000000000000000000, -0.000000000000000000 ) ) ;
#48633=CARTESIAN_POINT ( 'NONE',  ( 16.92187500061451999, -5.492252693125287522, -1.008910452111647106E-15 ) ) ;
#48644=CYLINDRICAL_SURFACE ( 'NONE', #72573, 4.999999999999998224 ) ;
#48647=CARTESIAN_POINT ( 'NONE',  ( 21.61875000122903145, -5.773502691896255534, -1.060575238724906372E-15 ) ) ;
#48651=CARTESIAN_POINT ( 'NONE',  ( 28.14375000122903359, 5.773502691896255534, 3.535250795749688894E-16 ) ) ;
#48653=CARTESIAN_POINT ( 'NONE',  ( 26.71875000122903288, 2.886751345948115333, -5.000000000000023093 ) ) ;
#48670=EDGE_CURVE ( 'NONE', #35381, #1580, #8546, .T. ) ;
#48677=CARTESIAN_POINT ( 'NONE',  ( 29.77499999999999858, 6.123233995736764310E-16, -4.999999999999998224 ) ) ;
#48685=( BOUNDED_CURVE ( )  B_SPLINE_CURVE ( 2, ( #59194, #59935, #53674, #48869, #70659, #42589, #37039 ),
 .UNSPECIFIED., .F., .F. ) 
 B_SPLINE_CURVE_WITH_KNOTS ( ( 3, 2, 2, 3 ),
 ( 0.4400000000000000022, 0.4433333333333333570, 0.4466666666666666563, 0.4500000000000000111 ),
 .UNSPECIFIED. ) 
 CURVE ( )  GEOMETRIC_REPRESENTATION_ITEM ( )  RATIONAL_B_SPLINE_CURVE ( ( 1.000000000000000000, 0.8660254037844387076, 1.000000000000000000, 0.8660254037844387076, 1.000000000000000000, 0.8660254037844387076, 1.000000000000000000 ) ) 
 REPRESENTATION_ITEM ( '' )  );
#48696=CARTESIAN_POINT ( 'NONE',  ( 12.87187500061451750, 5.824947211148865298E-16, -4.756430356249998326 ) ) ;
#48700=CARTESIAN_POINT ( 'NONE',  ( 24.64687500061451431, 4.119189519843966529, -2.378215178124998275 ) ) ;
#48711=CARTESIAN_POINT ( 'NONE',  ( 12.52500000000000213, -4.330127018922194537, 2.499999999999995559 ) ) ;
#48718=CARTESIAN_POINT ( 'NONE',  ( 24.34687500061451715, 5.492252693125287522, 3.363034840372157021E-16 ) ) ;
#48738=CARTESIAN_POINT ( 'NONE',  ( 9.759375000614516793, -4.119189519843965641, -2.378215178125001383 ) ) ;
#48751=ORIENTED_EDGE ( 'NONE', *, *, #66440, .F. ) ;
#48767=CARTESIAN_POINT ( 'NONE',  ( 14.70937500061451786, -4.119189519843965641, -2.378215178125001383 ) ) ;
#48775=CARTESIAN_POINT ( 'NONE',  ( 15.11249999999999893, 2.886751345948126879, 4.999999999999999112 ) ) ;
#48778=FACE_OUTER_BOUND ( 'NONE', #66920, .T. ) ;
#48787=CARTESIAN_POINT ( 'NONE',  ( 22.13437500061451502, -2.746126346562646425, 4.756430356249996549 ) ) ;
#48800=CARTESIAN_POINT ( 'NONE',  ( 9.984375000614516438, -2.746126346562646425, 4.756430356249996549 ) ) ;
#48810=ORIENTED_EDGE ( 'NONE', *, *, #59386, .T. ) ;
#48822=CARTESIAN_POINT ( 'NONE',  ( 16.80937500061451573, 0.000000000000000000, 4.756430356249998326 ) ) ;
#48826=( BOUNDED_CURVE ( )  B_SPLINE_CURVE ( 2, ( #51097, #67376, #44111, #16739, #61808, #17101, #49650 ),
 .UNSPECIFIED., .F., .F. ) 
 B_SPLINE_CURVE_WITH_KNOTS ( ( 3, 2, 2, 3 ),
 ( 0.4400000000000000022, 0.4433333333333333570, 0.4466666666666666563, 0.4500000000000000111 ),
 .UNSPECIFIED. ) 
 CURVE ( )  GEOMETRIC_REPRESENTATION_ITEM ( )  RATIONAL_B_SPLINE_CURVE ( ( 1.000000000000000000, 0.8660254037844387076, 1.000000000000000000, 0.8660254037844387076, 1.000000000000000000, 0.8660254037844387076, 1.000000000000000000 ) ) 
 REPRESENTATION_ITEM ( '' )  );
#48856=CARTESIAN_POINT ( 'NONE',  ( 21.72187500061451715, 2.746126346562643317, 4.756430356249998326 ) ) ;
#48862=CARTESIAN_POINT ( 'NONE',  ( 23.06250000000000355, 2.886751345948129099, -4.999999999999998224 ) ) ;
#48866=DIRECTION ( 'NONE',  ( -1.000000000000000000, -0.000000000000000000, -0.000000000000000000 ) ) ;
#48869=CARTESIAN_POINT ( 'NONE',  ( 19.59375000122902932, 5.773502691896255534, 3.535250795749688401E-16 ) ) ;
#48874=CARTESIAN_POINT ( 'NONE',  ( 29.22187500061451360, 4.119189519843966529, 2.378215178124999607 ) ) ;
#48876=CARTESIAN_POINT ( 'NONE',  ( 12.42187500061451466, 5.824947211148865298E-16, -4.756430356249998326 ) ) ;
#48879=ORIENTED_EDGE ( 'NONE', *, *, #51676, .F. ) ;
#48882=DIRECTION ( 'NONE',  ( 0.000000000000000000, 0.000000000000000000, 1.000000000000000000 ) ) ;
#48886=CARTESIAN_POINT ( 'NONE',  ( 9.084375000614516082, -2.746126346562646425, 4.756430356249996549 ) ) ;
#48909=CARTESIAN_POINT ( 'NONE',  ( 26.52187500061451431, 2.746126346562645981, -4.756430356249997438 ) ) ;
#48911=DIRECTION ( 'NONE',  ( -1.000000000000000000, -0.000000000000000000, -0.000000000000000000 ) ) ;
#48931=CARTESIAN_POINT ( 'NONE',  ( 18.61875000122903145, 2.886751345948129099, -4.999999999999998224 ) ) ;
#48942=EDGE_CURVE ( 'NONE', #55986, #38622, #4148, .T. ) ;
#48947=CARTESIAN_POINT ( 'NONE',  ( 28.13437500061451502, -4.119189519843968306, 2.378215178124996054 ) ) ;
#48956=AXIS2_PLACEMENT_3D ( 'NONE', #65877, #32627, #49262 ) ;
#48981=CARTESIAN_POINT ( 'NONE',  ( 19.04999999999999716, 4.330127018922192761, -2.499999999999997780 ) ) ;
#48984=CARTESIAN_POINT ( 'NONE',  ( 14.37187500061451573, 4.119189519843966529, 2.378215178124999607 ) ) ;
#48995=CARTESIAN_POINT ( 'NONE',  ( 16.78125000122903288, 6.123233995736764310E-16, -4.999999999999998224 ) ) ;
#48998=CARTESIAN_POINT ( 'NONE',  ( 14.17500000000000071, 4.330127018922191873, 2.499999999999999556 ) ) ;
#49001=CARTESIAN_POINT ( 'NONE',  ( 0.000000000000000000, 0.000000000000000000, 50.00000000000000000 ) ) ;
#49002=CARTESIAN_POINT ( 'NONE',  ( 14.78437500061451715, 5.824947211148865298E-16, -4.756430356249998326 ) ) ;
#49021=CARTESIAN_POINT ( 'NONE',  ( 27.88125000122903074, -4.330127018922194537, 2.499999999999995559 ) ) ;
#49042=( BOUNDED_CURVE ( )  B_SPLINE_CURVE ( 2, ( #50018, #32287, #54821, #72542, #45567, #39297, #67730 ),
 .UNSPECIFIED., .F., .F. ) 
 B_SPLINE_CURVE_WITH_KNOTS ( ( 3, 2, 2, 3 ),
 ( 0.5400000000000001465, 0.5433333333333333348, 0.5466666666666666341, 0.5499999999999999334 ),
 .UNSPECIFIED. ) 
 CURVE ( )  GEOMETRIC_REPRESENTATION_ITEM ( )  RATIONAL_B_SPLINE_CURVE ( ( 0.9999999999999955591, 0.8660254037844431485, 1.000000000000000000, 0.8660254037844387076, 1.000000000000000000, 0.8660254037844431485, 0.9999999999999955591 ) ) 
 REPRESENTATION_ITEM ( '' )  );
#49048=CARTESIAN_POINT ( 'NONE',  ( 27.52500000000000213, 6.123233995736764310E-16, -4.999999999999998224 ) ) ;
#49066=EDGE_CURVE ( 'NONE', #37967, #18378, #66557, .T. ) ;
#49070=CARTESIAN_POINT ( 'NONE',  ( 20.82187500061451502, -4.119189519843968306, 2.378215178124996054 ) ) ;
#49074=CARTESIAN_POINT ( 'NONE',  ( 15.91875000122902684, 2.886751345948018077, -5.000000000000190070 ) ) ;
#49079=CARTESIAN_POINT ( 'NONE',  ( 23.40000000000000213, -4.330127018922190985, -2.500000000000001332 ) ) ;
#49080=ORIENTED_EDGE ( 'NONE', *, *, #1611, .T. ) ;
#49081=CARTESIAN_POINT ( 'NONE',  ( 14.06250000000000000, 2.886751345948129099, -4.999999999999998224 ) ) ;
#49089=CARTESIAN_POINT ( 'NONE',  ( 22.99687500061451573, 5.492252693125287522, 3.363034840372157021E-16 ) ) ;
#49098=LINE ( 'NONE', #49825, #50165 ) ;
#49110=CARTESIAN_POINT ( 'NONE',  ( 10.54687500061451644, -2.746126346562646425, 4.756430356249996549 ) ) ;
#49114=( BOUNDED_CURVE ( )  B_SPLINE_CURVE ( 2, ( #2441, #24964, #70038, #41971, #13884, #70409, #19785 ),
 .UNSPECIFIED., .F., .F. ) 
 B_SPLINE_CURVE_WITH_KNOTS ( ( 3, 2, 2, 3 ),
 ( 0.1799999999999999378, 0.1833333333333333204, 0.1866666666666667029, 0.1900000000000000855 ),
 .UNSPECIFIED. ) 
 CURVE ( )  GEOMETRIC_REPRESENTATION_ITEM ( )  RATIONAL_B_SPLINE_CURVE ( ( 1.000000000000002220, 0.8660254037844364872, 1.000000000000000000, 0.8660254037844387076, 1.000000000000000000, 0.8660254037844353769, 1.000000000000003331 ) ) 
 REPRESENTATION_ITEM ( '' )  );
#49136=CARTESIAN_POINT ( 'NONE',  ( 11.74687500061451573, 5.492252693125287522, 3.363034840372157021E-16 ) ) ;
#49137=CARTESIAN_POINT ( 'NONE',  ( 20.15625000122903288, 0.000000000000000000, 4.999999999999998224 ) ) ;
#49145=CARTESIAN_POINT ( 'NONE',  ( 16.80000000000000071, 4.330127018922192761, -2.499999999999997780 ) ) ;
#49156=CARTESIAN_POINT ( 'NONE',  ( 21.23437500061451644, -2.746126346562646425, 4.756430356249996549 ) ) ;
#49159=CARTESIAN_POINT ( 'NONE',  ( 14.15625000122903288, 4.330127018922192761, -2.499999999999997780 ) ) ;
#49173=CARTESIAN_POINT ( 'NONE',  ( 10.47187500061451715, -4.119189519843968306, 2.378215178124996054 ) ) ;
#49183=EDGE_LOOP ( 'NONE', ( #25993, #33169, #67787, #23791 ) ) ;
#49194=CARTESIAN_POINT ( 'NONE',  ( 17.97187500061451715, 2.746126346562645981, -4.756430356249997438 ) ) ;
#49206=EDGE_LOOP ( 'NONE', ( #16193, #54355, #1203, #10056 ) ) ;
#49225=CARTESIAN_POINT ( 'NONE',  ( 17.63437500061451502, 4.119189519843966529, 2.378215178124999607 ) ) ;
#49232=CARTESIAN_POINT ( 'NONE',  ( 22.91249999999999432, -5.773502691896255534, -1.060575238724906372E-15 ) ) ;
#49237=CARTESIAN_POINT ( 'NONE',  ( 28.31249999999999645, -5.773502691896255534, -1.060575238724906372E-15 ) ) ;
#49242=CARTESIAN_POINT ( 'NONE',  ( 27.79687500061451289, 4.119189519843966529, -2.378215178124998275 ) ) ;
#49244=CARTESIAN_POINT ( 'NONE',  ( 13.88437500061451679, 5.492252693125287522, 3.363034840372157021E-16 ) ) ;
#49252=VECTOR ( 'NONE', #50558, 1000.000000000000000 ) ;
#49255=CARTESIAN_POINT ( 'NONE',  ( 9.271875000614517859, 5.824947211148865298E-16, -4.756430356249998326 ) ) ;
#49257=EDGE_CURVE ( 'NONE', #61968, #72906, #10510, .T. ) ;
#49262=DIRECTION ( 'NONE',  ( 0.000000000000000000, 0.000000000000000000, 1.000000000000000000 ) ) ;
#49268=ORIENTED_EDGE ( 'NONE', *, *, #26320, .T. ) ;
#49277=CARTESIAN_POINT ( 'NONE',  ( 23.18437500061451573, -4.119189519843968306, 2.378215178124996054 ) ) ;
#49279=CARTESIAN_POINT ( 'NONE',  ( 8.109375000614518214, 4.119189519843966529, -2.378215178124998275 ) ) ;
#49296=CARTESIAN_POINT ( 'NONE',  ( 18.05625000122903501, -4.330127018922190985, -2.500000000000001332 ) ) ;
#49311=CARTESIAN_POINT ( 'NONE',  ( 29.48437500061451644, -4.119189519843968306, 2.378215178124996054 ) ) ;
#49318=( BOUNDED_CURVE ( )  B_SPLINE_CURVE ( 2, ( #3443, #25962, #20406, #48502, #31132, #14504, #41853 ),
 .UNSPECIFIED., .F., .F. ) 
 B_SPLINE_CURVE_WITH_KNOTS ( ( 3, 2, 2, 3 ),
 ( 0.7800000000000001377, 0.7833333333333334370, 0.7866666666666667362, 0.7900000000000001465 ),
 .UNSPECIFIED. ) 
 CURVE ( )  GEOMETRIC_REPRESENTATION_ITEM ( )  RATIONAL_B_SPLINE_CURVE ( ( 0.9999999999999955591, 0.8660254037844431485, 1.000000000000000000, 0.8660254037844387076, 1.000000000000000000, 0.8660254037844342667, 1.000000000000004441 ) ) 
 REPRESENTATION_ITEM ( '' )  );
#49321=CARTESIAN_POINT ( 'NONE',  ( 25.05000000000000071, 0.000000000000000000, 4.999999999999998224 ) ) ;
#49325=CARTESIAN_POINT ( 'NONE',  ( 8.625000000000000000, 6.123233995736764310E-16, -4.999999999999998224 ) ) ;
#49331=CARTESIAN_POINT ( 'NONE',  ( 20.44687500061451502, -4.119189519843965641, -2.378215178125001383 ) ) ;
#49334=ORIENTED_EDGE ( 'NONE', *, *, #24198, .F. ) ;
#49342=ORIENTED_EDGE ( 'NONE', *, *, #29976, .T. ) ;
#49346=ORIENTED_EDGE ( 'NONE', *, *, #61190, .T. ) ;
#49350=CARTESIAN_POINT ( 'NONE',  ( 14.93437500061451573, -2.746126346562646425, 4.756430356249996549 ) ) ;
#49358=ORIENTED_EDGE ( 'NONE', *, *, #16519, .T. ) ;
#49365=CARTESIAN_POINT ( 'NONE',  ( 16.98750000000000426, -2.886751345948074920, 5.000000000000092371 ) ) ;
#49369=CARTESIAN_POINT ( 'NONE',  ( 15.27187500061451786, 2.746126346562645981, -4.756430356249997438 ) ) ;
#49379=CARTESIAN_POINT ( 'NONE',  ( 12.44999999999999929, 0.000000000000000000, 4.999999999999998224 ) ) ;
#49385=CARTESIAN_POINT ( 'NONE',  ( 24.88125000122903074, 6.123233995736764310E-16, -4.999999999999998224 ) ) ;
#49387=CARTESIAN_POINT ( 'NONE',  ( 26.75625000122903430, 4.330127018922192761, -2.499999999999997780 ) ) ;
#49397=CARTESIAN_POINT ( 'NONE',  ( 13.63125000122903252, 6.123233995736764310E-16, -4.999999999999998224 ) ) ;
#49416=CARTESIAN_POINT ( 'NONE',  ( 22.42500000000000071, -4.330127018922194537, 2.499999999999995559 ) ) ;
#49427=EDGE_CURVE ( 'NONE', #63177, #31702, #36387, .T. ) ;
#49431=CARTESIAN_POINT ( 'NONE',  ( 21.42187500061451644, 5.824947211148865298E-16, -4.756430356249998326 ) ) ;
#49439=ORIENTED_EDGE ( 'NONE', *, *, #64274, .F. ) ;
#49440=CARTESIAN_POINT ( 'NONE',  ( 12.41249999999999964, 2.886751345948126879, 4.999999999999999112 ) ) ;
#49447=CARTESIAN_POINT ( 'NONE',  ( 23.55937500061451573, 0.000000000000000000, 4.756430356249998326 ) ) ;
#49469=CARTESIAN_POINT ( 'NONE',  ( 10.35937500061451644, 4.119189519843966529, -2.378215178124998275 ) ) ;
#49490=ORIENTED_EDGE ( 'NONE', *, *, #71191, .T. ) ;
#49491=ADVANCED_FACE ( 'NONE', ( #42044 ), #7689, .T. ) ;
#49495=CARTESIAN_POINT ( 'NONE',  ( 10.92187500061451644, 2.746126346562643317, 4.756430356249998326 ) ) ;
#49500=EDGE_CURVE ( 'NONE', #39358, #72520, #59016, .T. ) ;
#49511=( BOUNDED_CURVE ( )  B_SPLINE_CURVE ( 2, ( #45414, #67592, #29507, #6249, #5530, #28067, #39511 ),
 .UNSPECIFIED., .F., .F. ) 
 B_SPLINE_CURVE_WITH_KNOTS ( ( 3, 2, 2, 3 ),
 ( 0.7500000000000000000, 0.7533333333333332993, 0.7566666666666667096, 0.7600000000000000089 ),
 .UNSPECIFIED. ) 
 CURVE ( )  GEOMETRIC_REPRESENTATION_ITEM ( )  RATIONAL_B_SPLINE_CURVE ( ( 1.000000000000000000, 0.8660254037844387076, 1.000000000000000000, 0.8660254037844387076, 1.000000000000000000, 0.8660254037844387076, 1.000000000000000000 ) ) 
 REPRESENTATION_ITEM ( '' )  );
#49515=( BOUNDED_CURVE ( )  B_SPLINE_CURVE ( 2, ( #50434, #44893, #62589, #34508, #57036, #18222, #23423 ),
 .UNSPECIFIED., .F., .F. ) 
 B_SPLINE_CURVE_WITH_KNOTS ( ( 3, 2, 2, 3 ),
 ( 0.4200000000000000955, 0.4233333333333334503, 0.4266666666666668051, 0.4300000000000001044 ),
 .UNSPECIFIED. ) 
 CURVE ( )  GEOMETRIC_REPRESENTATION_ITEM ( )  RATIONAL_B_SPLINE_CURVE ( ( 0.9999999999999955591, 0.8660254037844431485, 1.000000000000000000, 0.8660254037844387076, 1.000000000000000000, 0.8660254037844342667, 1.000000000000004441 ) ) 
 REPRESENTATION_ITEM ( '' )  );
#49517=CARTESIAN_POINT ( 'NONE',  ( 20.52187500061451786, 5.824947211148865298E-16, -4.756430356249998326 ) ) ;
#49520=CARTESIAN_POINT ( 'NONE',  ( 15.31875000122903252, -5.773502691896255534, -1.060575238724906372E-15 ) ) ;
#49522=CARTESIAN_POINT ( 'NONE',  ( 7.359375000614516438, -5.492252693125287522, -1.008910452111647106E-15 ) ) ;
#49534=CARTESIAN_POINT ( 'NONE',  ( 28.54687500061451644, -2.746126346562646425, 4.756430356249996549 ) ) ;
#49545=ORIENTED_EDGE ( 'NONE', *, *, #11547, .F. ) ;
#49557=CARTESIAN_POINT ( 'NONE',  ( 16.69687500061451502, 5.492252693125287522, 3.363034840372157021E-16 ) ) ;
#49561=ORIENTED_EDGE ( 'NONE', *, *, #54635, .T. ) ;
#49587=CARTESIAN_POINT ( 'NONE',  ( 18.42187500061451644, 2.746126346562645981, -4.756430356249997438 ) ) ;
#49594=CARTESIAN_POINT ( 'NONE',  ( 20.96250000000000213, 2.886751345948126879, 4.999999999999999112 ) ) ;
#49596=CARTESIAN_POINT ( 'NONE',  ( 20.66250000000000142, -5.773502691896255534, -1.060575238724906372E-15 ) ) ;
#49597=CARTESIAN_POINT ( 'NONE',  ( 24.20625000122903359, 0.000000000000000000, 4.999999999999998224 ) ) ;
#49604=CARTESIAN_POINT ( 'NONE',  ( 27.08437500061451431, -2.746126346562646425, 4.756430356249996549 ) ) ;
#49606=CARTESIAN_POINT ( 'NONE',  ( 14.18437500061451573, -2.746126346562641984, -4.756430356249999214 ) ) ;
#49618=EDGE_LOOP ( 'NONE', ( #69966, #20839, #123, #33011 ) ) ;
#49633=CARTESIAN_POINT ( 'NONE',  ( 25.55625000122903501, 0.000000000000000000, 4.999999999999998224 ) ) ;
#49641=CARTESIAN_POINT ( 'NONE',  ( 24.12187500061451573, -5.492252693125287522, -1.008910452111647106E-15 ) ) ;
#49643=CARTESIAN_POINT ( 'NONE',  ( 8.484375000614518214, 5.824947211148865298E-16, -4.756430356249998326 ) ) ;
#49650=CARTESIAN_POINT ( 'NONE',  ( 19.87500000000000000, 6.123233995736764310E-16, -4.999999999999998224 ) ) ;
#49661=CARTESIAN_POINT ( 'NONE',  ( 18.58125000122903003, 6.123233995736764310E-16, -4.999999999999998224 ) ) ;
#49678=CARTESIAN_POINT ( 'NONE',  ( 25.54687500061451644, -2.746126346562642428, -4.756430356249999214 ) ) ;
#49693=CARTESIAN_POINT ( 'NONE',  ( 10.74375000122903323, -2.886751345948129988, 4.999999999999997335 ) ) ;
#49695=CARTESIAN_POINT ( 'NONE',  ( 14.00625000122903252, -4.330127018922190985, -2.500000000000001332 ) ) ;
#49697=CARTESIAN_POINT ( 'NONE',  ( 20.03437500061451715, -2.746126346562641984, -4.756430356249999214 ) ) ;
#49701=CYLINDRICAL_SURFACE ( 'NONE', #35978, 4.999999999999998224 ) ;
#49715=CARTESIAN_POINT ( 'NONE',  ( 13.09687500061451715, 0.000000000000000000, 4.756430356249998326 ) ) ;
#49721=ORIENTED_EDGE ( 'NONE', *, *, #8883, .F. ) ;
#49732=CARTESIAN_POINT ( 'NONE',  ( 29.03437500061451360, -2.746126346562641984, -4.756430356249999214 ) ) ;
#49733=CARTESIAN_POINT ( 'NONE',  ( 15.57187500061451679, -5.492252693125287522, -1.008910452111647106E-15 ) ) ;
#49743=CARTESIAN_POINT ( 'NONE',  ( 13.04999999999999893, -4.330127018922190985, -2.500000000000001332 ) ) ;
#49746=CARTESIAN_POINT ( 'NONE',  ( 25.53750000000000142, -2.886751345948116221, 5.000000000000021316 ) ) ;
#49750=CARTESIAN_POINT ( 'NONE',  ( 25.93125000122903145, 4.330127018922191873, 2.499999999999999556 ) ) ;
#49755=COLOUR_RGB ( '',0.8941176470588234615, 0.8941176470588234615, 0.8941176470588234615 ) ;
#49758=( BOUNDED_CURVE ( )  B_SPLINE_CURVE ( 2, ( #52005, #56804, #51644, #23915, #41289, #46101, #46463 ),
 .UNSPECIFIED., .F., .F. ) 
 B_SPLINE_CURVE_WITH_KNOTS ( ( 3, 2, 2, 3 ),
 ( 0.3800000000000000044, 0.3833333333333333592, 0.3866666666666666585, 0.3900000000000000133 ),
 .UNSPECIFIED. ) 
 CURVE ( )  GEOMETRIC_REPRESENTATION_ITEM ( )  RATIONAL_B_SPLINE_CURVE ( ( 1.000000000000000000, 0.8660254037844387076, 1.000000000000000000, 0.8660254037844387076, 1.000000000000000000, 0.8660254037844387076, 1.000000000000000000 ) ) 
 REPRESENTATION_ITEM ( '' )  );
#49767=CARTESIAN_POINT ( 'NONE',  ( 34.99999999999999289, -2.499999999999999556, 3.499999999999999556 ) ) ;
#49796=VECTOR ( 'NONE', #34114, 1000.000000000000000 ) ;
#49799=CARTESIAN_POINT ( 'NONE',  ( 21.27187500061451431, -4.119189519843968306, 2.378215178124996054 ) ) ;
#49807=VERTEX_POINT ( 'NONE', #3620 ) ;
#49808=CARTESIAN_POINT ( 'NONE',  ( 10.80000000000000071, -4.330127018922190985, -2.500000000000001332 ) ) ;
#49814=CARTESIAN_POINT ( 'NONE',  ( 34.99999999999999289, 6.123233995736764310E-16, -4.999999999999998224 ) ) ;
#49815=CARTESIAN_POINT ( 'NONE',  ( 21.45937500061451786, -4.119189519843965641, -2.378215178125001383 ) ) ;
#49825=CARTESIAN_POINT ( 'NONE',  ( 45.00000000000000000, 6.123233995736764310E-16, -4.999999999999998224 ) ) ;
#49832=CARTESIAN_POINT ( 'NONE',  ( 18.45000000000000284, -4.330127018922190985, -2.500000000000001332 ) ) ;
#49837=CARTESIAN_POINT ( 'NONE',  ( 10.73437500061451644, 5.824947211148865298E-16, -4.756430356249998326 ) ) ;
#49860=CARTESIAN_POINT ( 'NONE',  ( 12.30937500061451573, 0.000000000000000000, 4.756430356249998326 ) ) ;
#49861=CARTESIAN_POINT ( 'NONE',  ( 45.00000000000000000, 0.000000000000000000, 4.999999999999998224 ) ) ;
#49874=DIRECTION ( 'NONE',  ( -1.000000000000000000, -0.000000000000000000, -0.000000000000000000 ) ) ;
#49878=CARTESIAN_POINT ( 'NONE',  ( 18.90937500061451360, 2.746126346562643317, 4.756430356249998326 ) ) ;
#49881=CARTESIAN_POINT ( 'NONE',  ( 13.81875000122903074, 2.886751345948126879, 4.999999999999999112 ) ) ;
#49896=CARTESIAN_POINT ( 'NONE',  ( 7.771875000614516082, -4.119189519843968306, 2.378215178124996054 ) ) ;
#49899=( BOUNDED_CURVE ( )  B_SPLINE_CURVE ( 2, ( #70106, #40959, #46491, #57919, #64193, #58645, #18391 ),
 .UNSPECIFIED., .F., .F. ) 
 B_SPLINE_CURVE_WITH_KNOTS ( ( 3, 2, 2, 3 ),
 ( 0.4099999999999999201, 0.4133333333333333304, 0.4166666666666667407, 0.4200000000000000955 ),
 .UNSPECIFIED. ) 
 CURVE ( )  GEOMETRIC_REPRESENTATION_ITEM ( )  RATIONAL_B_SPLINE_CURVE ( ( 1.000000000000002220, 0.8660254037844364872, 1.000000000000000000, 0.8660254037844387076, 1.000000000000000000, 0.8660254037844342667, 1.000000000000004441 ) ) 
 REPRESENTATION_ITEM ( '' )  );
#49918=CARTESIAN_POINT ( 'NONE',  ( 16.50937500061451502, -4.119189519843965641, -2.378215178125001383 ) ) ;
#49932=EDGE_LOOP ( 'NONE', ( #63975, #26392, #28395, #139 ) ) ;
#49936=EDGE_CURVE ( 'NONE', #1846, #64001, #16108, .T. ) ;
#49950=CARTESIAN_POINT ( 'NONE',  ( 19.28437500061451360, 5.824947211148865298E-16, -4.756430356249998326 ) ) ;
#49957=CARTESIAN_POINT ( 'NONE',  ( 19.83750000000000213, -2.886751345948125991, -5.000000000000000000 ) ) ;
#49959=CARTESIAN_POINT ( 'NONE',  ( 21.60000000000000142, -4.330127018922190985, -2.500000000000001332 ) ) ;
#49960=CARTESIAN_POINT ( 'NONE',  ( 25.77187500061451431, -4.119189519843968306, 2.378215178124996054 ) ) ;
#49961=CARTESIAN_POINT ( 'NONE',  ( 14.41875000122903394, -5.773502691896255534, -1.060575238724906372E-15 ) ) ;
#49968=CARTESIAN_POINT ( 'NONE',  ( 27.27187500061451786, 5.824947211148865298E-16, -4.756430356249998326 ) ) ;
#49970=CARTESIAN_POINT ( 'NONE',  ( 14.52187500061451608, -4.119189519843968306, 2.378215178124996054 ) ) ;
#49976=CARTESIAN_POINT ( 'NONE',  ( 17.19375000122903430, -2.886751345948070480, -5.000000000000095923 ) ) ;
#50005=CARTESIAN_POINT ( 'NONE',  ( 24.23437500061451644, 5.824947211148865298E-16, -4.756430356249998326 ) ) ;
#50007=CARTESIAN_POINT ( 'NONE',  ( 7.546875000614517326, -2.746126346562642428, -4.756430356249999214 ) ) ;
#50018=CARTESIAN_POINT ( 'NONE',  ( 17.45625000122903003, 0.000000000000000000, 4.999999999999998224 ) ) ;
#50025=CARTESIAN_POINT ( 'NONE',  ( 18.99375000122903501, -2.886751345948125991, -5.000000000000000000 ) ) ;
#50040=CARTESIAN_POINT ( 'NONE',  ( 26.52187500061451431, 2.746126346562645981, -4.756430356249997438 ) ) ;
#50054=CARTESIAN_POINT ( 'NONE',  ( 11.79375000122903394, -2.886751345948125991, -5.000000000000000000 ) ) ;
#50055=CARTESIAN_POINT ( 'NONE',  ( 9.581250001229033586, 6.123233995736764310E-16, -4.999999999999998224 ) ) ;
#50057=CARTESIAN_POINT ( 'NONE',  ( 20.93437500061450862, -2.746126346562641984, -4.756430356249999214 ) ) ;
#50058=AXIS2_PLACEMENT_3D ( 'NONE', #11423, #33940, #56483 ) ;
#50061=ORIENTED_EDGE ( 'NONE', *, *, #19119, .T. ) ;
#50064=FACE_OUTER_BOUND ( 'NONE', #5224, .T. ) ;
#50069=CARTESIAN_POINT ( 'NONE',  ( 12.98437500061451289, 5.492252693125287522, 3.363034840372157021E-16 ) ) ;
#50078=CARTESIAN_POINT ( 'NONE',  ( 13.88437500061451502, 5.492252693125287522, 3.363034840372157021E-16 ) ) ;
#50094=CARTESIAN_POINT ( 'NONE',  ( 22.59375000122903288, -2.886751345948126435, -5.000000000000000000 ) ) ;
#50095=CARTESIAN_POINT ( 'NONE',  ( 15.08437500061451786, -4.119189519843968306, 2.378215178124996054 ) ) ;
#50096=FACE_OUTER_BOUND ( 'NONE', #49183, .T. ) ;
#50099=EDGE_CURVE ( 'NONE', #48021, #41736, #3385, .T. ) ;
#50104=CARTESIAN_POINT ( 'NONE',  ( 8.175000000000002487, 6.123233995736764310E-16, -4.999999999999998224 ) ) ;
#50114=CARTESIAN_POINT ( 'NONE',  ( 25.25625000122903074, -4.330127018922190985, -2.500000000000001332 ) ) ;
#50127=CARTESIAN_POINT ( 'NONE',  ( 13.70625000122903359, 4.330127018922192761, -2.499999999999997780 ) ) ;
#50154=CARTESIAN_POINT ( 'NONE',  ( 29.15625000122903288, 0.000000000000000000, 4.999999999999998224 ) ) ;
#50162=CARTESIAN_POINT ( 'NONE',  ( 21.45937500061451075, 2.746126346562645981, -4.756430356249997438 ) ) ;
#50165=VECTOR ( 'NONE', #67546, 1000.000000000000000 ) ;
#50172=CARTESIAN_POINT ( 'NONE',  ( 11.55000000000000071, 0.000000000000000000, 4.999999999999998224 ) ) ;
#50180=CARTESIAN_POINT ( 'NONE',  ( 22.77187500061451786, -5.492252693125287522, -1.008910452111647106E-15 ) ) ;
#50205=CARTESIAN_POINT ( 'NONE',  ( 9.159375000614515372, 0.000000000000000000, 4.756430356249998326 ) ) ;
#50227=CARTESIAN_POINT ( 'NONE',  ( 11.55937500061451928, -4.119189519843965641, -2.378215178125001383 ) ) ;
#50233=VECTOR ( 'NONE', #30767, 1000.000000000000000 ) ;
#50243=DIRECTION ( 'NONE',  ( 0.000000000000000000, 0.000000000000000000, 1.000000000000000000 ) ) ;
#50250=CARTESIAN_POINT ( 'NONE',  ( 20.25937500061451502, 2.746126346562643317, 4.756430356249998326 ) ) ;
#50253=CARTESIAN_POINT ( 'NONE',  ( 14.83125000122903359, -4.330127018922194537, 2.499999999999995559 ) ) ;
#50255=CARTESIAN_POINT ( 'NONE',  ( 7.471875000614514484, 5.824947211148865298E-16, -4.756430356249998326 ) ) ;
#50267=CARTESIAN_POINT ( 'NONE',  ( 29.29687500061451644, 5.492252693125287522, 3.363034840372157021E-16 ) ) ;
#50290=CARTESIAN_POINT ( 'NONE',  ( 17.82187500061451502, -5.492252693125287522, -1.008910452111647106E-15 ) ) ;
#50296=ORIENTED_EDGE ( 'NONE', *, *, #33344, .F. ) ;
#50323=CARTESIAN_POINT ( 'NONE',  ( 19.95937500061451786, 0.000000000000000000, 4.756430356249998326 ) ) ;
#50328=CARTESIAN_POINT ( 'NONE',  ( 19.27500000000000213, -4.330127018922194537, 2.499999999999995559 ) ) ;
#50331=CARTESIAN_POINT ( 'NONE',  ( 21.56250000000000000, -5.773502691896255534, -1.060575238724906372E-15 ) ) ;
#50332=CARTESIAN_POINT ( 'NONE',  ( 25.35937500061451644, -5.492252693125287522, -1.008910452111647106E-15 ) ) ;
#50335=CARTESIAN_POINT ( 'NONE',  ( 45.00000000000000000, 6.123233995736764310E-16, -4.999999999999998224 ) ) ;
#50339=CARTESIAN_POINT ( 'NONE',  ( 28.17187500061451289, 5.824947211148865298E-16, -4.756430356249998326 ) ) ;
#50341=CARTESIAN_POINT ( 'NONE',  ( 14.63437500061451502, -2.746126346562641984, -4.756430356249999214 ) ) ;
#50344=VERTEX_POINT ( 'NONE', #63294 ) ;
#50374=CARTESIAN_POINT ( 'NONE',  ( 24.27187500061451786, 2.746126346562645981, -4.756430356249997438 ) ) ;
#50385=CARTESIAN_POINT ( 'NONE',  ( 7.706250001229031810, -4.330127018922190985, -2.500000000000001332 ) ) ;
#50392=CARTESIAN_POINT ( 'NONE',  ( 18.73125000122903216, 4.330127018922191873, 2.499999999999999556 ) ) ;
#50394=CARTESIAN_POINT ( 'NONE',  ( 29.53125000122903288, 4.330127018922191873, 2.499999999999999556 ) ) ;
#50395=ORIENTED_EDGE ( 'NONE', *, *, #5393, .F. ) ;
#50404=( BOUNDED_CURVE ( )  B_SPLINE_CURVE ( 2, ( #1104, #41344, #7716, #63854, #23611, #6640, #52782 ),
 .UNSPECIFIED., .F., .F. ) 
 B_SPLINE_CURVE_WITH_KNOTS ( ( 3, 2, 2, 3 ),
 ( 0.06000000000000003941, 0.06333333333333336645, 0.06666666666666667962, 0.07000000000000000666 ),
 .UNSPECIFIED. ) 
 CURVE ( )  GEOMETRIC_REPRESENTATION_ITEM ( )  RATIONAL_B_SPLINE_CURVE ( ( 0.9999999999999983347, 0.8660254037844403729, 1.000000000000000000, 0.8660254037844387076, 1.000000000000000000, 0.8660254037844387076, 1.000000000000000000 ) ) 
 REPRESENTATION_ITEM ( '' )  );
#50409=CARTESIAN_POINT ( 'NONE',  ( 27.15937500061451360, 0.000000000000000000, 4.756430356249998326 ) ) ;
#50415=CARTESIAN_POINT ( 'NONE',  ( 27.07499999999999929, 6.123233995736764310E-16, -4.999999999999998224 ) ) ;
#50422=CARTESIAN_POINT ( 'NONE',  ( 12.84375000122903288, 5.773502691896255534, 3.535250795749688894E-16 ) ) ;
#50424=CARTESIAN_POINT ( 'NONE',  ( 13.96875000122903465, -5.773502691896255534, -1.060575238724906372E-15 ) ) ;
#50426=CARTESIAN_POINT ( 'NONE',  ( 21.30937500061451217, -5.492252693125287522, -1.008910452111647106E-15 ) ) ;
#50433=ADVANCED_FACE ( 'NONE', ( #17850 ), #62929, .T. ) ;
#50434=CARTESIAN_POINT ( 'NONE',  ( 20.54999999999999716, 0.000000000000000000, 4.999999999999998224 ) ) ;
#50438=CARTESIAN_POINT ( 'NONE',  ( 13.69687500061451679, -4.119189519843965641, -2.378215178125001383 ) ) ;
#50451=VERTEX_POINT ( 'NONE', #3067 ) ;
#50459=CARTESIAN_POINT ( 'NONE',  ( 29.63437500061451857, 5.492252693125287522, 3.363034840372157021E-16 ) ) ;
#50460=CARTESIAN_POINT ( 'NONE',  ( 14.40937500061451715, 4.119189519843966529, -2.378215178124998275 ) ) ;
#50478=CARTESIAN_POINT ( 'NONE',  ( 25.63125000122903074, -4.330127018922194537, 2.499999999999995559 ) ) ;
#50480=CARTESIAN_POINT ( 'NONE',  ( 0.000000000000000000, 4.999999999999998224, 0.000000000000000000 ) ) ;
#50505=EDGE_CURVE ( 'NONE', #30573, #59457, #1012, .T. ) ;
#50518=VERTEX_POINT ( 'NONE', #43330 ) ;
#50524=CARTESIAN_POINT ( 'NONE',  ( 20.78437500061451360, -2.746126346562646425, 4.756430356249996549 ) ) ;
#50535=CARTESIAN_POINT ( 'NONE',  ( 10.35000000000000142, -4.330127018922190985, -2.500000000000001332 ) ) ;
#50541=CARTESIAN_POINT ( 'NONE',  ( 22.20937500061451431, 0.000000000000000000, 4.756430356249998326 ) ) ;
#50544=CARTESIAN_POINT ( 'NONE',  ( 12.78749999999999787, 5.773502691896255534, 3.535250795749688401E-16 ) ) ;
#50558=DIRECTION ( 'NONE',  ( -0.000000000000000000, 6.195440985631455317E-17, 1.000000000000000000 ) ) ;
#50564=CARTESIAN_POINT ( 'NONE',  ( 7.996875000614519280, -2.746126346562641984, -4.756430356249999214 ) ) ;
#50575=CARTESIAN_POINT ( 'NONE',  ( 45.00000000000000000, 0.000000000000000000, 0.000000000000000000 ) ) ;
#50585=CARTESIAN_POINT ( 'NONE',  ( 11.48437500061451644, -4.119189519843968306, 2.378215178124996054 ) ) ;
#50602=CYLINDRICAL_SURFACE ( 'NONE', #2511, 4.999999999999998224 ) ;
#50603=( BOUNDED_CURVE ( )  B_SPLINE_CURVE ( 2, ( #52188, #1590, #18180, #24100, #41113, #40749, #51107 ),
 .UNSPECIFIED., .F., .F. ) 
 B_SPLINE_CURVE_WITH_KNOTS ( ( 3, 2, 2, 3 ),
 ( 0.3800000000000000044, 0.3833333333333333592, 0.3866666666666666585, 0.3900000000000000133 ),
 .UNSPECIFIED. ) 
 CURVE ( )  GEOMETRIC_REPRESENTATION_ITEM ( )  RATIONAL_B_SPLINE_CURVE ( ( 1.000000000000000000, 0.8660254037844387076, 1.000000000000000000, 0.8660254037844387076, 1.000000000000000000, 0.8660254037844387076, 1.000000000000000000 ) ) 
 REPRESENTATION_ITEM ( '' )  );
#50605=CARTESIAN_POINT ( 'NONE',  ( 19.62187500061451573, 5.824947211148865298E-16, -4.756430356249998326 ) ) ;
#50608=CARTESIAN_POINT ( 'NONE',  ( 15.24375000122903323, -2.886751345948129988, 4.999999999999997335 ) ) ;
#50616=CARTESIAN_POINT ( 'NONE',  ( 15.80625000122903145, -4.330127018922190985, -2.500000000000001332 ) ) ;
#50622=CARTESIAN_POINT ( 'NONE',  ( 7.471875000614514484, 5.824947211148865298E-16, -4.756430356249998326 ) ) ;
#50645=CARTESIAN_POINT ( 'NONE',  ( 14.14687500061451786, -2.746126346562646425, 4.756430356249996549 ) ) ;
#50659=ORIENTED_EDGE ( 'NONE', *, *, #36974, .F. ) ;
#50673=VERTEX_POINT ( 'NONE', #37412 ) ;
#50676=CARTESIAN_POINT ( 'NONE',  ( 18.79687500061451644, -2.746126346562642428, -4.756430356249999214 ) ) ;
#50679=EDGE_CURVE ( 'NONE', #14695, #31243, #48685, .T. ) ;
#50682=CARTESIAN_POINT ( 'NONE',  ( 18.89999999999999858, -4.330127018922190985, -2.500000000000001332 ) ) ;
#50686=CARTESIAN_POINT ( 'NONE',  ( 24.79687500061451644, 0.000000000000000000, 4.756430356249998326 ) ) ;
#50693=CARTESIAN_POINT ( 'NONE',  ( 27.90937500061451715, 2.746126346562643317, 4.756430356249998326 ) ) ;
#50695=CARTESIAN_POINT ( 'NONE',  ( 12.30937500061451573, -5.492252693125287522, -1.008910452111647106E-15 ) ) ;
#50706=ORIENTED_EDGE ( 'NONE', *, *, #163, .F. ) ;
#50720=ORIENTED_EDGE ( 'NONE', *, *, #46859, .F. ) ;
#50730=CARTESIAN_POINT ( 'NONE',  ( 23.93437500061451573, 4.119189519843966529, 2.378215178124999607 ) ) ;
#50741=CARTESIAN_POINT ( 'NONE',  ( 15.13125000122903252, 4.330127018922191873, 2.499999999999999556 ) ) ;
#50748=CARTESIAN_POINT ( 'NONE',  ( 15.99375000122903323, 5.773502691896255534, 3.535250795749688894E-16 ) ) ;
#50763=CARTESIAN_POINT ( 'NONE',  ( 26.97187500061451360, 2.746126346562645981, -4.756430356249997438 ) ) ;
#50768=ADVANCED_FACE ( 'NONE', ( #59563 ), #3444, .T. ) ;
#50770=CARTESIAN_POINT ( 'NONE',  ( 27.41250000000000142, -5.773502691896255534, -1.060575238724906372E-15 ) ) ;
#50778=CARTESIAN_POINT ( 'NONE',  ( 11.34375000122903465, -2.886751345948125991, -5.000000000000000000 ) ) ;
#50779=CARTESIAN_POINT ( 'NONE',  ( 13.23750000000000071, 5.773502691896255534, 3.535250795749688401E-16 ) ) ;
#50782=CARTESIAN_POINT ( 'NONE',  ( 21.57187500061451146, 4.119189519843966529, 2.378215178124999607 ) ) ;
#50788=CARTESIAN_POINT ( 'NONE',  ( 27.82499999999999929, -4.330127018922194537, 2.499999999999995559 ) ) ;
#50793=CARTESIAN_POINT ( 'NONE',  ( 12.08437500061451608, 5.492252693125287522, 3.363034840372157021E-16 ) ) ;
#50815=CARTESIAN_POINT ( 'NONE',  ( 13.38750000000000107, -2.886751345948130876, 4.999999999999996447 ) ) ;
#50817=CARTESIAN_POINT ( 'NONE',  ( 12.04687500061451821, -2.746126346562642428, -4.756430356249999214 ) ) ;
#50825=CARTESIAN_POINT ( 'NONE',  ( 7.950000000000001954, 0.000000000000000000, 4.999999999999998224 ) ) ;
#50826=( BOUNDED_CURVE ( )  B_SPLINE_CURVE ( 2, ( #38826, #44737, #33627, #60232, #61341, #32180, #27737 ),
 .UNSPECIFIED., .F., .F. ) 
 B_SPLINE_CURVE_WITH_KNOTS ( ( 3, 2, 2, 3 ),
 ( 0.6600000000000000311, 0.6633333333333333304, 0.6666666666666666297, 0.6700000000000000400 ),
 .UNSPECIFIED. ) 
 CURVE ( )  GEOMETRIC_REPRESENTATION_ITEM ( )  RATIONAL_B_SPLINE_CURVE ( ( 1.000000000000000000, 0.8660254037844387076, 1.000000000000000000, 0.8660254037844387076, 1.000000000000000000, 0.8660254037844387076, 1.000000000000000000 ) ) 
 REPRESENTATION_ITEM ( '' )  );
#50837=CARTESIAN_POINT ( 'NONE',  ( 26.08125000122903003, -4.330127018922194537, 2.499999999999995559 ) ) ;
#50852=EDGE_CURVE ( 'NONE', #19210, #28191, #39246, .T. ) ;
#50867=CARTESIAN_POINT ( 'NONE',  ( 26.11875000122902790, -5.773502691896255534, -1.060575238724906372E-15 ) ) ;
#50882=CARTESIAN_POINT ( 'NONE',  ( 17.97187500061451360, 4.119189519843966529, 2.378215178124999607 ) ) ;
#50897=CARTESIAN_POINT ( 'NONE',  ( 18.26249999999999929, 2.886751345948126879, 4.999999999999998224 ) ) ;
#50898=CARTESIAN_POINT ( 'NONE',  ( 19.17187500061451999, -5.492252693125287522, -1.008910452111647106E-15 ) ) ;
#50906=EDGE_CURVE ( 'NONE', #1518, #31518, #63352, .T. ) ;
#50917=CARTESIAN_POINT ( 'NONE',  ( 45.00000000000000000, 2.500000000000000444, 3.499999999999999112 ) ) ;
#50922=CARTESIAN_POINT ( 'NONE',  ( 8.071875000614518569, 2.746126346562645981, -4.756430356249997438 ) ) ;
#50932=ORIENTED_EDGE ( 'NONE', *, *, #26912, .F. ) ;
#50943=CARTESIAN_POINT ( 'NONE',  ( 10.05937500061451750, 0.000000000000000000, 4.756430356249998326 ) ) ;
#50955=CARTESIAN_POINT ( 'NONE',  ( 24.24375000122903145, -2.886751345948143310, 4.999999999999972466 ) ) ;
#50961=( BOUNDED_CURVE ( )  B_SPLINE_CURVE ( 2, ( #38258, #53801, #3564, #32728, #21264, #26455, #48995 ),
 .UNSPECIFIED., .F., .F. ) 
 B_SPLINE_CURVE_WITH_KNOTS ( ( 3, 2, 2, 3 ),
 ( 0.5600000000000000533, 0.5633333333333333526, 0.5666666666666667629, 0.5700000000000000622 ),
 .UNSPECIFIED. ) 
 CURVE ( )  GEOMETRIC_REPRESENTATION_ITEM ( )  RATIONAL_B_SPLINE_CURVE ( ( 1.000000000000000000, 0.8660254037844387076, 1.000000000000000000, 0.8660254037844387076, 1.000000000000000000, 0.8660254037844342667, 1.000000000000004441 ) ) 
 REPRESENTATION_ITEM ( '' )  );
#50964=CARTESIAN_POINT ( 'NONE',  ( 17.18437500061451573, -2.746126346562646425, 4.756430356249996549 ) ) ;
#50967=CARTESIAN_POINT ( 'NONE',  ( 27.00937500061451502, 2.746126346562643317, 4.756430356249998326 ) ) ;
#50974=CARTESIAN_POINT ( 'NONE',  ( 15.65625000122903465, 0.000000000000000000, 4.999999999999998224 ) ) ;
#50980=CARTESIAN_POINT ( 'NONE',  ( 29.85937500061451644, 0.000000000000000000, 4.756430356249998326 ) ) ;
#50990=ORIENTED_EDGE ( 'NONE', *, *, #25676, .T. ) ;
#51001=CARTESIAN_POINT ( 'NONE',  ( 14.52187500061451786, 2.746126346562643317, 4.756430356249998326 ) ) ;
#51006=EDGE_CURVE ( 'NONE', #41736, #58199, #27978, .T. ) ;
#51031=EDGE_LOOP ( 'NONE', ( #39353, #51160, #20296, #55811 ) ) ;
#51034=CARTESIAN_POINT ( 'NONE',  ( 16.58437500061451786, 5.824947211148865298E-16, -4.756430356249998326 ) ) ;
#51035=CARTESIAN_POINT ( 'NONE',  ( 14.68125000122903323, 4.330127018922191873, 2.499999999999999556 ) ) ;
#51041=CARTESIAN_POINT ( 'NONE',  ( 18.71249999999999858, 2.886751345948126879, 4.999999999999999112 ) ) ;
#51045=CARTESIAN_POINT ( 'NONE',  ( 26.03437500061451360, 5.492252693125287522, 3.363034840372157021E-16 ) ) ;
#51053=CARTESIAN_POINT ( 'NONE',  ( 24.98437500061451289, -2.746126346562642428, -4.756430356249999214 ) ) ;
#51056=CARTESIAN_POINT ( 'NONE',  ( 11.22187500061451537, 4.119189519843966529, 2.378215178124999607 ) ) ;
#51059=ORIENTED_EDGE ( 'NONE', *, *, #30907, .F. ) ;
#51064=CARTESIAN_POINT ( 'NONE',  ( 18.09375000122903288, -2.886751345948126435, -5.000000000000000000 ) ) ;
#51065=CARTESIAN_POINT ( 'NONE',  ( 18.63749999999999929, 5.773502691896255534, 3.535250795749688401E-16 ) ) ;
#51089=CARTESIAN_POINT ( 'NONE',  ( 21.64687500061451786, 5.492252693125287522, 3.363034840372157021E-16 ) ) ;
#51091=CARTESIAN_POINT ( 'NONE',  ( 24.95625000122903003, 4.330127018922192761, -2.499999999999997780 ) ) ;
#51097=CARTESIAN_POINT ( 'NONE',  ( 20.10000000000000142, 0.000000000000000000, 4.999999999999998224 ) ) ;
#51107=CARTESIAN_POINT ( 'NONE',  ( 21.22500000000000142, 6.123233995736764310E-16, -4.999999999999998224 ) ) ;
#51110=CARTESIAN_POINT ( 'NONE',  ( 15.58125000122903181, 4.330127018922191873, 2.499999999999999556 ) ) ;
#51122=ORIENTED_EDGE ( 'NONE', *, *, #15050, .F. ) ;
#51126=CARTESIAN_POINT ( 'NONE',  ( 25.35937500061451644, 0.000000000000000000, 4.756430356249998326 ) ) ;
#51131=CARTESIAN_POINT ( 'NONE',  ( 27.33750000000000213, -2.886751345948129988, 4.999999999999997335 ) ) ;
#51139=CARTESIAN_POINT ( 'NONE',  ( 11.56875000122903252, 2.886751345948126879, 4.999999999999999112 ) ) ;
#51143=CARTESIAN_POINT ( 'NONE',  ( 19.28437500061451360, 5.492252693125287522, 3.363034840372157021E-16 ) ) ;
#51146=VERTEX_POINT ( 'NONE', #33688 ) ;
#51149=CARTESIAN_POINT ( 'NONE',  ( 27.93749999999999645, -2.886751345948112224, -5.000000000000023981 ) ) ;
#51154=CARTESIAN_POINT ( 'NONE',  ( 13.24687500061451750, -4.119189519843965641, -2.378215178125001383 ) ) ;
#51160=ORIENTED_EDGE ( 'NONE', *, *, #8691, .T. ) ;
#51162=CARTESIAN_POINT ( 'NONE',  ( 13.68750000000000000, 5.773502691896255534, 3.535250795749688401E-16 ) ) ;
#51175=CARTESIAN_POINT ( 'NONE',  ( 29.40937500061451715, 0.000000000000000000, 4.756430356249998326 ) ) ;
#51179=CARTESIAN_POINT ( 'NONE',  ( 11.70937500061451608, 4.119189519843966529, -2.378215178124998275 ) ) ;
#51186=FACE_OUTER_BOUND ( 'NONE', #60234, .T. ) ;
#51187=EDGE_CURVE ( 'NONE', #39431, #36820, #31207, .T. ) ;
#51189=CARTESIAN_POINT ( 'NONE',  ( 11.83125000122903181, 6.123233995736764310E-16, -4.999999999999998224 ) ) ;
#51197=CARTESIAN_POINT ( 'NONE',  ( 22.40625000122903288, 0.000000000000000000, 4.999999999999998224 ) ) ;
#51225=CARTESIAN_POINT ( 'NONE',  ( 45.00000000000000000, 0.000000000000000000, 0.000000000000000000 ) ) ;
#51244=CARTESIAN_POINT ( 'NONE',  ( 18.94687500061451857, 0.000000000000000000, 4.756430356249998326 ) ) ;
#51254=ORIENTED_EDGE ( 'NONE', *, *, #62210, .T. ) ;
#51260=FACE_OUTER_BOUND ( 'NONE', #31075, .T. ) ;
#51261=CARTESIAN_POINT ( 'NONE',  ( 18.94687500061451502, 5.492252693125287522, 3.363034840372157021E-16 ) ) ;
#51292=DIRECTION ( 'NONE',  ( -1.000000000000000000, -0.000000000000000000, -0.000000000000000000 ) ) ;
#51304=CARTESIAN_POINT ( 'NONE',  ( 8.821875000614518569, -5.492252693125287522, -1.008910452111647106E-15 ) ) ;
#51327=CARTESIAN_POINT ( 'NONE',  ( 18.49687500061451573, 0.000000000000000000, 4.756430356249998326 ) ) ;
#51330=CARTESIAN_POINT ( 'NONE',  ( 25.43437500061451217, -2.746126346562642428, -4.756430356249999214 ) ) ;
#51344=CARTESIAN_POINT ( 'NONE',  ( 26.22187500061451715, 2.746126346562643317, 4.756430356249998326 ) ) ;
#51349=CARTESIAN_POINT ( 'NONE',  ( 24.73125000122903216, -4.330127018922194537, 2.499999999999995559 ) ) ;
#51363=CARTESIAN_POINT ( 'NONE',  ( 15.90937500061451892, 0.000000000000000000, 4.756430356249998326 ) ) ;
#51375=VECTOR ( 'NONE', #18365, 1000.000000000000000 ) ;
#51393=AXIS2_PLACEMENT_3D ( 'NONE', #22257, #39627, #17428 ) ;
#51395=CARTESIAN_POINT ( 'NONE',  ( 16.88437500061451502, -4.119189519843968306, 2.378215178124996054 ) ) ;
#51396=DIRECTION ( 'NONE',  ( -1.000000000000000000, -0.000000000000000000, -0.000000000000000000 ) ) ;
#51398=( BOUNDED_CURVE ( )  B_SPLINE_CURVE ( 2, ( #51189, #68545, #28295, #68187, #67468, #6120, #22380 ),
 .UNSPECIFIED., .F., .F. ) 
 B_SPLINE_CURVE_WITH_KNOTS ( ( 3, 2, 2, 3 ),
 ( 0.7900000000000001465, 0.7933333333333334458, 0.7966666666666666341, 0.8000000000000000444 ),
 .UNSPECIFIED. ) 
 CURVE ( )  GEOMETRIC_REPRESENTATION_ITEM ( )  RATIONAL_B_SPLINE_CURVE ( ( 0.9999999999999955591, 0.8660254037844431485, 1.000000000000000000, 0.8660254037844387076, 1.000000000000000000, 0.8660254037844387076, 1.000000000000000000 ) ) 
 REPRESENTATION_ITEM ( '' )  );
#51402=CARTESIAN_POINT ( 'NONE',  ( 16.91250000000000142, 2.886751345948126879, 4.999999999999999112 ) ) ;
#51406=CARTESIAN_POINT ( 'NONE',  ( 25.24687500061451217, 0.000000000000000000, 4.756430356249998326 ) ) ;
#51414=CARTESIAN_POINT ( 'NONE',  ( 23.97187500061451715, -4.119189519843968306, 2.378215178124996054 ) ) ;
#51416=CARTESIAN_POINT ( 'NONE',  ( 10.73437500061451644, 5.492252693125287522, 3.363034840372157021E-16 ) ) ;
#51417=VECTOR ( 'NONE', #27068, 1000.000000000000000 ) ;
#51429=CARTESIAN_POINT ( 'NONE',  ( 11.78437500061451360, -2.746126346562646425, 4.756430356249996549 ) ) ;
#51440=EDGE_LOOP ( 'NONE', ( #26428, #71187, #68062, #24165 ) ) ;
#51450=CARTESIAN_POINT ( 'NONE',  ( 21.45937500061451786, -4.119189519843965641, -2.378215178125001383 ) ) ;
#51470=CARTESIAN_POINT ( 'NONE',  ( 17.08125000122903003, -4.330127018922194537, 2.499999999999995559 ) ) ;
#51485=ORIENTED_EDGE ( 'NONE', *, *, #25902, .T. ) ;
#51489=CARTESIAN_POINT ( 'NONE',  ( 24.64687500061451431, -2.746126346562642428, -4.756430356249999214 ) ) ;
#51494=CARTESIAN_POINT ( 'NONE',  ( 24.00000000000000000, 4.330127018922192761, -2.499999999999997780 ) ) ;
#51504=CARTESIAN_POINT ( 'NONE',  ( 8.756250001229034297, 4.330127018922192761, -2.499999999999997780 ) ) ;
#51508=CARTESIAN_POINT ( 'NONE',  ( 18.38437500061451857, 5.492252693125287522, 3.363034840372157021E-16 ) ) ;
#51520=CARTESIAN_POINT ( 'NONE',  ( 10.24687500061451395, 4.119189519843966529, -2.378215178124998275 ) ) ;
#51527=CARTESIAN_POINT ( 'NONE',  ( 19.72499999999999787, -4.330127018922194537, 2.499999999999995559 ) ) ;
#51541=CARTESIAN_POINT ( 'NONE',  ( 29.44687500061451502, -2.746126346562646425, 4.756430356249996549 ) ) ;
#51544=CARTESIAN_POINT ( 'NONE',  ( 27.68437500061451573, -2.746126346562641984, -4.756430356249999214 ) ) ;
#51545=CARTESIAN_POINT ( 'NONE',  ( 13.09687500061451892, 5.492252693125287522, 3.363034840372157021E-16 ) ) ;
#51561=CARTESIAN_POINT ( 'NONE',  ( 22.66875000122902861, 2.886751345948129099, -4.999999999999998224 ) ) ;
#51587=DIRECTION ( 'NONE',  ( 0.000000000000000000, 0.000000000000000000, 1.000000000000000000 ) ) ;
#51591=EDGE_CURVE ( 'NONE', #37967, #71135, #7394, .T. ) ;
#51596=CARTESIAN_POINT ( 'NONE',  ( 19.21875000122902932, 2.886751345948126879, 4.999999999999998224 ) ) ;
#51602=CARTESIAN_POINT ( 'NONE',  ( 29.04375000122903572, 5.773502691896255534, 3.535250795749688401E-16 ) ) ;
#51610=CARTESIAN_POINT ( 'NONE',  ( 20.14687500061451786, 4.119189519843966529, -2.378215178124998275 ) ) ;
#51619=ORIENTED_EDGE ( 'NONE', *, *, #19740, .F. ) ;
#51627=CYLINDRICAL_SURFACE ( 'NONE', #25677, 4.999999999999998224 ) ;
#51628=CARTESIAN_POINT ( 'NONE',  ( 20.52187500061451786, -5.492252693125287522, -1.008910452111647106E-15 ) ) ;
#51644=CARTESIAN_POINT ( 'NONE',  ( 20.98125000122903216, 4.330127018922191873, 2.499999999999999556 ) ) ;
#51669=CARTESIAN_POINT ( 'NONE',  ( 8.184375000614515727, 4.119189519843966529, 2.378215178124999607 ) ) ;
#51676=EDGE_CURVE ( 'NONE', #40722, #46244, #30291, .T. ) ;
#51690=CARTESIAN_POINT ( 'NONE',  ( 16.80937500061451573, -5.492252693125287522, -1.008910452111647106E-15 ) ) ;
#51693=CARTESIAN_POINT ( 'NONE',  ( 26.52187500061451431, 4.119189519843966529, 2.378215178124999607 ) ) ;
#51697=CARTESIAN_POINT ( 'NONE',  ( 45.00000000000000000, 0.000000000000000000, 4.999999999999998224 ) ) ;
#51708=CARTESIAN_POINT ( 'NONE',  ( 27.42187500061451644, 2.746126346562645981, -4.756430356249997438 ) ) ;
#51727=CARTESIAN_POINT ( 'NONE',  ( 14.33437500061451786, 5.824947211148865298E-16, -4.756430356249998326 ) ) ;
#51734=EDGE_CURVE ( 'NONE', #24022, #64545, #23342, .T. ) ;
#51739=EDGE_CURVE ( 'NONE', #70443, #40553, #3069, .T. ) ;
#51759=CARTESIAN_POINT ( 'NONE',  ( 16.39687500061451786, -2.746126346562646425, 4.756430356249996549 ) ) ;
#51766=CARTESIAN_POINT ( 'NONE',  ( 17.06250000000000000, -5.773502691896255534, -1.060575238724906372E-15 ) ) ;
#51770=CARTESIAN_POINT ( 'NONE',  ( 23.29687500061451644, 4.119189519843966529, -2.378215178124998275 ) ) ;
#51776=CARTESIAN_POINT ( 'NONE',  ( 25.92187500061451644, 5.824947211148865298E-16, -4.756430356249998326 ) ) ;
#51778=CARTESIAN_POINT ( 'NONE',  ( 10.43437500061451395, -2.746126346562646425, 4.756430356249996549 ) ) ;
#51781=VERTEX_POINT ( 'NONE', #23651 ) ;
#51787=ORIENTED_EDGE ( 'NONE', *, *, #34726, .F. ) ;
#51789=CARTESIAN_POINT ( 'NONE',  ( 11.89687500061451608, -4.119189519843965641, -2.378215178125001383 ) ) ;
#51806=DIRECTION ( 'NONE',  ( -1.000000000000000000, -0.000000000000000000, -0.000000000000000000 ) ) ;
#51808=CARTESIAN_POINT ( 'NONE',  ( 22.99687500061452283, 5.492252693125287522, 3.363034840372157021E-16 ) ) ;
#51810=CARTESIAN_POINT ( 'NONE',  ( 24.91875000122902861, 2.886751345948101122, -5.000000000000046185 ) ) ;
#51825=CARTESIAN_POINT ( 'NONE',  ( 28.64999999999999858, 0.000000000000000000, 4.999999999999998224 ) ) ;
#51828=CARTESIAN_POINT ( 'NONE',  ( 16.55625000122903145, 0.000000000000000000, 4.999999999999998224 ) ) ;
#51845=CARTESIAN_POINT ( 'NONE',  ( 22.84687500061451715, -2.746126346562642428, -4.756430356249999214 ) ) ;
#51850=CARTESIAN_POINT ( 'NONE',  ( 23.92499999999999716, 6.123233995736764310E-16, -4.999999999999998224 ) ) ;
#51854=EDGE_CURVE ( 'NONE', #65422, #65176, #20967, .T. ) ;
#51856=CARTESIAN_POINT ( 'NONE',  ( 24.56249999999999645, 2.886751345948112668, 5.000000000000023981 ) ) ;
#51860=CARTESIAN_POINT ( 'NONE',  ( 8.531250001229034652, -4.330127018922194537, 2.499999999999995559 ) ) ;
#51863=CARTESIAN_POINT ( 'NONE',  ( 18.04687500061451644, 0.000000000000000000, 4.756430356249998326 ) ) ;
#51875=DIRECTION ( 'NONE',  ( 0.000000000000000000, 0.000000000000000000, 1.000000000000000000 ) ) ;
#51876=CARTESIAN_POINT ( 'NONE',  ( 11.10937500061451821, 2.746126346562645981, -4.756430356249997438 ) ) ;
#51877=ORIENTED_EDGE ( 'NONE', *, *, #24198, .T. ) ;
#51880=( BOUNDED_CURVE ( )  B_SPLINE_CURVE ( 2, ( #41647, #29115, #24286, #70081, #46834, #63452, #58622 ),
 .UNSPECIFIED., .F., .F. ) 
 B_SPLINE_CURVE_WITH_KNOTS ( ( 3, 2, 2, 3 ),
 ( 0.6700000000000000400, 0.6733333333333333393, 0.6766666666666667496, 0.6800000000000001599 ),
 .UNSPECIFIED. ) 
 CURVE ( )  GEOMETRIC_REPRESENTATION_ITEM ( )  RATIONAL_B_SPLINE_CURVE ( ( 1.000000000000000000, 0.8660254037844387076, 1.000000000000000000, 0.8660254037844387076, 1.000000000000000000, 0.8660254037844342667, 1.000000000000004441 ) ) 
 REPRESENTATION_ITEM ( '' )  );
#51890=CARTESIAN_POINT ( 'NONE',  ( 9.750000000000001776, 0.000000000000000000, 4.999999999999998224 ) ) ;
#51899=CARTESIAN_POINT ( 'NONE',  ( 29.74687500061451573, 5.492252693125287522, 3.363034840372157021E-16 ) ) ;
#51901=CARTESIAN_POINT ( 'NONE',  ( 27.38437500061451502, 5.492252693125287522, 3.363034840372157021E-16 ) ) ;
#51902=CARTESIAN_POINT ( 'NONE',  ( 13.80937500061451750, -4.119189519843965641, -2.378215178125001383 ) ) ;
#51910=( BOUNDED_CURVE ( )  B_SPLINE_CURVE ( 2, ( #32716, #72970, #66329, #33801, #44547, #16437, #21988 ),
 .UNSPECIFIED., .F., .F. ) 
 B_SPLINE_CURVE_WITH_KNOTS ( ( 3, 2, 2, 3 ),
 ( 0.3699999999999999956, 0.3733333333333333504, 0.3766666666666666496, 0.3800000000000000044 ),
 .UNSPECIFIED. ) 
 CURVE ( )  GEOMETRIC_REPRESENTATION_ITEM ( )  RATIONAL_B_SPLINE_CURVE ( ( 1.000000000000000000, 0.8660254037844387076, 1.000000000000000000, 0.8660254037844387076, 1.000000000000000000, 0.8660254037844387076, 1.000000000000000000 ) ) 
 REPRESENTATION_ITEM ( '' )  );
#51915=SURFACE_STYLE_FILL_AREA ( #19355 ) ;
#51920=CARTESIAN_POINT ( 'NONE',  ( 23.15625000122903288, 4.330127018922192761, -2.499999999999997780 ) ) ;
#51945=CARTESIAN_POINT ( 'NONE',  ( 18.58125000122903003, 6.123233995736764310E-16, -4.999999999999998224 ) ) ;
#51953=CARTESIAN_POINT ( 'NONE',  ( 18.03749999999999787, -2.886751345948126435, -5.000000000000000000 ) ) ;
#51956=ORIENTED_EDGE ( 'NONE', *, *, #53564, .T. ) ;
#51957=CARTESIAN_POINT ( 'NONE',  ( 34.99999999999999289, -2.499999999999999556, 3.499999999999999556 ) ) ;
#51962=CARTESIAN_POINT ( 'NONE',  ( 11.25000000000000000, -4.330127018922190985, -2.500000000000001332 ) ) ;
#51968=ORIENTED_EDGE ( 'NONE', *, *, #21481, .T. ) ;
#51971=CARTESIAN_POINT ( 'NONE',  ( 18.83437500061451786, 5.492252693125287522, 3.363034840372157021E-16 ) ) ;
#51975=DIRECTION ( 'NONE',  ( -1.000000000000000000, -0.000000000000000000, -0.000000000000000000 ) ) ;
#51980=ORIENTED_EDGE ( 'NONE', *, *, #45339, .T. ) ;
#51987=CARTESIAN_POINT ( 'NONE',  ( 19.62187500061451573, -5.492252693125287522, -1.008910452111647106E-15 ) ) ;
#52005=CARTESIAN_POINT ( 'NONE',  ( 21.05625000122903145, 0.000000000000000000, 4.999999999999998224 ) ) ;
#52010=CARTESIAN_POINT ( 'NONE',  ( 8.296875000614518214, -2.746126346562646425, 4.756430356249996549 ) ) ;
#52031=CARTESIAN_POINT ( 'NONE',  ( 8.109375000614518214, 4.119189519843966529, -2.378215178124998275 ) ) ;
#52042=CARTESIAN_POINT ( 'NONE',  ( 9.674999999999998934, 4.330127018922191873, 2.499999999999999556 ) ) ;
#52051=CARTESIAN_POINT ( 'NONE',  ( 16.69687500061451502, 0.000000000000000000, 4.756430356249998326 ) ) ;
#52054=CARTESIAN_POINT ( 'NONE',  ( 27.19687500061451502, -4.119189519843965641, -2.378215178125001383 ) ) ;
#52068=CARTESIAN_POINT ( 'NONE',  ( 27.34687500061451360, -2.746126346562642428, -4.756430356249999214 ) ) ;
#52071=CARTESIAN_POINT ( 'NONE',  ( 18.07499999999999929, 6.123233995736764310E-16, -4.999999999999998224 ) ) ;
#52075=CARTESIAN_POINT ( 'NONE',  ( 9.393750001229035362, -2.886751345948130876, 4.999999999999996447 ) ) ;
#52077=ORIENTED_EDGE ( 'NONE', *, *, #47659, .F. ) ;
#52087=CARTESIAN_POINT ( 'NONE',  ( 13.99687500061451928, 5.492252693125287522, 3.363034840372157021E-16 ) ) ;
#52100=DIRECTION ( 'NONE',  ( 1.000000000000000000, -0.000000000000000000, -0.000000000000000000 ) ) ;
#52109=MECHANICAL_DESIGN_GEOMETRIC_PRESENTATION_REPRESENTATION('',(#3706),#47508);
#52114=( BOUNDED_CURVE ( )  B_SPLINE_CURVE ( 2, ( #34132, #23766, #11614, #902, #63654, #35225, #46319 ),
 .UNSPECIFIED., .F., .F. ) 
 B_SPLINE_CURVE_WITH_KNOTS ( ( 3, 2, 2, 3 ),
 ( 0.2900000000000000355, 0.2933333333333333903, 0.2966666666666666896, 0.2999999999999999889 ),
 .UNSPECIFIED. ) 
 CURVE ( )  GEOMETRIC_REPRESENTATION_ITEM ( )  RATIONAL_B_SPLINE_CURVE ( ( 0.9999999999999977796, 0.8660254037844409281, 1.000000000000000000, 0.8660254037844387076, 1.000000000000000000, 0.8660254037844387076, 1.000000000000000000 ) ) 
 REPRESENTATION_ITEM ( '' )  );
#52120=CARTESIAN_POINT ( 'NONE',  ( 15.68437500061451573, 5.824947211148865298E-16, -4.756430356249998326 ) ) ;
#52126=CARTESIAN_POINT ( 'NONE',  ( 17.92500000000000071, -4.330127018922194537, 2.499999999999995559 ) ) ;
#52129=CARTESIAN_POINT ( 'NONE',  ( 23.59687500061451360, -4.119189519843965641, -2.378215178125001383 ) ) ;
#52130=CARTESIAN_POINT ( 'NONE',  ( 26.39999999999999858, 0.000000000000000000, 4.999999999999998224 ) ) ;
#52136=CARTESIAN_POINT ( 'NONE',  ( 24.53437500061451715, -2.746126346562642428, -4.756430356249999214 ) ) ;
#52138=CARTESIAN_POINT ( 'NONE',  ( 10.65937500061451715, 2.746126346562645981, -4.756430356249997438 ) ) ;
#52148=EDGE_LOOP ( 'NONE', ( #42121, #36006, #36703, #59335 ) ) ;
#52150=CARTESIAN_POINT ( 'NONE',  ( 10.62187500061451395, 5.824947211148865298E-16, -4.756430356249998326 ) ) ;
#52157=DIRECTION ( 'NONE',  ( 0.000000000000000000, 0.000000000000000000, 1.000000000000000000 ) ) ;
#52169=CARTESIAN_POINT ( 'NONE',  ( 29.92500000000000071, 4.330127018922191873, 2.499999999999999556 ) ) ;
#52171=CARTESIAN_POINT ( 'NONE',  ( 22.47187500061452070, 2.746126346562645981, -4.756430356249997438 ) ) ;
#52188=CARTESIAN_POINT ( 'NONE',  ( 21.44999999999999929, 0.000000000000000000, 4.999999999999998224 ) ) ;
#52192=CYLINDRICAL_SURFACE ( 'NONE', #70294, 4.999999999999998224 ) ;
#52199=CARTESIAN_POINT ( 'NONE',  ( 7.331250001229031810, 6.123233995736764310E-16, -4.999999999999998224 ) ) ;
#52206=CARTESIAN_POINT ( 'NONE',  ( 23.74687500061451573, -2.746126346562642428, -4.756430356249999214 ) ) ;
#52212=CARTESIAN_POINT ( 'NONE',  ( 25.72499999999999787, 6.123233995736764310E-16, -4.999999999999998224 ) ) ;
#52220=ADVANCED_FACE ( 'NONE', ( #22229 ), #62832, .T. ) ;
#52222=CARTESIAN_POINT ( 'NONE',  ( 8.606250001229033941, -4.330127018922190985, -2.500000000000001332 ) ) ;
#52225=CARTESIAN_POINT ( 'NONE',  ( 18.23437500061451644, -2.746126346562641984, -4.756430356249999214 ) ) ;
#52228=ORIENTED_EDGE ( 'NONE', *, *, #39715, .T. ) ;
#52232=ADVANCED_FACE ( 'NONE', ( #56923 ), #34032, .T. ) ;
#52236=CARTESIAN_POINT ( 'NONE',  ( 10.17187500061451644, 5.824947211148865298E-16, -4.756430356249998326 ) ) ;
#52237=ORIENTED_EDGE ( 'NONE', *, *, #46464, .F. ) ;
#52250=CARTESIAN_POINT ( 'NONE',  ( 10.38750000000000107, -2.886751345948125991, -5.000000000000000000 ) ) ;
#52253=ORIENTED_EDGE ( 'NONE', *, *, #23045, .T. ) ;
#52260=CARTESIAN_POINT ( 'NONE',  ( 27.90937500061452070, 2.746126346562643317, 4.756430356249998326 ) ) ;
#52261=CARTESIAN_POINT ( 'NONE',  ( 12.12187500061451573, 2.746126346562645981, -4.756430356249997438 ) ) ;
#52268=DIRECTION ( 'NONE',  ( 0.000000000000000000, 0.000000000000000000, 1.000000000000000000 ) ) ;
#52277=CARTESIAN_POINT ( 'NONE',  ( 24.35625000122903216, -4.330127018922190985, -2.500000000000001332 ) ) ;
#52280=VERTEX_POINT ( 'NONE', #12226 ) ;
#52283=EDGE_CURVE ( 'NONE', #60154, #53798, #18580, .T. ) ;
#52286=CARTESIAN_POINT ( 'NONE',  ( 28.98750000000000071, 5.773502691896255534, 3.535250795749688401E-16 ) ) ;
#52301=CARTESIAN_POINT ( 'NONE',  ( 0.000000000000000000, 4.999999999999998224, 0.000000000000000000 ) ) ;
#52305=( BOUNDED_CURVE ( )  B_SPLINE_CURVE ( 2, ( #37072, #31540, #54080, #4931, #44466, #21172, #49633 ),
 .UNSPECIFIED., .F., .F. ) 
 B_SPLINE_CURVE_WITH_KNOTS ( ( 3, 2, 2, 3 ),
 ( 0.1699999999999999567, 0.1733333333333332837, 0.1766666666666666108, 0.1799999999999999378 ),
 .UNSPECIFIED. ) 
 CURVE ( )  GEOMETRIC_REPRESENTATION_ITEM ( )  RATIONAL_B_SPLINE_CURVE ( ( 1.000000000000002220, 0.8660254037844364872, 1.000000000000000000, 0.8660254037844387076, 1.000000000000000000, 0.8660254037844409281, 0.9999999999999977796 ) ) 
 REPRESENTATION_ITEM ( '' )  );
#52328=CARTESIAN_POINT ( 'NONE',  ( 18.90937500061451360, 2.746126346562643317, 4.756430356249998326 ) ) ;
#52346=CARTESIAN_POINT ( 'NONE',  ( 19.84687500061451360, 5.492252693125287522, 3.363034840372157021E-16 ) ) ;
#52366=CARTESIAN_POINT ( 'NONE',  ( 8.587500000000000355, -2.886751345948181946, -4.999999999999904077 ) ) ;
#52391=CARTESIAN_POINT ( 'NONE',  ( 10.17187500061451999, -5.492252693125287522, -1.008910452111647106E-15 ) ) ;
#52393=CARTESIAN_POINT ( 'NONE',  ( 45.00000000000000000, 0.000000000000000000, 0.000000000000000000 ) ) ;
#52410=CARTESIAN_POINT ( 'NONE',  ( 18.30937500061451573, 2.746126346562645981, -4.756430356249997438 ) ) ;
#52413=CARTESIAN_POINT ( 'NONE',  ( 25.24687500061451217, 0.000000000000000000, 4.756430356249998326 ) ) ;
#52430=CARTESIAN_POINT ( 'NONE',  ( 26.78437500061451360, -4.119189519843968306, 2.378215178124996054 ) ) ;
#52433=CARTESIAN_POINT ( 'NONE',  ( 45.00000000000000000, 6.123233995736764310E-16, -4.999999999999998224 ) ) ;
#52440=ORIENTED_EDGE ( 'NONE', *, *, #63109, .T. ) ;
#52450=CARTESIAN_POINT ( 'NONE',  ( 13.32187500061451502, -5.492252693125287522, -1.008910452111647106E-15 ) ) ;
#52462=CARTESIAN_POINT ( 'NONE',  ( 29.19375000122903074, -2.886751345948150860, 4.999999999999960920 ) ) ;
#52479=CARTESIAN_POINT ( 'NONE',  ( 16.32187500061451502, 2.746126346562643317, 4.756430356249998326 ) ) ;
#52485=CARTESIAN_POINT ( 'NONE',  ( 17.43750000000000355, -2.886751345948129988, 4.999999999999997335 ) ) ;
#52489=CARTESIAN_POINT ( 'NONE',  ( 23.22187500061451360, 5.824947211148865298E-16, -4.756430356249998326 ) ) ;
#52490=CARTESIAN_POINT ( 'NONE',  ( 26.28750000000000142, 5.773502691896255534, 3.535250795749688401E-16 ) ) ;
#52497=CARTESIAN_POINT ( 'NONE',  ( 24.38437500061451502, -2.746126346562646425, 4.756430356249996549 ) ) ;
#52499=CARTESIAN_POINT ( 'NONE',  ( 8.446875000614515017, 4.119189519843966529, -2.378215178124998275 ) ) ;
#52502=ORIENTED_EDGE ( 'NONE', *, *, #28533, .F. ) ;
#52508=CARTESIAN_POINT ( 'NONE',  ( 12.35625000122903394, 4.330127018922192761, -2.499999999999997780 ) ) ;
#52509=ORIENTED_EDGE ( 'NONE', *, *, #34544, .F. ) ;
#52511=CARTESIAN_POINT ( 'NONE',  ( 10.58437500061451608, -2.746126346562642428, -4.756430356249999214 ) ) ;
#52519=CARTESIAN_POINT ( 'NONE',  ( 23.58749999999999858, 5.773502691896255534, 3.535250795749688401E-16 ) ) ;
#52523=AXIS2_PLACEMENT_3D ( 'NONE', #54186, #41282, #63793 ) ;
#52529=CARTESIAN_POINT ( 'NONE',  ( 45.00000000000000000, 0.000000000000000000, 0.000000000000000000 ) ) ;
#52531=CARTESIAN_POINT ( 'NONE',  ( 20.37187500061451573, 2.746126346562643317, 4.756430356249998326 ) ) ;
#52537=ORIENTED_EDGE ( 'NONE', *, *, #25258, .F. ) ;
#52561=CARTESIAN_POINT ( 'NONE',  ( 45.00000000000000000, 0.000000000000000000, 0.000000000000000000 ) ) ;
#52568=CARTESIAN_POINT ( 'NONE',  ( 23.55937500061451573, 0.000000000000000000, 4.756430356249998326 ) ) ;
#52573=CARTESIAN_POINT ( 'NONE',  ( 25.16249999999999432, -5.773502691896255534, -1.060575238724906372E-15 ) ) ;
#52579=CARTESIAN_POINT ( 'NONE',  ( 18.31875000122903430, 2.886751345948182834, 4.999999999999902300 ) ) ;
#52583=CARTESIAN_POINT ( 'NONE',  ( 9.543750001229033941, -2.886751345948125991, -5.000000000000000000 ) ) ;
#52584=CARTESIAN_POINT ( 'NONE',  ( 8.849999999999999645, 0.000000000000000000, 4.999999999999998224 ) ) ;
#52586=CARTESIAN_POINT ( 'NONE',  ( 18.90937500061451360, 2.746126346562643317, 4.756430356249998326 ) ) ;
#52598=CARTESIAN_POINT ( 'NONE',  ( 11.33437500061451431, -2.746126346562646425, 4.756430356249996549 ) ) ;
#52599=VERTEX_POINT ( 'NONE', #63917 ) ;
#52607=CARTESIAN_POINT ( 'NONE',  ( 8.006250001229034297, 0.000000000000000000, 4.999999999999998224 ) ) ;
#52609=CARTESIAN_POINT ( 'NONE',  ( 28.65937500061451715, 2.746126346562645981, -4.756430356249997438 ) ) ;
#52612=CARTESIAN_POINT ( 'NONE',  ( 8.662499999999999645, 2.886751345948129099, -4.999999999999998224 ) ) ;
#52615=EDGE_LOOP ( 'NONE', ( #4866, #36055, #61369, #38531 ) ) ;
#52620=CARTESIAN_POINT ( 'NONE',  ( 28.05937500061451573, 0.000000000000000000, 4.756430356249998326 ) ) ;
#52622=CARTESIAN_POINT ( 'NONE',  ( 28.54687500061451644, -4.119189519843965641, -2.378215178125001383 ) ) ;
#52623=CARTESIAN_POINT ( 'NONE',  ( 10.92187500061451644, 2.746126346562643317, 4.756430356249998326 ) ) ;
#52637=CARTESIAN_POINT ( 'NONE',  ( 21.01875000122903003, 2.886751345948126879, 4.999999999999999112 ) ) ;
#52644=CARTESIAN_POINT ( 'NONE',  ( 7.893750001229031810, 5.773502691896255534, 3.535250795749688401E-16 ) ) ;
#52652=CARTESIAN_POINT ( 'NONE',  ( 29.82187500061451502, 2.746126346562643317, 4.756430356249998326 ) ) ;
#52659=CARTESIAN_POINT ( 'NONE',  ( 25.34999999999999787, 4.330127018922192761, -2.499999999999997780 ) ) ;
#52672=EDGE_LOOP ( 'NONE', ( #44481, #42089, #37022, #53059 ) ) ;
#52682=( BOUNDED_CURVE ( )  B_SPLINE_CURVE ( 2, ( #49321, #54854, #4263, #26786, #30852, #53387, #2782 ),
 .UNSPECIFIED., .F., .F. ) 
 B_SPLINE_CURVE_WITH_KNOTS ( ( 3, 2, 2, 3 ),
 ( 0.2200000000000000011, 0.2233333333333333282, 0.2266666666666666552, 0.2300000000000000100 ),
 .UNSPECIFIED. ) 
 CURVE ( )  GEOMETRIC_REPRESENTATION_ITEM ( )  RATIONAL_B_SPLINE_CURVE ( ( 1.000000000000000000, 0.8660254037844387076, 1.000000000000000000, 0.8660254037844387076, 1.000000000000000000, 0.8660254037844387076, 1.000000000000000000 ) ) 
 REPRESENTATION_ITEM ( '' )  );
#52688=CARTESIAN_POINT ( 'NONE',  ( 15.45937500061451608, -5.492252693125287522, -1.008910452111647106E-15 ) ) ;
#52696=CARTESIAN_POINT ( 'NONE',  ( 11.38125000122903252, 6.123233995736764310E-16, -4.999999999999998224 ) ) ;
#52697=ORIENTED_EDGE ( 'NONE', *, *, #7510, .F. ) ;
#52707=CARTESIAN_POINT ( 'NONE',  ( 17.22187500061451715, 2.746126346562643317, 4.756430356249998326 ) ) ;
#52727=CARTESIAN_POINT ( 'NONE',  ( 7.246875000614514839, 0.000000000000000000, 4.756430356249998326 ) ) ;
#52728=VECTOR ( 'NONE', #11366, 1000.000000000000000 ) ;
#52753=CARTESIAN_POINT ( 'NONE',  ( 29.69999999999999574, -4.330127018922190985, -2.500000000000001332 ) ) ;
#52762=CARTESIAN_POINT ( 'NONE',  ( 45.00000000000000000, 0.000000000000000000, 0.000000000000000000 ) ) ;
#52772=CARTESIAN_POINT ( 'NONE',  ( 14.25937500061451679, 2.746126346562645981, -4.756430356249997438 ) ) ;
#52775=CARTESIAN_POINT ( 'NONE',  ( 23.55937500061451573, -5.492252693125287522, -1.008910452111647106E-15 ) ) ;
#52782=CARTESIAN_POINT ( 'NONE',  ( 28.03125000122903288, 6.123233995736764310E-16, -4.999999999999998224 ) ) ;
#52791=CARTESIAN_POINT ( 'NONE',  ( 27.57187500061451857, 2.746126346562643317, 4.756430356249998326 ) ) ;
#52794=DIRECTION ( 'NONE',  ( 0.000000000000000000, 0.000000000000000000, 1.000000000000000000 ) ) ;
#52801=EDGE_LOOP ( 'NONE', ( #13312, #8483, #7518, #47830 ) ) ;
#52810=CARTESIAN_POINT ( 'NONE',  ( 12.08437500061451608, 5.824947211148865298E-16, -4.756430356249998326 ) ) ;
#52823=CARTESIAN_POINT ( 'NONE',  ( 29.15625000122903288, 0.000000000000000000, 4.999999999999998224 ) ) ;
#52832=VECTOR ( 'NONE', #30539, 1000.000000000000000 ) ;
#52841=CARTESIAN_POINT ( 'NONE',  ( 14.18437500061451750, -4.119189519843968306, 2.378215178124996054 ) ) ;
#52842=VECTOR ( 'NONE', #41413, 1000.000000000000000 ) ;
#52848=CARTESIAN_POINT ( 'NONE',  ( 18.03749999999999787, -2.886751345948125991, -5.000000000000000000 ) ) ;
#52852=CARTESIAN_POINT ( 'NONE',  ( 22.39687500061451431, 4.119189519843966529, -2.378215178124998275 ) ) ;
#52853=CARTESIAN_POINT ( 'NONE',  ( 15.82499999999999929, 6.123233995736764310E-16, -4.999999999999998224 ) ) ;
#52860=CARTESIAN_POINT ( 'NONE',  ( 22.05937500061451217, 2.746126346562643317, 4.756430356249998326 ) ) ;
#52862=CARTESIAN_POINT ( 'NONE',  ( 9.421875000614514661, 4.119189519843966529, 2.378215178124999607 ) ) ;
#52869=CARTESIAN_POINT ( 'NONE',  ( 19.23750000000000071, -2.886751345948157965, 4.999999999999948486 ) ) ;
#52870=CARTESIAN_POINT ( 'NONE',  ( 16.05000000000000071, 0.000000000000000000, 4.999999999999998224 ) ) ;
#52873=CARTESIAN_POINT ( 'NONE',  ( 11.40937500061451360, -5.492252693125287522, -1.008910452111647106E-15 ) ) ;
#52894=CARTESIAN_POINT ( 'NONE',  ( 18.34687500061451715, -2.746126346562641984, -4.756430356249999214 ) ) ;
#52925=ORIENTED_EDGE ( 'NONE', *, *, #59515, .T. ) ;
#52928=CARTESIAN_POINT ( 'NONE',  ( 24.68437500061451573, 5.824947211148865298E-16, -4.756430356249998326 ) ) ;
#52933=CARTESIAN_POINT ( 'NONE',  ( 24.60000000000000142, 0.000000000000000000, 4.999999999999998224 ) ) ;
#52937=CARTESIAN_POINT ( 'NONE',  ( 12.73125000122903394, 6.123233995736764310E-16, -4.999999999999998224 ) ) ;
#52944=CARTESIAN_POINT ( 'NONE',  ( 7.368750001229035007, 2.886751345948129099, -4.999999999999998224 ) ) ;
#52946=CARTESIAN_POINT ( 'NONE',  ( 16.43437500061451573, -2.746126346562641984, -4.756430356249999214 ) ) ;
#52958=CARTESIAN_POINT ( 'NONE',  ( 11.67187500061451644, 4.119189519843966529, 2.378215178124999607 ) ) ;
#52965=VERTEX_POINT ( 'NONE', #36943 ) ;
#52966=CARTESIAN_POINT ( 'NONE',  ( 10.23750000000000071, -2.886751345948130876, 4.999999999999996447 ) ) ;
#52970=CARTESIAN_POINT ( 'NONE',  ( 27.94687500061451502, 0.000000000000000000, 4.756430356249998326 ) ) ;
#52973=CARTESIAN_POINT ( 'NONE',  ( 8.849999999999999645, 0.000000000000000000, 4.999999999999998224 ) ) ;
#52981=CARTESIAN_POINT ( 'NONE',  ( 25.84687500061451715, -2.746126346562646425, 4.756430356249996549 ) ) ;
#52983=CARTESIAN_POINT ( 'NONE',  ( 10.20937500061451786, -4.119189519843965641, -2.378215178125001383 ) ) ;
#52999=CARTESIAN_POINT ( 'NONE',  ( 21.58125000122903359, -4.330127018922194537, 2.499999999999995559 ) ) ;
#53002=ORIENTED_EDGE ( 'NONE', *, *, #26320, .F. ) ;
#53007=CARTESIAN_POINT ( 'NONE',  ( 7.968750001229034652, 2.886751345948126879, 4.999999999999998224 ) ) ;
#53023=CARTESIAN_POINT ( 'NONE',  ( 25.31249999999999645, 2.886751345948101122, -5.000000000000046185 ) ) ;
#53038=CARTESIAN_POINT ( 'NONE',  ( 45.00000000000000000, 0.000000000000000000, 0.000000000000000000 ) ) ;
#53045=EDGE_CURVE ( 'NONE', #48156, #52599, #30900, .T. ) ;
#53050=CARTESIAN_POINT ( 'NONE',  ( 16.28437500061451715, -2.746126346562646425, 4.756430356249996549 ) ) ;
#53059=ORIENTED_EDGE ( 'NONE', *, *, #7959, .F. ) ;
#53066=CARTESIAN_POINT ( 'NONE',  ( 45.00000000000000000, 0.000000000000000000, 0.000000000000000000 ) ) ;
#53068=CARTESIAN_POINT ( 'NONE',  ( 28.03125000122903288, 6.123233995736764310E-16, -4.999999999999998224 ) ) ;
#53069=CARTESIAN_POINT ( 'NONE',  ( 18.27187500061451431, -5.492252693125287522, -1.008910452111647106E-15 ) ) ;
#53087=CARTESIAN_POINT ( 'NONE',  ( 27.69375000122902719, 5.773502691896255534, 3.535250795749688894E-16 ) ) ;
#53111=CARTESIAN_POINT ( 'NONE',  ( 7.771875000614516971, 2.746126346562643317, 4.756430356249998326 ) ) ;
#53113=FACE_OUTER_BOUND ( 'NONE', #52801, .T. ) ;
#53118=CARTESIAN_POINT ( 'NONE',  ( 27.41250000000000142, -5.773502691896255534, -1.060575238724906372E-15 ) ) ;
#53121=FACE_OUTER_BOUND ( 'NONE', #42025, .T. ) ;
#53131=CARTESIAN_POINT ( 'NONE',  ( 14.29687500061451644, 4.119189519843966529, -2.378215178124998275 ) ) ;
#53134=CARTESIAN_POINT ( 'NONE',  ( 23.85937500061451644, 2.746126346562643317, 4.756430356249998326 ) ) ;
#53138=CARTESIAN_POINT ( 'NONE',  ( 24.14999999999999858, 0.000000000000000000, 4.999999999999998224 ) ) ;
#53150=CARTESIAN_POINT ( 'NONE',  ( 23.82187500061451502, 2.746126346562645981, -4.756430356249997438 ) ) ;
#53154=CARTESIAN_POINT ( 'NONE',  ( 25.19999999999999929, -4.330127018922190985, -2.500000000000001332 ) ) ;
#53160=CARTESIAN_POINT ( 'NONE',  ( 7.256250001229033408, -4.330127018922190985, -2.500000000000001332 ) ) ;
#53170=CARTESIAN_POINT ( 'NONE',  ( 12.38437500061451857, -4.119189519843968306, 2.378215178124996054 ) ) ;
#53197=VERTEX_POINT ( 'NONE', #3713 ) ;
#53200=CARTESIAN_POINT ( 'NONE',  ( 15.04687500061451644, -2.746126346562646425, 4.756430356249996549 ) ) ;
#53206=CARTESIAN_POINT ( 'NONE',  ( 14.69999999999999929, 0.000000000000000000, 4.999999999999998224 ) ) ;
#53210=CARTESIAN_POINT ( 'NONE',  ( 22.54687500061451644, 0.000000000000000000, 4.756430356249998326 ) ) ;
#53211=CARTESIAN_POINT ( 'NONE',  ( 15.75000000000000000, -4.330127018922190985, -2.500000000000001332 ) ) ;
#53214=CARTESIAN_POINT ( 'NONE',  ( 26.47499999999999787, -4.330127018922194537, 2.499999999999995559 ) ) ;
#53218=CARTESIAN_POINT ( 'NONE',  ( 23.48437500061451644, -2.746126346562646425, 4.756430356249996549 ) ) ;
#53220=CARTESIAN_POINT ( 'NONE',  ( 8.296875000614518214, -4.119189519843965641, -2.378215178125001383 ) ) ;
#53229=ORIENTED_EDGE ( 'NONE', *, *, #32685, .T. ) ;
#53231=CARTESIAN_POINT ( 'NONE',  ( 10.02187500061451431, -4.119189519843968306, 2.378215178124996054 ) ) ;
#53254=CARTESIAN_POINT ( 'NONE',  ( 20.48437500061451289, -4.119189519843968306, 2.378215178124996054 ) ) ;
#53275=CARTESIAN_POINT ( 'NONE',  ( 45.00000000000000000, 0.000000000000000000, 4.999999999999998224 ) ) ;
#53288=CARTESIAN_POINT ( 'NONE',  ( 20.70937500061451786, 4.119189519843966529, -2.378215178124998275 ) ) ;
#53295=CARTESIAN_POINT ( 'NONE',  ( 22.19999999999999574, 4.330127018922192761, -2.499999999999997780 ) ) ;
#53306=CARTESIAN_POINT ( 'NONE',  ( 29.14687500061451431, 4.119189519843966529, -2.378215178124998275 ) ) ;
#53308=CARTESIAN_POINT ( 'NONE',  ( 17.07187500061451502, 4.119189519843966529, 2.378215178124999607 ) ) ;
#53311=VERTEX_POINT ( 'NONE', #42864 ) ;
#53320=CARTESIAN_POINT ( 'NONE',  ( 7.696875000614517681, 0.000000000000000000, 4.756430356249998326 ) ) ;
#53326=EDGE_CURVE ( 'NONE', #3324, #34631, #56387, .T. ) ;
#53333=CARTESIAN_POINT ( 'NONE',  ( 28.73437500061451644, 5.492252693125287522, 3.363034840372157021E-16 ) ) ;
#53336=CARTESIAN_POINT ( 'NONE',  ( 7.650000000000000355, -4.330127018922190985, -2.500000000000001332 ) ) ;
#53343=CARTESIAN_POINT ( 'NONE',  ( 27.00937500061451857, 4.119189519843966529, -2.378215178124998275 ) ) ;
#53345=CARTESIAN_POINT ( 'NONE',  ( 10.95937500061451964, 0.000000000000000000, 4.756430356249998326 ) ) ;
#53362=CARTESIAN_POINT ( 'NONE',  ( 21.24375000122903501, -2.886751345948125991, -5.000000000000000000 ) ) ;
#53373=VECTOR ( 'NONE', #15202, 1000.000000000000000 ) ;
#53378=CARTESIAN_POINT ( 'NONE',  ( 28.47187500061451715, 2.746126346562643317, 4.756430356249998326 ) ) ;
#53381=( BOUNDED_CURVE ( )  B_SPLINE_CURVE ( 2, ( #217, #44562, #72984, #22366, #44918, #50815, #22722 ),
 .UNSPECIFIED., .F., .F. ) 
 B_SPLINE_CURVE_WITH_KNOTS ( ( 3, 2, 2, 3 ),
 ( 0.7299999999999999822, 0.7333333333333332815, 0.7366666666666666918, 0.7399999999999999911 ),
 .UNSPECIFIED. ) 
 CURVE ( )  GEOMETRIC_REPRESENTATION_ITEM ( )  RATIONAL_B_SPLINE_CURVE ( ( 1.000000000000000000, 0.8660254037844387076, 1.000000000000000000, 0.8660254037844387076, 1.000000000000000000, 0.8660254037844387076, 1.000000000000000000 ) ) 
 REPRESENTATION_ITEM ( '' )  );
#53387=CARTESIAN_POINT ( 'NONE',  ( 24.86250000000000071, 2.886751345948129099, -4.999999999999997335 ) ) ;
#53403=CARTESIAN_POINT ( 'NONE',  ( 28.19999999999999929, 0.000000000000000000, 4.999999999999998224 ) ) ;
#53407=CARTESIAN_POINT ( 'NONE',  ( 11.21250000000000036, -5.773502691896255534, -1.060575238724906372E-15 ) ) ;
#53411=VERTEX_POINT ( 'NONE', #26976 ) ;
#53414=ADVANCED_FACE ( 'NONE', ( #72034 ), #21410, .T. ) ;
#53419=CARTESIAN_POINT ( 'NONE',  ( 17.14687500061451431, 0.000000000000000000, 4.756430356249998326 ) ) ;
#53421=( BOUNDED_CURVE ( )  B_SPLINE_CURVE ( 2, ( #57450, #57804, #36005, #63362, #64075, #69278, #12746 ),
 .UNSPECIFIED., .F., .F. ) 
 B_SPLINE_CURVE_WITH_KNOTS ( ( 3, 2, 2, 3 ),
 ( 0.3199999999999999512, 0.3233333333333333059, 0.3266666666666666607, 0.3300000000000000711 ),
 .UNSPECIFIED. ) 
 CURVE ( )  GEOMETRIC_REPRESENTATION_ITEM ( )  RATIONAL_B_SPLINE_CURVE ( ( 1.000000000000002220, 0.8660254037844364872, 1.000000000000000000, 0.8660254037844387076, 1.000000000000000000, 0.8660254037844364872, 1.000000000000002220 ) ) 
 REPRESENTATION_ITEM ( '' )  );
#53428=CARTESIAN_POINT ( 'NONE',  ( 45.00000000000000000, 0.000000000000000000, 0.000000000000000000 ) ) ;
#53436=DIRECTION ( 'NONE',  ( 0.000000000000000000, 0.000000000000000000, -1.000000000000000000 ) ) ;
#53439=CARTESIAN_POINT ( 'NONE',  ( 17.29687500061451999, -2.746126346562646425, 4.756430356249996549 ) ) ;
#53442=ADVANCED_FACE ( 'NONE', ( #60936 ), #10340, .T. ) ;
#53457=CARTESIAN_POINT ( 'NONE',  ( 27.13125000122903430, 6.123233995736764310E-16, -4.999999999999998224 ) ) ;
#53480=CARTESIAN_POINT ( 'NONE',  ( 17.64375000122903003, -2.886751345948126435, -5.000000000000000000 ) ) ;
#53481=CARTESIAN_POINT ( 'NONE',  ( 29.51249999999999929, 2.886751345948126879, 4.999999999999999112 ) ) ;
#53499=CARTESIAN_POINT ( 'NONE',  ( 14.70937500061451431, 2.746126346562645981, -4.756430356249997438 ) ) ;
#53502=CARTESIAN_POINT ( 'NONE',  ( 24.45937500061451786, -5.492252693125287522, -1.008910452111647106E-15 ) ) ;
#53518=CARTESIAN_POINT ( 'NONE',  ( 24.12187500061451217, -5.492252693125287522, -1.008910452111647106E-15 ) ) ;
#53521=LINE ( 'NONE', #7005, #14838 ) ;
#53529=VERTEX_POINT ( 'NONE', #33951 ) ;
#53538=CARTESIAN_POINT ( 'NONE',  ( 12.04687500061451821, -2.746126346562641984, -4.756430356249999214 ) ) ;
#53551=ORIENTED_EDGE ( 'NONE', *, *, #71833, .F. ) ;
#53564=EDGE_CURVE ( 'NONE', #34347, #63177, #68671, .T. ) ;
#53567=CARTESIAN_POINT ( 'NONE',  ( 14.82187500061451679, 2.746126346562645981, -4.756430356249997438 ) ) ;
#53574=CARTESIAN_POINT ( 'NONE',  ( 15.07499999999999929, 4.330127018922191873, 2.499999999999999556 ) ) ;
#53588=CARTESIAN_POINT ( 'NONE',  ( 22.95937500061451786, 2.746126346562643317, 4.756430356249998326 ) ) ;
#53590=CARTESIAN_POINT ( 'NONE',  ( 9.834375000614514306, 5.492252693125287522, 3.363034840372157021E-16 ) ) ;
#53594=CARTESIAN_POINT ( 'NONE',  ( 9.918750001229033941, -5.773502691896255534, -1.060575238724906372E-15 ) ) ;
#53599=CARTESIAN_POINT ( 'NONE',  ( 9.975000000000001421, 6.123233995736764310E-16, -4.999999999999998224 ) ) ;
#53600=ORIENTED_EDGE ( 'NONE', *, *, #34883, .T. ) ;
#53602=CARTESIAN_POINT ( 'NONE',  ( 8.784375000614515372, -2.746126346562642428, -4.756430356249999214 ) ) ;
#53626=CARTESIAN_POINT ( 'NONE',  ( 19.32187500061451857, 2.746126346562645981, -4.756430356249997438 ) ) ;
#53640=ORIENTED_EDGE ( 'NONE', *, *, #28075, .T. ) ;
#53655=ORIENTED_EDGE ( 'NONE', *, *, #4530, .T. ) ;
#53661=CARTESIAN_POINT ( 'NONE',  ( 21.83437500061451786, -4.119189519843968306, 2.378215178124996054 ) ) ;
#53665=EDGE_CURVE ( 'NONE', #50344, #51146, #28066, .T. ) ;
#53668=CARTESIAN_POINT ( 'NONE',  ( 22.01249999999999574, -5.773502691896255534, -1.060575238724906372E-15 ) ) ;
#53671=LINE ( 'NONE', #8601, #59549 ) ;
#53674=CARTESIAN_POINT ( 'NONE',  ( 19.63125000122903430, 4.330127018922191873, 2.499999999999999556 ) ) ;
#53678=CARTESIAN_POINT ( 'NONE',  ( 8.043750001229032165, -2.886751345948129988, 4.999999999999997335 ) ) ;
#53680=CARTESIAN_POINT ( 'NONE',  ( 15.57187500061451679, 5.824947211148865298E-16, -4.756430356249998326 ) ) ;
#53698=CARTESIAN_POINT ( 'NONE',  ( 10.31250000000000178, -5.773502691896255534, -1.060575238724906372E-15 ) ) ;
#53701=CARTESIAN_POINT ( 'NONE',  ( 19.74375000122903145, -2.886751345948130876, 4.999999999999996447 ) ) ;
#53703=CARTESIAN_POINT ( 'NONE',  ( 29.10937500061451999, 2.746126346562645981, -4.756430356249997438 ) ) ;
#53715=CARTESIAN_POINT ( 'NONE',  ( 26.63437500061451857, 4.119189519843966529, 2.378215178124999607 ) ) ;
#53717=CARTESIAN_POINT ( 'NONE',  ( 11.37187500061451750, 2.746126346562643317, 4.756430356249998326 ) ) ;
#53736=CARTESIAN_POINT ( 'NONE',  ( 20.08125000122903359, 4.330127018922191873, 2.499999999999999556 ) ) ;
#53750=CARTESIAN_POINT ( 'NONE',  ( 27.49687500061451217, 5.492252693125287522, 3.363034840372157021E-16 ) ) ;
#53758=VECTOR ( 'NONE', #55520, 1000.000000000000000 ) ;
#53769=CARTESIAN_POINT ( 'NONE',  ( 23.13749999999999929, 5.773502691896255534, 3.535250795749688401E-16 ) ) ;
#53774=DIRECTION ( 'NONE',  ( 0.000000000000000000, 0.000000000000000000, 1.000000000000000000 ) ) ;
#53777=CARTESIAN_POINT ( 'NONE',  ( 28.01249999999999574, 2.886751345948142866, -4.999999999999973355 ) ) ;
#53781=ORIENTED_EDGE ( 'NONE', *, *, #68789, .T. ) ;
#53785=CYLINDRICAL_SURFACE ( 'NONE', #28910, 5.000000000000000000 ) ;
#53788=CARTESIAN_POINT ( 'NONE',  ( 16.65937500061451715, 2.746126346562643317, 4.756430356249998326 ) ) ;
#53791=AXIS2_PLACEMENT_3D ( 'NONE', #36493, #70481, #69751 ) ;
#53798=VERTEX_POINT ( 'NONE', #22505 ) ;
#53801=CARTESIAN_POINT ( 'NONE',  ( 16.96875000122903288, 2.886751345948126879, 4.999999999999998224 ) ) ;
#53806=LINE ( 'NONE', #69700, #11538 ) ;
#53808=DIRECTION ( 'NONE',  ( -1.000000000000000000, 0.000000000000000000, 0.000000000000000000 ) ) ;
#53809=CARTESIAN_POINT ( 'NONE',  ( 17.93437500061451928, 5.824947211148865298E-16, -4.756430356249998326 ) ) ;
#53824=DIRECTION ( 'NONE',  ( 0.000000000000000000, 6.195440985631455317E-17, 1.000000000000000000 ) ) ;
#53828=CARTESIAN_POINT ( 'NONE',  ( 27.16875000122903216, 2.886751345948129099, -4.999999999999998224 ) ) ;
#53840=ORIENTED_EDGE ( 'NONE', *, *, #14279, .F. ) ;
#53854=CARTESIAN_POINT ( 'NONE',  ( 17.56875000122903074, -5.773502691896255534, -1.060575238724906372E-15 ) ) ;
#53856=CARTESIAN_POINT ( 'NONE',  ( 28.27499999999999858, -4.330127018922194537, 2.499999999999995559 ) ) ;
#53874=CARTESIAN_POINT ( 'NONE',  ( 16.28437500061451715, -2.746126346562646425, 4.756430356249996549 ) ) ;
#53878=CARTESIAN_POINT ( 'NONE',  ( 23.78437500061451360, 5.492252693125287522, 3.363034840372157021E-16 ) ) ;
#53883=CARTESIAN_POINT ( 'NONE',  ( 15.99375000122903145, 5.773502691896255534, 3.535250795749688401E-16 ) ) ;
#53889=CARTESIAN_POINT ( 'NONE',  ( 12.75000000000000178, 4.330127018922192761, -2.499999999999997780 ) ) ;
#53896=CARTESIAN_POINT ( 'NONE',  ( 25.32187500061451857, 2.746126346562643317, 4.756430356249998326 ) ) ;
#53916=CARTESIAN_POINT ( 'NONE',  ( 11.59687500061451892, -2.746126346562641984, -4.756430356249999214 ) ) ;
#53929=ORIENTED_EDGE ( 'NONE', *, *, #41327, .F. ) ;
#53944=CARTESIAN_POINT ( 'NONE',  ( 14.85937500061451644, 4.119189519843966529, -2.378215178124998275 ) ) ;
#53948=VECTOR ( 'NONE', #9932, 1000.000000000000000 ) ;
#53953=CARTESIAN_POINT ( 'NONE',  ( 14.77500000000000036, -4.330127018922194537, 2.499999999999995559 ) ) ;
#53956=CARTESIAN_POINT ( 'NONE',  ( 45.00000000000000000, 0.000000000000000000, 0.000000000000000000 ) ) ;
#53965=CARTESIAN_POINT ( 'NONE',  ( 22.50937500061451502, 2.746126346562643317, 4.756430356249998326 ) ) ;
#53967=CARTESIAN_POINT ( 'NONE',  ( 7.696875000614517681, 0.000000000000000000, 4.756430356249998326 ) ) ;
#53978=CARTESIAN_POINT ( 'NONE',  ( 9.496875000614517504, 0.000000000000000000, 4.756430356249998326 ) ) ;
#54001=AXIS2_PLACEMENT_3D ( 'NONE', #53066, #70057, #43084 ) ;
#54003=CARTESIAN_POINT ( 'NONE',  ( 19.17187500061451644, -5.492252693125287522, -1.008910452111647106E-15 ) ) ;
#54007=EDGE_CURVE ( 'NONE', #20756, #61022, #29864, .T. ) ;
#54016=ORIENTED_EDGE ( 'NONE', *, *, #2783, .T. ) ;
#54029=CYLINDRICAL_SURFACE ( 'NONE', #22676, 4.999999999999998224 ) ;
#54032=ORIENTED_EDGE ( 'NONE', *, *, #47475, .F. ) ;
#54036=CARTESIAN_POINT ( 'NONE',  ( 20.10937500061451289, -4.119189519843965641, -2.378215178125001383 ) ) ;
#54042=CARTESIAN_POINT ( 'NONE',  ( 22.53750000000000142, -2.886751345948125991, -5.000000000000000000 ) ) ;
#54044=CARTESIAN_POINT ( 'NONE',  ( 9.299999999999998934, 0.000000000000000000, 4.999999999999998224 ) ) ;
#54049=DIRECTION ( 'NONE',  ( 0.000000000000000000, 0.000000000000000000, 1.000000000000000000 ) ) ;
#54054=CARTESIAN_POINT ( 'NONE',  ( 7.893750001229032698, 5.773502691896255534, 3.535250795749688894E-16 ) ) ;
#54056=CARTESIAN_POINT ( 'NONE',  ( 16.88437500061451502, -2.746126346562641984, -4.756430356249999214 ) ) ;
#54065=CARTESIAN_POINT ( 'NONE',  ( 8.596875000614515372, 0.000000000000000000, 4.756430356249998326 ) ) ;
#54076=CARTESIAN_POINT ( 'NONE',  ( 27.57187500061451502, -4.119189519843968306, 2.378215178124996054 ) ) ;
#54080=CARTESIAN_POINT ( 'NONE',  ( 25.70625000122903003, -4.330127018922190985, -2.500000000000001332 ) ) ;
#54087=CARTESIAN_POINT ( 'NONE',  ( 27.30937500061451573, -4.119189519843965641, -2.378215178125001383 ) ) ;
#54089=CARTESIAN_POINT ( 'NONE',  ( 9.271875000614516082, -5.492252693125287522, -1.008910452111647106E-15 ) ) ;
#54092=ADVANCED_FACE ( 'NONE', ( #23592 ), #30595, .T. ) ;
#54105=CARTESIAN_POINT ( 'NONE',  ( 19.85625000122902861, -4.330127018922190985, -2.500000000000001332 ) ) ;
#54107=CARTESIAN_POINT ( 'NONE',  ( 23.69999999999999929, 0.000000000000000000, 4.999999999999998224 ) ) ;
#54121=CARTESIAN_POINT ( 'NONE',  ( 27.23437500061451644, -4.119189519843968306, 2.378215178124996054 ) ) ;
#54157=CARTESIAN_POINT ( 'NONE',  ( 16.47187500061451715, 5.824947211148865298E-16, -4.756430356249998326 ) ) ;
#54170=CARTESIAN_POINT ( 'NONE',  ( 16.46249999999999858, 2.886751345948126879, 4.999999999999998224 ) ) ;
#54171=CARTESIAN_POINT ( 'NONE',  ( 14.24999999999999822, 0.000000000000000000, 4.999999999999998224 ) ) ;
#54175=CARTESIAN_POINT ( 'NONE',  ( 16.88437500061451502, -4.119189519843968306, 2.378215178124996054 ) ) ;
#54186=CARTESIAN_POINT ( 'NONE',  ( 45.00000000000000000, 0.000000000000000000, 0.000000000000000000 ) ) ;
#54193=CARTESIAN_POINT ( 'NONE',  ( 29.30625000122903145, -4.330127018922190985, -2.500000000000001332 ) ) ;
#54217=CARTESIAN_POINT ( 'NONE',  ( 28.72500000000000142, -4.330127018922194537, 2.499999999999995559 ) ) ;
#54219=DIRECTION ( 'NONE',  ( 0.000000000000000000, 0.000000000000000000, 1.000000000000000000 ) ) ;
#54228=CARTESIAN_POINT ( 'NONE',  ( 27.54375000122902506, -2.886751345948112224, -5.000000000000023981 ) ) ;
#54236=CARTESIAN_POINT ( 'NONE',  ( 12.04687500061451821, 4.119189519843966529, -2.378215178124998275 ) ) ;
#54240=CARTESIAN_POINT ( 'NONE',  ( 22.88437500061451502, 5.492252693125287522, 3.363034840372157021E-16 ) ) ;
#54250=CARTESIAN_POINT ( 'NONE',  ( 14.17500000000000071, 4.330127018922191873, 2.499999999999999556 ) ) ;
#54258=CARTESIAN_POINT ( 'NONE',  ( 24.94687500061451502, -2.746126346562646425, 4.756430356249996549 ) ) ;
#54261=CARTESIAN_POINT ( 'NONE',  ( 13.21875000122903288, 2.886751345948129099, -4.999999999999997335 ) ) ;
#54265=EDGE_CURVE ( 'NONE', #68363, #67338, #26155, .T. ) ;
#54270=CARTESIAN_POINT ( 'NONE',  ( 25.18125000122903145, -4.330127018922194537, 2.499999999999995559 ) ) ;
#54281=CARTESIAN_POINT ( 'NONE',  ( 8.746875000614515727, -2.746126346562646425, 4.756430356249996549 ) ) ;
#54299=FACE_OUTER_BOUND ( 'NONE', #49206, .T. ) ;
#54310=UNCERTAINTY_MEASURE_WITH_UNIT (LENGTH_MEASURE( 1.000000000000000082E-05 ), #71243, 'distance_accuracy_value', 'NONE');
#54311=CARTESIAN_POINT ( 'NONE',  ( 14.93437500061451750, 4.119189519843966529, 2.378215178124999607 ) ) ;
#54320=CARTESIAN_POINT ( 'NONE',  ( 16.05000000000000071, 0.000000000000000000, 4.999999999999998224 ) ) ;
#54323=CARTESIAN_POINT ( 'NONE',  ( 24.82499999999999929, 6.123233995736764310E-16, -4.999999999999998224 ) ) ;
#54332=CARTESIAN_POINT ( 'NONE',  ( 23.25937500061451502, 2.746126346562645981, -4.756430356249997438 ) ) ;
#54342=CARTESIAN_POINT ( 'NONE',  ( 8.718750001229031099, 2.886751345948073588, -5.000000000000094147 ) ) ;
#54344=CARTESIAN_POINT ( 'NONE',  ( 10.24687500061451395, 4.119189519843966529, -2.378215178124998275 ) ) ;
#54355=ORIENTED_EDGE ( 'NONE', *, *, #51734, .T. ) ;
#54366=CARTESIAN_POINT ( 'NONE',  ( 16.09687500061451715, -2.746126346562641984, -4.756430356249999214 ) ) ;
#54378=ORIENTED_EDGE ( 'NONE', *, *, #43656, .T. ) ;
#54396=CARTESIAN_POINT ( 'NONE',  ( 21.98437500061451644, 5.824947211148865298E-16, -4.756430356249998326 ) ) ;
#54402=CARTESIAN_POINT ( 'NONE',  ( 21.11249999999999716, -5.773502691896255534, -1.060575238724906372E-15 ) ) ;
#54413=CARTESIAN_POINT ( 'NONE',  ( 7.593750001229034652, -2.886751345948129988, 4.999999999999997335 ) ) ;
#54415=CARTESIAN_POINT ( 'NONE',  ( 15.12187500061451573, 5.824947211148865298E-16, -4.756430356249998326 ) ) ;
#54422=CARTESIAN_POINT ( 'NONE',  ( 26.09999999999999787, -4.330127018922190985, -2.500000000000001332 ) ) ;
#54425=CARTESIAN_POINT ( 'NONE',  ( 28.64999999999999858, 0.000000000000000000, 4.999999999999998224 ) ) ;
#54426=CARTESIAN_POINT ( 'NONE',  ( 9.046875000614514661, 0.000000000000000000, 4.756430356249998326 ) ) ;
#54427=AXIS2_PLACEMENT_3D ( 'NONE', #57886, #69716, #53824 ) ;
#54428=ORIENTED_EDGE ( 'NONE', *, *, #27670, .T. ) ;
#54432=VERTEX_POINT ( 'NONE', #54590 ) ;
#54439=ORIENTED_EDGE ( 'NONE', *, *, #51854, .F. ) ;
#54449=CARTESIAN_POINT ( 'NONE',  ( 27.27187500061451431, -5.492252693125287522, -1.008910452111647106E-15 ) ) ;
#54451=CYLINDRICAL_SURFACE ( 'NONE', #38600, 4.999999999999998224 ) ;
#54460=FACE_OUTER_BOUND ( 'NONE', #11172, .T. ) ;
#54468=CARTESIAN_POINT ( 'NONE',  ( 18.50625000122903430, -4.330127018922190985, -2.500000000000001332 ) ) ;
#54471=ORIENTED_EDGE ( 'NONE', *, *, #43566, .F. ) ;
#54483=CARTESIAN_POINT ( 'NONE',  ( 29.40937500061451715, 0.000000000000000000, 4.756430356249998326 ) ) ;
#54505=DIRECTION ( 'NONE',  ( -1.000000000000000000, -0.000000000000000000, -0.000000000000000000 ) ) ;
#54518=CARTESIAN_POINT ( 'NONE',  ( 13.54687500061451466, 0.000000000000000000, 4.756430356249998326 ) ) ;
#54538=CARTESIAN_POINT ( 'NONE',  ( 16.20937500061451786, 4.119189519843966529, -2.378215178124998275 ) ) ;
#54548=CARTESIAN_POINT ( 'NONE',  ( 13.01249999999999929, -5.773502691896255534, -1.060575238724906372E-15 ) ) ;
#54555=CARTESIAN_POINT ( 'NONE',  ( 27.80625000122903145, 0.000000000000000000, 4.999999999999998224 ) ) ;
#54557=CARTESIAN_POINT ( 'NONE',  ( 26.83125000122903003, 4.330127018922191873, 2.499999999999999556 ) ) ;
#54566=ORIENTED_EDGE ( 'NONE', *, *, #53564, .F. ) ;
#54579=CARTESIAN_POINT ( 'NONE',  ( 26.73749999999999716, 5.773502691896255534, 3.535250795749688894E-16 ) ) ;
#54581=CARTESIAN_POINT ( 'NONE',  ( 26.56875000122903074, -5.773502691896255534, -1.060575238724906372E-15 ) ) ;
#54590=CARTESIAN_POINT ( 'NONE',  ( 12.90000000000000213, 0.000000000000000000, 4.999999999999998224 ) ) ;
#54602=CARTESIAN_POINT ( 'NONE',  ( 22.17187500061451644, -4.119189519843968306, 2.378215178124996054 ) ) ;
#54610=CARTESIAN_POINT ( 'NONE',  ( 13.16249999999999964, 2.886751345948129099, -4.999999999999998224 ) ) ;
#54617=CARTESIAN_POINT ( 'NONE',  ( 24.08437500061451786, -4.119189519843968306, 2.378215178124996054 ) ) ;
#54627=CARTESIAN_POINT ( 'NONE',  ( -4.999999999999996447, -2.928932188134524051, -4.999999999999996447 ) ) ;
#54628=ORIENTED_EDGE ( 'NONE', *, *, #59386, .F. ) ;
#54635=EDGE_CURVE ( 'NONE', #6912, #48096, #11057, .T. ) ;
#54639=CARTESIAN_POINT ( 'NONE',  ( 10.62187500061451750, -5.492252693125287522, -1.008910452111647106E-15 ) ) ;
#54650=CARTESIAN_POINT ( 'NONE',  ( 23.38125000122903074, -4.330127018922194537, 2.499999999999995559 ) ) ;
#54666=CARTESIAN_POINT ( 'NONE',  ( 12.60937500061451821, 4.119189519843966529, -2.378215178124998275 ) ) ;
#54677=CARTESIAN_POINT ( 'NONE',  ( 14.24999999999999822, 0.000000000000000000, 4.999999999999998224 ) ) ;
#54681=DIRECTION ( 'NONE',  ( -1.000000000000000000, -0.000000000000000000, -0.000000000000000000 ) ) ;
#54682=( BOUNDED_CURVE ( )  B_SPLINE_CURVE ( 2, ( #32977, #49976, #20047, #65128, #8989, #31521, #457 ),
 .UNSPECIFIED., .F., .F. ) 
 B_SPLINE_CURVE_WITH_KNOTS ( ( 3, 2, 2, 3 ),
 ( 0.5499999999999999334, 0.5533333333333332327, 0.5566666666666666430, 0.5600000000000000533 ),
 .UNSPECIFIED. ) 
 CURVE ( )  GEOMETRIC_REPRESENTATION_ITEM ( )  RATIONAL_B_SPLINE_CURVE ( ( 1.000000000000004441, 0.8660254037844342667, 1.000000000000000000, 0.8660254037844387076, 1.000000000000000000, 0.8660254037844387076, 1.000000000000000000 ) ) 
 REPRESENTATION_ITEM ( '' )  );
#54688=CARTESIAN_POINT ( 'NONE',  ( 19.95937500061451786, -5.492252693125287522, -1.008910452111647106E-15 ) ) ;
#54704=CARTESIAN_POINT ( 'NONE',  ( 9.159375000614517148, -5.492252693125287522, -1.008910452111647106E-15 ) ) ;
#54709=( BOUNDED_CURVE ( )  B_SPLINE_CURVE ( 2, ( #65790, #60230, #9644, #29181, #72798, #17708, #67982 ),
 .UNSPECIFIED., .F., .F. ) 
 B_SPLINE_CURVE_WITH_KNOTS ( ( 3, 2, 2, 3 ),
 ( 0.6800000000000001599, 0.6833333333333334592, 0.6866666666666667584, 0.6900000000000000577 ),
 .UNSPECIFIED. ) 
 CURVE ( )  GEOMETRIC_REPRESENTATION_ITEM ( )  RATIONAL_B_SPLINE_CURVE ( ( 0.9999999999999955591, 0.8660254037844431485, 1.000000000000000000, 0.8660254037844387076, 1.000000000000000000, 0.8660254037844342667, 1.000000000000004441 ) ) 
 REPRESENTATION_ITEM ( '' )  );
#54727=CARTESIAN_POINT ( 'NONE',  ( 15.94687500061451502, -2.746126346562646425, 4.756430356249996549 ) ) ;
#54731=ORIENTED_EDGE ( 'NONE', *, *, #49427, .T. ) ;
#54758=CARTESIAN_POINT ( 'NONE',  ( 20.63437500061451857, 5.824947211148865298E-16, -4.756430356249998326 ) ) ;
#54765=CARTESIAN_POINT ( 'NONE',  ( 22.42500000000000071, -4.330127018922194537, 2.499999999999995559 ) ) ;
#54769=CARTESIAN_POINT ( 'NONE',  ( 28.35000000000000142, -4.330127018922190985, -2.500000000000001332 ) ) ;
#54774=CARTESIAN_POINT ( 'NONE',  ( 27.68437500061451573, -2.746126346562642428, -4.756430356249999214 ) ) ;
#54776=CARTESIAN_POINT ( 'NONE',  ( 14.03437500061451537, -2.746126346562646425, 4.756430356249996549 ) ) ;
#54786=CARTESIAN_POINT ( 'NONE',  ( 7.809375000614515727, -5.492252693125287522, -1.008910452111647106E-15 ) ) ;
#54798=AXIS2_PLACEMENT_3D ( 'NONE', #2417, #63385, #12770 ) ;
#54803=DIRECTION ( 'NONE',  ( -1.000000000000000000, -0.000000000000000000, -0.000000000000000000 ) ) ;
#54810=CARTESIAN_POINT ( 'NONE',  ( 23.33437500061451786, 5.824947211148865298E-16, -4.756430356249998326 ) ) ;
#54812=CARTESIAN_POINT ( 'NONE',  ( 8.709375000614517859, 0.000000000000000000, 4.756430356249998326 ) ) ;
#54821=CARTESIAN_POINT ( 'NONE',  ( 17.38125000122903074, 4.330127018922191873, 2.499999999999999556 ) ) ;
#54830=CARTESIAN_POINT ( 'NONE',  ( 17.45625000122903003, 0.000000000000000000, 4.999999999999998224 ) ) ;
#54838=LINE ( 'NONE', #15301, #60374 ) ;
#54845=CARTESIAN_POINT ( 'NONE',  ( 28.73437500061451644, 5.824947211148865298E-16, -4.756430356249998326 ) ) ;
#54852=VECTOR ( 'NONE', #17993, 1000.000000000000000 ) ;
#54854=CARTESIAN_POINT ( 'NONE',  ( 25.01249999999999929, 2.886751345948126879, 4.999999999999998224 ) ) ;
#54863=CARTESIAN_POINT ( 'NONE',  ( 27.97500000000000142, 6.123233995736764310E-16, -4.999999999999998224 ) ) ;
#54865=CARTESIAN_POINT ( 'NONE',  ( 21.98437500061451644, 5.492252693125287522, 3.363034840372157021E-16 ) ) ;
#54877=ORIENTED_EDGE ( 'NONE', *, *, #65091, .T. ) ;
#54880=VERTEX_POINT ( 'NONE', #62310 ) ;
#54884=CARTESIAN_POINT ( 'NONE',  ( 13.77187500061451431, 5.824947211148865298E-16, -4.756430356249998326 ) ) ;
#54901=CYLINDRICAL_SURFACE ( 'NONE', #18232, 5.000000000000000000 ) ;
#54902=CARTESIAN_POINT ( 'NONE',  ( 15.49687500061451750, -2.746126346562646425, 4.756430356249996549 ) ) ;
#54917=CARTESIAN_POINT ( 'NONE',  ( 25.57499999999999929, -4.330127018922194537, 2.499999999999995559 ) ) ;
#54921=CARTESIAN_POINT ( 'NONE',  ( 26.86875000122903145, 2.886751345948126879, 4.999999999999999112 ) ) ;
#54927=( BOUNDED_CURVE ( )  B_SPLINE_CURVE ( 2, ( #29416, #18667, #24221, #45691, #63741, #29770, #34583 ),
 .UNSPECIFIED., .F., .F. ) 
 B_SPLINE_CURVE_WITH_KNOTS ( ( 3, 2, 2, 3 ),
 ( 0.2700000000000000733, 0.2733333333333333726, 0.2766666666666666718, 0.2800000000000000266 ),
 .UNSPECIFIED. ) 
 CURVE ( )  GEOMETRIC_REPRESENTATION_ITEM ( )  RATIONAL_B_SPLINE_CURVE ( ( 0.9999999999999977796, 0.8660254037844409281, 1.000000000000000000, 0.8660254037844387076, 1.000000000000000000, 0.8660254037844387076, 1.000000000000000000 ) ) 
 REPRESENTATION_ITEM ( '' )  );
#54935=CARTESIAN_POINT ( 'NONE',  ( 13.74375000122903323, 5.773502691896255534, 3.535250795749688401E-16 ) ) ;
#54964=ORIENTED_EDGE ( 'NONE', *, *, #45125, .T. ) ;
#54970=CARTESIAN_POINT ( 'NONE',  ( 20.93437500061451217, -2.746126346562642428, -4.756430356249999214 ) ) ;
#54979=VERTEX_POINT ( 'NONE', #29774 ) ;
#54980=CARTESIAN_POINT ( 'NONE',  ( 13.95000000000000107, -4.330127018922190985, -2.500000000000001332 ) ) ;
#54987=CARTESIAN_POINT ( 'NONE',  ( 21.87187500061451573, -5.492252693125287522, -1.008910452111647106E-15 ) ) ;
#55009=CARTESIAN_POINT ( 'NONE',  ( 10.32187500061451679, 2.746126346562645981, -4.756430356249997438 ) ) ;
#55023=CARTESIAN_POINT ( 'NONE',  ( 14.90625000122903110, -4.330127018922190985, -2.500000000000001332 ) ) ;
#55035=CARTESIAN_POINT ( 'NONE',  ( 11.44687500061451857, -2.746126346562646425, 4.756430356249996549 ) ) ;
#55038=CARTESIAN_POINT ( 'NONE',  ( 13.63125000122903252, 6.123233995736764310E-16, -4.999999999999998224 ) ) ;
#55047=CYLINDRICAL_SURFACE ( 'NONE', #40685, 4.999999999999998224 ) ;
#55050=EDGE_CURVE ( 'NONE', #1482, #59687, #5881, .T. ) ;
#55052=CARTESIAN_POINT ( 'NONE',  ( 19.61249999999999716, 2.886751345948126879, 4.999999999999998224 ) ) ;
#55057=CARTESIAN_POINT ( 'NONE',  ( 19.24687500061451573, 4.119189519843966529, -2.378215178124998275 ) ) ;
#55060=CARTESIAN_POINT ( 'NONE',  ( 14.08125000122903181, 6.123233995736764310E-16, -4.999999999999998224 ) ) ;
#55074=CARTESIAN_POINT ( 'NONE',  ( 28.62187500061451573, -5.492252693125287522, -1.008910452111647106E-15 ) ) ;
#55084=ORIENTED_EDGE ( 'NONE', *, *, #2651, .T. ) ;
#55095=EDGE_CURVE ( 'NONE', #31243, #1482, #5450, .T. ) ;
#55097=CARTESIAN_POINT ( 'NONE',  ( 17.14687500061451786, 5.492252693125287522, 3.363034840372157021E-16 ) ) ;
#55125=CARTESIAN_POINT ( 'NONE',  ( 14.28749999999999787, -2.886751345948019409, 5.000000000000189182 ) ) ;
#55127=ORIENTED_EDGE ( 'NONE', *, *, #14279, .T. ) ;
#55130=CARTESIAN_POINT ( 'NONE',  ( 19.58437500061451786, -4.119189519843968306, 2.378215178124996054 ) ) ;
#55137=CARTESIAN_POINT ( 'NONE',  ( 20.02500000000000213, 4.330127018922191873, 2.499999999999999556 ) ) ;
#55139=CARTESIAN_POINT ( 'NONE',  ( 18.84375000122903643, -2.886751345948157965, 4.999999999999948486 ) ) ;
#55141=CARTESIAN_POINT ( 'NONE',  ( 17.23125000122903572, 6.123233995736764310E-16, -4.999999999999998224 ) ) ;
#55142=CARTESIAN_POINT ( 'NONE',  ( 24.33749999999999858, -2.886751345948112224, -5.000000000000023981 ) ) ;
#55146=CARTESIAN_POINT ( 'NONE',  ( 26.40937500061451360, 2.746126346562645981, -4.756430356249997438 ) ) ;
#55148=CARTESIAN_POINT ( 'NONE',  ( 13.47187500061451715, 4.119189519843966529, 2.378215178124999607 ) ) ;
#55155=EDGE_CURVE ( 'NONE', #19407, #27917, #12981, .T. ) ;
#55179=EDGE_CURVE ( 'NONE', #44765, #63037, #25734, .T. ) ;
#55183=CARTESIAN_POINT ( 'NONE',  ( 25.50937500061451502, -4.119189519843965641, -2.378215178125001383 ) ) ;
#55185=CARTESIAN_POINT ( 'NONE',  ( 7.771875000614516971, 2.746126346562643317, 4.756430356249998326 ) ) ;
#55204=CARTESIAN_POINT ( 'NONE',  ( 19.25625000122903430, 0.000000000000000000, 4.999999999999998224 ) ) ;
#55206=CARTESIAN_POINT ( 'NONE',  ( 29.45625000122903003, 4.330127018922192761, -2.499999999999997780 ) ) ;
#55219=CARTESIAN_POINT ( 'NONE',  ( 25.69687500061451502, 5.492252693125287522, 3.363034840372157021E-16 ) ) ;
#55222=AXIS2_PLACEMENT_3D ( 'NONE', #16573, #61640, #43945 ) ;
#55234=CARTESIAN_POINT ( 'NONE',  ( 11.38125000122903252, 6.123233995736764310E-16, -4.999999999999998224 ) ) ;
#55235=CARTESIAN_POINT ( 'NONE',  ( 7.950000000000001954, 0.000000000000000000, 4.999999999999998224 ) ) ;
#55238=CARTESIAN_POINT ( 'NONE',  ( 20.52187500061451786, 5.824947211148865298E-16, -4.756430356249998326 ) ) ;
#55241=ORIENTED_EDGE ( 'NONE', *, *, #16377, .T. ) ;
#55256=CARTESIAN_POINT ( 'NONE',  ( 15.04687500061451466, -4.119189519843965641, -2.378215178125001383 ) ) ;
#55272=CARTESIAN_POINT ( 'NONE',  ( 29.25937500061451502, 2.746126346562643317, 4.756430356249998326 ) ) ;
#55273=CARTESIAN_POINT ( 'NONE',  ( 16.39687500061451786, -2.746126346562646425, 4.756430356249996549 ) ) ;
#55291=CARTESIAN_POINT ( 'NONE',  ( 26.94375000122903074, -2.886751345948129988, 4.999999999999997335 ) ) ;
#55303=CARTESIAN_POINT ( 'NONE',  ( 10.40625000122903288, -4.330127018922190985, -2.500000000000001332 ) ) ;
#55319=CARTESIAN_POINT ( 'NONE',  ( 12.56250000000000000, -5.773502691896255534, -1.060575238724906372E-15 ) ) ;
#55337=CARTESIAN_POINT ( 'NONE',  ( 21.79687500061451644, -4.119189519843965641, -2.378215178125001383 ) ) ;
#55340=LINE ( 'NONE', #27269, #52728 ) ;
#55345=CARTESIAN_POINT ( 'NONE',  ( 26.69999999999999929, 4.330127018922192761, -2.499999999999997780 ) ) ;
#55347=CARTESIAN_POINT ( 'NONE',  ( 11.13750000000000284, -2.886751345948129988, 4.999999999999997335 ) ) ;
#55354=CARTESIAN_POINT ( 'NONE',  ( 22.35937500061451644, -4.119189519843965641, -2.378215178125001383 ) ) ;
#55362=( BOUNDED_CURVE ( )  B_SPLINE_CURVE ( 2, ( #62527, #29280, #11571, #11924, #51091, #51810, #67722 ),
 .UNSPECIFIED., .F., .F. ) 
 B_SPLINE_CURVE_WITH_KNOTS ( ( 3, 2, 2, 3 ),
 ( 0.2000000000000000389, 0.2033333333333333659, 0.2066666666666667207, 0.2100000000000000477 ),
 .UNSPECIFIED. ) 
 CURVE ( )  GEOMETRIC_REPRESENTATION_ITEM ( )  RATIONAL_B_SPLINE_CURVE ( ( 0.9999999999999988898, 0.8660254037844398178, 1.000000000000000000, 0.8660254037844387076, 1.000000000000000000, 0.8660254037844364872, 1.000000000000002220 ) ) 
 REPRESENTATION_ITEM ( '' )  );
#55366=VERTEX_POINT ( 'NONE', #54863 ) ;
#55372=CARTESIAN_POINT ( 'NONE',  ( 18.41249999999999787, -5.773502691896255534, -1.060575238724906372E-15 ) ) ;
#55376=CARTESIAN_POINT ( 'NONE',  ( 9.646875000614519635, -2.746126346562646425, 4.756430356249996549 ) ) ;
#55398=CARTESIAN_POINT ( 'NONE',  ( 11.03437500061451715, -4.119189519843968306, 2.378215178124996054 ) ) ;
#55404=EDGE_CURVE ( 'NONE', #58120, #4995, #43071, .T. ) ;
#55421=CARTESIAN_POINT ( 'NONE',  ( 19.17187500061451289, 5.824947211148865298E-16, -4.756430356249998326 ) ) ;
#55424=CARTESIAN_POINT ( 'NONE',  ( 13.40625000122903288, 0.000000000000000000, 4.999999999999998224 ) ) ;
#55439=CARTESIAN_POINT ( 'NONE',  ( 7.846875000614515372, -4.119189519843965641, -2.378215178125001383 ) ) ;
#55460=CARTESIAN_POINT ( 'NONE',  ( 17.37187500061451573, -5.492252693125287522, -1.008910452111647106E-15 ) ) ;
#55490=CARTESIAN_POINT ( 'NONE',  ( 18.12187500061451573, 2.746126346562643317, 4.756430356249998326 ) ) ;
#55496=CARTESIAN_POINT ( 'NONE',  ( 20.58750000000000213, -2.886751345948129988, 4.999999999999997335 ) ) ;
#55499=DIRECTION ( 'NONE',  ( 0.000000000000000000, 0.000000000000000000, 1.000000000000000000 ) ) ;
#55502=CARTESIAN_POINT ( 'NONE',  ( 24.26249999999999929, -5.773502691896255534, -1.060575238724906372E-15 ) ) ;
#55509=CARTESIAN_POINT ( 'NONE',  ( 28.43437500061451573, -2.746126346562646425, 4.756430356249996549 ) ) ;
#55511=CARTESIAN_POINT ( 'NONE',  ( 14.44687500061451502, 0.000000000000000000, 4.756430356249998326 ) ) ;
#55517=CYLINDRICAL_SURFACE ( 'NONE', #30185, 4.999999999999998224 ) ;
#55520=DIRECTION ( 'NONE',  ( -1.000000000000000000, -0.000000000000000000, -0.000000000000000000 ) ) ;
#55543=CARTESIAN_POINT ( 'NONE',  ( 25.13437500061451502, 5.824947211148865298E-16, -4.756430356249998326 ) ) ;
#55545=CARTESIAN_POINT ( 'NONE',  ( 7.959375000614516971, -4.119189519843965641, -2.378215178125001383 ) ) ;
#55562=CARTESIAN_POINT ( 'NONE',  ( 19.36875000122903501, -5.773502691896255534, -1.060575238724906372E-15 ) ) ;
#55564=LINE ( 'NONE', #509, #32546 ) ;
#55580=CARTESIAN_POINT ( 'NONE',  ( 25.92187500061451999, -5.492252693125287522, -1.008910452111647106E-15 ) ) ;
#55593=CARTESIAN_POINT ( 'NONE',  ( 11.26875000122903003, -5.773502691896255534, -1.060575238724906372E-15 ) ) ;
#55597=CARTESIAN_POINT ( 'NONE',  ( 19.73437500061451289, 5.492252693125287522, 3.363034840372157021E-16 ) ) ;
#55607=CARTESIAN_POINT ( 'NONE',  ( 11.82187500061451502, -4.119189519843968306, 2.378215178124996054 ) ) ;
#55616=CARTESIAN_POINT ( 'NONE',  ( 13.80937500061451395, 2.746126346562645981, -4.756430356249997438 ) ) ;
#55619=CARTESIAN_POINT ( 'NONE',  ( 45.00000000000000000, 0.000000000000000000, 0.000000000000000000 ) ) ;
#55632=CARTESIAN_POINT ( 'NONE',  ( 8.568750001229034297, -5.773502691896255534, -1.060575238724906372E-15 ) ) ;
#55633=CARTESIAN_POINT ( 'NONE',  ( 15.90937500061451892, 0.000000000000000000, 4.756430356249998326 ) ) ;
#55641=DIRECTION ( 'NONE',  ( -0.000000000000000000, 6.195440985631455317E-17, 1.000000000000000000 ) ) ;
#55650=CARTESIAN_POINT ( 'NONE',  ( 25.81875000122903074, 2.886751345948129099, -4.999999999999998224 ) ) ;
#55660=ORIENTED_EDGE ( 'NONE', *, *, #41079, .F. ) ;
#55662=CYLINDRICAL_SURFACE ( 'NONE', #47977, 4.999999999999998224 ) ;
#55670=EDGE_CURVE ( 'NONE', #8461, #17653, #40851, .T. ) ;
#55689=CARTESIAN_POINT ( 'NONE',  ( 45.00000000000000000, 0.000000000000000000, 4.999999999999998224 ) ) ;
#55693=EDGE_CURVE ( 'NONE', #7820, #53311, #42088, .T. ) ;
#55696=AXIS2_PLACEMENT_3D ( 'NONE', #25196, #3045, #13754 ) ;
#55699=CARTESIAN_POINT ( 'NONE',  ( 20.59687500061451715, 4.119189519843966529, -2.378215178124998275 ) ) ;
#55706=CARTESIAN_POINT ( 'NONE',  ( 9.525000000000002132, 6.123233995736764310E-16, -4.999999999999998224 ) ) ;
#55708=CARTESIAN_POINT ( 'NONE',  ( 9.862500000000000711, -5.773502691896255534, -1.060575238724906372E-15 ) ) ;
#55715=CARTESIAN_POINT ( 'NONE',  ( 22.47187500061451715, 2.746126346562645981, -4.756430356249997438 ) ) ;
#55731=CARTESIAN_POINT ( 'NONE',  ( 27.20625000122903359, 4.330127018922192761, -2.499999999999997780 ) ) ;
#55738=CARTESIAN_POINT ( 'NONE',  ( 9.946875000614516793, 5.492252693125287522, 3.363034840372157021E-16 ) ) ;
#55760=CARTESIAN_POINT ( 'NONE',  ( 12.04687500061451821, -2.746126346562642428, -4.756430356249999214 ) ) ;
#55761=LINE ( 'NONE', #49861, #8765 ) ;
#55773=DIRECTION ( 'NONE',  ( -1.000000000000000000, -0.000000000000000000, -0.000000000000000000 ) ) ;
#55783=CARTESIAN_POINT ( 'NONE',  ( 20.48437500061451644, -2.746126346562642428, -4.756430356249999214 ) ) ;
#55786=CARTESIAN_POINT ( 'NONE',  ( 13.36875000122903145, 2.886751345948126879, 4.999999999999999112 ) ) ;
#55801=CARTESIAN_POINT ( 'NONE',  ( 29.78437500061451715, 4.119189519843966529, 2.378215178124999607 ) ) ;
#55811=ORIENTED_EDGE ( 'NONE', *, *, #44062, .F. ) ;
#55822=CARTESIAN_POINT ( 'NONE',  ( 16.35937500061451644, 0.000000000000000000, 4.756430356249998326 ) ) ;
#55854=CARTESIAN_POINT ( 'NONE',  ( 18.94687500061451502, 5.492252693125287522, 3.363034840372157021E-16 ) ) ;
#55856=CARTESIAN_POINT ( 'NONE',  ( 45.00000000000000000, 0.000000000000000000, 0.000000000000000000 ) ) ;
#55860=CARTESIAN_POINT ( 'NONE',  ( 20.54999999999999716, 0.000000000000000000, 4.999999999999998224 ) ) ;
#55864=CARTESIAN_POINT ( 'NONE',  ( 25.17187500061451644, 4.119189519843966529, 2.378215178124999607 ) ) ;
#55865=CARTESIAN_POINT ( 'NONE',  ( 14.49375000122903145, -2.886751345948126435, -5.000000000000000000 ) ) ;
#55872=CARTESIAN_POINT ( 'NONE',  ( 26.55937500061451217, 2.746126346562643317, 4.756430356249998326 ) ) ;
#55874=CARTESIAN_POINT ( 'NONE',  ( 13.54687500061451466, 0.000000000000000000, 4.756430356249998326 ) ) ;
#55896=ORIENTED_EDGE ( 'NONE', *, *, #5848, .F. ) ;
#55905=CARTESIAN_POINT ( 'NONE',  ( 25.32187500061451857, 2.746126346562643317, 4.756430356249998326 ) ) ;
#55916=CARTESIAN_POINT ( 'NONE',  ( 7.668750001229033053, -5.773502691896255534, -1.060575238724906372E-15 ) ) ;
#55923=CARTESIAN_POINT ( 'NONE',  ( 17.71875000122903288, 2.886751345948129099, -4.999999999999998224 ) ) ;
#55926=VERTEX_POINT ( 'NONE', #11619 ) ;
#55940=CARTESIAN_POINT ( 'NONE',  ( 25.05937500061451573, -4.119189519843965641, -2.378215178125001383 ) ) ;
#55946=CARTESIAN_POINT ( 'NONE',  ( 27.86249999999999716, -5.773502691896255534, -1.060575238724906372E-15 ) ) ;
#55954=CARTESIAN_POINT ( 'NONE',  ( 11.04375000122903216, 5.773502691896255534, 3.535250795749688894E-16 ) ) ;
#55958=CARTESIAN_POINT ( 'NONE',  ( 19.80937500061451217, 2.746126346562643317, 4.756430356249998326 ) ) ;
#55959=AXIS2_PLACEMENT_3D ( 'NONE', #40943, #63457, #18012 ) ;
#55971=CARTESIAN_POINT ( 'NONE',  ( 11.70937500061451608, 2.746126346562643317, 4.756430356249998326 ) ) ;
#55977=EDGE_LOOP ( 'NONE', ( #32331, #49561, #54877, #34882 ) ) ;
#55986=VERTEX_POINT ( 'NONE', #49137 ) ;
#55995=CARTESIAN_POINT ( 'NONE',  ( 8.531250001229034652, -4.330127018922194537, 2.499999999999995559 ) ) ;
#55996=CARTESIAN_POINT ( 'NONE',  ( 15.42187500061451821, 2.746126346562643317, 4.756430356249998326 ) ) ;
#56005=( BOUNDED_CURVE ( )  B_SPLINE_CURVE ( 2, ( #57491, #69673, #51962, #53407, #23509, #68592, #1361 ),
 .UNSPECIFIED., .F., .F. ) 
 B_SPLINE_CURVE_WITH_KNOTS ( ( 3, 2, 2, 3 ),
 ( 0.8300000000000000711, 0.8333333333333334814, 0.8366666666666666696, 0.8399999999999999689 ),
 .UNSPECIFIED. ) 
 CURVE ( )  GEOMETRIC_REPRESENTATION_ITEM ( )  RATIONAL_B_SPLINE_CURVE ( ( 0.9999999999999955591, 0.8660254037844431485, 1.000000000000000000, 0.8660254037844387076, 1.000000000000000000, 0.8660254037844387076, 1.000000000000000000 ) ) 
 REPRESENTATION_ITEM ( '' )  );
#56015=CARTESIAN_POINT ( 'NONE',  ( 24.76875000122903003, -5.773502691896255534, -1.060575238724906372E-15 ) ) ;
#56017=LINE ( 'NONE', #29027, #30157 ) ;
#56020=EDGE_CURVE ( 'NONE', #6086, #69242, #20533, .T. ) ;
#56021=CARTESIAN_POINT ( 'NONE',  ( -4.999999999999998224, -2.928932188134522718, 4.999999999999998224 ) ) ;
#56029=CARTESIAN_POINT ( 'NONE',  ( 13.85625000122903216, 0.000000000000000000, 4.999999999999998224 ) ) ;
#56039=VECTOR ( 'NONE', #62481, 1000.000000000000000 ) ;
#56048=CARTESIAN_POINT ( 'NONE',  ( 26.15625000122903288, -4.330127018922190985, -2.500000000000001332 ) ) ;
#56062=CARTESIAN_POINT ( 'NONE',  ( 21.57187500061451146, 4.119189519843966529, 2.378215178124999607 ) ) ;
#56074=CARTESIAN_POINT ( 'NONE',  ( 10.65000000000000036, 0.000000000000000000, 4.999999999999998224 ) ) ;
#56075=VECTOR ( 'NONE', #14895, 1000.000000000000000 ) ;
#56081=CARTESIAN_POINT ( 'NONE',  ( 45.00000000000000000, 0.000000000000000000, 0.000000000000000000 ) ) ;
#56082=CARTESIAN_POINT ( 'NONE',  ( 23.33437500061451786, 5.824947211148865298E-16, -4.756430356249998326 ) ) ;
#56085=CARTESIAN_POINT ( 'NONE',  ( 12.86250000000000071, 2.886751345948126879, 4.999999999999998224 ) ) ;
#56098=CARTESIAN_POINT ( 'NONE',  ( 27.24375000122903145, 5.773502691896255534, 3.535250795749688401E-16 ) ) ;
#56126=CARTESIAN_POINT ( 'NONE',  ( 12.75937500061451857, 0.000000000000000000, 4.756430356249998326 ) ) ;
#56127=FACE_OUTER_BOUND ( 'NONE', #34028, .T. ) ;
#56135=AXIS2_PLACEMENT_3D ( 'NONE', #47253, #36528, #52794 ) ;
#56138=FACE_OUTER_BOUND ( 'NONE', #17747, .T. ) ;
#56140=CARTESIAN_POINT ( 'NONE',  ( 29.09999999999999787, 0.000000000000000000, 4.999999999999998224 ) ) ;
#56145=CARTESIAN_POINT ( 'NONE',  ( 19.84687500061451360, 0.000000000000000000, 4.756430356249998326 ) ) ;
#56148=CARTESIAN_POINT ( 'NONE',  ( 15.16875000122903394, 2.886751345948126879, 4.999999999999999112 ) ) ;
#56152=CARTESIAN_POINT ( 'NONE',  ( 26.96249999999999858, -5.773502691896255534, -1.060575238724906372E-15 ) ) ;
#56163=CARTESIAN_POINT ( 'NONE',  ( 7.621875000614515727, 4.119189519843966529, 2.378215178124999607 ) ) ;
#56173=VECTOR ( 'NONE', #69192, 1000.000000000000000 ) ;
#56186=CARTESIAN_POINT ( 'NONE',  ( 15.49687500061451750, -2.746126346562646425, 4.756430356249996549 ) ) ;
#56194=ADVANCED_FACE ( 'NONE', ( #38035 ), #71665, .T. ) ;
#56219=CARTESIAN_POINT ( 'NONE',  ( 17.97187500061451715, 2.746126346562645981, -4.756430356249997438 ) ) ;
#56225=CARTESIAN_POINT ( 'NONE',  ( 18.93750000000000000, -2.886751345948125991, -5.000000000000000000 ) ) ;
#56229=CARTESIAN_POINT ( 'NONE',  ( 24.60937500061451644, 2.746126346562645981, -4.756430356249997438 ) ) ;
#56232=CARTESIAN_POINT ( 'NONE',  ( 17.55000000000000071, -4.330127018922190985, -2.500000000000001332 ) ) ;
#56236=CARTESIAN_POINT ( 'NONE',  ( 26.59687500061451360, 0.000000000000000000, 4.756430356249998326 ) ) ;
#56239=CARTESIAN_POINT ( 'NONE',  ( 13.24687500061451750, -4.119189519843965641, -2.378215178125001383 ) ) ;
#56240=EDGE_CURVE ( 'NONE', #26559, #72520, #55761, .T. ) ;
#56245=LINE ( 'NONE', #456, #64236 ) ;
#56276=CARTESIAN_POINT ( 'NONE',  ( 24.64687500061451431, -2.746126346562641984, -4.756430356249999214 ) ) ;
#56293=CARTESIAN_POINT ( 'NONE',  ( 16.63125000122903074, -4.330127018922194537, 2.499999999999995559 ) ) ;
#56295=CARTESIAN_POINT ( 'NONE',  ( 29.56875000122903074, 2.886751345948126879, 4.999999999999998224 ) ) ;
#56302=CARTESIAN_POINT ( 'NONE',  ( 10.68749999999999467, -2.886751345948019409, 5.000000000000189182 ) ) ;
#56308=CARTESIAN_POINT ( 'NONE',  ( 25.39687500061451431, -2.746126346562646425, 4.756430356249996549 ) ) ;
#56313=CARTESIAN_POINT ( 'NONE',  ( 27.44999999999999929, -4.330127018922190985, -2.500000000000001332 ) ) ;
#56322=CARTESIAN_POINT ( 'NONE',  ( 12.61875000122903323, -5.773502691896255534, -1.060575238724906372E-15 ) ) ;
#56326=CARTESIAN_POINT ( 'NONE',  ( 20.70937500061451786, 2.746126346562643317, 4.756430356249998326 ) ) ;
#56337=CARTESIAN_POINT ( 'NONE',  ( 12.53437500061451537, 5.492252693125287522, 3.363034840372157021E-16 ) ) ;
#56340=ADVANCED_FACE ( 'NONE', ( #56127 ), #73114, .T. ) ;
#56345=CARTESIAN_POINT ( 'NONE',  ( 45.00000000000000000, 0.000000000000000000, 4.999999999999998224 ) ) ;
#56347=CARTESIAN_POINT ( 'NONE',  ( 45.00000000000000000, 0.000000000000000000, 4.999999999999998224 ) ) ;
#56359=CARTESIAN_POINT ( 'NONE',  ( 17.02499999999999858, -4.330127018922194537, 2.499999999999995559 ) ) ;
#56361=CARTESIAN_POINT ( 'NONE',  ( 29.55937500061451217, 2.746126346562645981, -4.756430356249997438 ) ) ;
#56362=CARTESIAN_POINT ( 'NONE',  ( 13.88437500061451679, 5.824947211148865298E-16, -4.756430356249998326 ) ) ;
#56379=CARTESIAN_POINT ( 'NONE',  ( 26.23125000122903216, 6.123233995736764310E-16, -4.999999999999998224 ) ) ;
#56384=AXIS2_PLACEMENT_3D ( 'NONE', #57870, #64879, #46808 ) ;
#56387=( BOUNDED_CURVE ( )  B_SPLINE_CURVE ( 2, ( #32872, #70572, #26607, #15500, #49145, #14777, #4448 ),
 .UNSPECIFIED., .F., .F. ) 
 B_SPLINE_CURVE_WITH_KNOTS ( ( 3, 2, 2, 3 ),
 ( 0.5800000000000000711, 0.5833333333333334814, 0.5866666666666666696, 0.5899999999999999689 ),
 .UNSPECIFIED. ) 
 CURVE ( )  GEOMETRIC_REPRESENTATION_ITEM ( )  RATIONAL_B_SPLINE_CURVE ( ( 0.9999999999999955591, 0.8660254037844431485, 1.000000000000000000, 0.8660254037844387076, 1.000000000000000000, 0.8660254037844387076, 1.000000000000000000 ) ) 
 REPRESENTATION_ITEM ( '' )  );
#56415=CARTESIAN_POINT ( 'NONE',  ( 27.73125000122902861, 4.330127018922191873, 2.499999999999999556 ) ) ;
#56422=ORIENTED_EDGE ( 'NONE', *, *, #60445, .F. ) ;
#56425=CARTESIAN_POINT ( 'NONE',  ( 18.34687500061451360, 4.119189519843966529, -2.378215178124998275 ) ) ;
#56439=DIRECTION ( 'NONE',  ( 0.000000000000000000, 0.000000000000000000, 1.000000000000000000 ) ) ;
#56440=CARTESIAN_POINT ( 'NONE',  ( 23.07187500061451857, 2.746126346562643317, 4.756430356249998326 ) ) ;
#56457=LINE ( 'NONE', #5847, #53948 ) ;
#56462=CARTESIAN_POINT ( 'NONE',  ( 7.921875000614517326, -5.492252693125287522, -1.008910452111647106E-15 ) ) ;
#56470=VERTEX_POINT ( 'NONE', #23583 ) ;
#56482=CARTESIAN_POINT ( 'NONE',  ( 9.609375000614518214, 0.000000000000000000, 4.756430356249998326 ) ) ;
#56483=DIRECTION ( 'NONE',  ( 0.000000000000000000, 0.000000000000000000, 1.000000000000000000 ) ) ;
#56493=CARTESIAN_POINT ( 'NONE',  ( 24.31875000122903074, -5.773502691896255534, -1.060575238724906372E-15 ) ) ;
#56501=CARTESIAN_POINT ( 'NONE',  ( 18.12187500061451928, -4.119189519843968306, 2.378215178124996054 ) ) ;
#56504=CARTESIAN_POINT ( 'NONE',  ( 25.58437500061451431, 5.492252693125287522, 3.363034840372157021E-16 ) ) ;
#56512=CARTESIAN_POINT ( 'NONE',  ( 15.73125000122903216, -4.330127018922194537, 2.499999999999995559 ) ) ;
#56518=CARTESIAN_POINT ( 'NONE',  ( 28.80937500061451573, 4.119189519843966529, -2.378215178124998275 ) ) ;
#56524=CARTESIAN_POINT ( 'NONE',  ( 24.69375000122903074, -2.886751345948130876, 4.999999999999996447 ) ) ;
#56539=CARTESIAN_POINT ( 'NONE',  ( 13.69687500061451679, -2.746126346562646425, 4.756430356249996549 ) ) ;
#56568=CARTESIAN_POINT ( 'NONE',  ( 19.20937500061451786, -4.119189519843965641, -2.378215178125001383 ) ) ;
#56576=CARTESIAN_POINT ( 'NONE',  ( 19.50000000000000000, 4.330127018922192761, -2.499999999999997780 ) ) ;
#56580=CARTESIAN_POINT ( 'NONE',  ( 24.94687500061451502, -4.119189519843965641, -2.378215178125001383 ) ) ;
#56588=CARTESIAN_POINT ( 'NONE',  ( 24.08437500061451075, -2.746126346562642428, -4.756430356249999214 ) ) ;
#56590=CARTESIAN_POINT ( 'NONE',  ( 11.89687500061451608, -4.119189519843965641, -2.378215178125001383 ) ) ;
#56595=FACE_OUTER_BOUND ( 'NONE', #29788, .T. ) ;
#56601=ORIENTED_EDGE ( 'NONE', *, *, #71019, .F. ) ;
#56625=CARTESIAN_POINT ( 'NONE',  ( 20.82187500061451857, 2.746126346562643317, 4.756430356249998326 ) ) ;
#56636=CARTESIAN_POINT ( 'NONE',  ( 7.781250001229034652, 6.123233995736764310E-16, -4.999999999999998224 ) ) ;
#56644=CARTESIAN_POINT ( 'NONE',  ( 16.93125000122903145, 4.330127018922191873, 2.499999999999999556 ) ) ;
#56660=CARTESIAN_POINT ( 'NONE',  ( 25.88437500061451502, -4.119189519843968306, 2.378215178124996054 ) ) ;
#56665=CARTESIAN_POINT ( 'NONE',  ( 25.98750000000000071, -2.886751345948129988, 4.999999999999997335 ) ) ;
#56668=EDGE_CURVE ( 'NONE', #51781, #18169, #40225, .T. ) ;
#56672=CARTESIAN_POINT ( 'NONE',  ( 12.54375000122903394, -2.886751345948129988, 4.999999999999997335 ) ) ;
#56676=CARTESIAN_POINT ( 'NONE',  ( 17.85937500061451644, 2.746126346562645981, -4.756430356249997438 ) ) ;
#56679=ORIENTED_EDGE ( 'NONE', *, *, #45231, .T. ) ;
#56686=CARTESIAN_POINT ( 'NONE',  ( 13.17187500061451466, -4.119189519843968306, 2.378215178124996054 ) ) ;
#56687=ORIENTED_EDGE ( 'NONE', *, *, #25127, .F. ) ;
#56695=CARTESIAN_POINT ( 'NONE',  ( 12.41249999999999964, 2.886751345948182834, 4.999999999999902300 ) ) ;
#56700=ORIENTED_EDGE ( 'NONE', *, *, #14319, .T. ) ;
#56708=CARTESIAN_POINT ( 'NONE',  ( 8.456250001229033586, 0.000000000000000000, 4.999999999999998224 ) ) ;
#56709=CARTESIAN_POINT ( 'NONE',  ( 12.60937500061451821, 4.119189519843966529, -2.378215178124998275 ) ) ;
#56725=CARTESIAN_POINT ( 'NONE',  ( 22.48125000122903216, -4.330127018922194537, 2.499999999999995559 ) ) ;
#56731=PLANE ( 'NONE',  #63189 ) ;
#56771=CARTESIAN_POINT ( 'NONE',  ( 19.88437500061451502, -2.746126346562646425, 4.756430356249996549 ) ) ;
#56786=DIRECTION ( 'NONE',  ( -1.000000000000000000, -0.000000000000000000, -0.000000000000000000 ) ) ;
#56787=CARTESIAN_POINT ( 'NONE',  ( 18.98437500061451644, 4.119189519843966529, 2.378215178124999607 ) ) ;
#56790=CARTESIAN_POINT ( 'NONE',  ( 20.17499999999999716, -4.330127018922194537, 2.499999999999995559 ) ) ;
#56798=ORIENTED_EDGE ( 'NONE', *, *, #41535, .T. ) ;
#56804=CARTESIAN_POINT ( 'NONE',  ( 21.01875000122903003, 2.886751345948126879, 4.999999999999998224 ) ) ;
#56809=CARTESIAN_POINT ( 'NONE',  ( 8.596875000614518925, 5.492252693125287522, 3.363034840372157021E-16 ) ) ;
#56819=VERTEX_POINT ( 'NONE', #23941 ) ;
#56830=CARTESIAN_POINT ( 'NONE',  ( 8.971875000614515372, 2.746126346562645981, -4.756430356249997438 ) ) ;
#56842=CARTESIAN_POINT ( 'NONE',  ( 12.07499999999999929, -4.330127018922194537, 2.499999999999995559 ) ) ;
#56852=CARTESIAN_POINT ( 'NONE',  ( 18.00937500061451502, 2.746126346562643317, 4.756430356249998326 ) ) ;
#56855=CARTESIAN_POINT ( 'NONE',  ( 26.10937500061451644, 2.746126346562643317, 4.756430356249998326 ) ) ;
#56871=CARTESIAN_POINT ( 'NONE',  ( 26.74687500061451573, -2.746126346562646425, 4.756430356249996549 ) ) ;
#56890=CARTESIAN_POINT ( 'NONE',  ( 15.60937500061451644, -4.119189519843965641, -2.378215178125001383 ) ) ;
#56904=CARTESIAN_POINT ( 'NONE',  ( 7.303125000614516082, 0.000000000000000000, 4.756430356249998326 ) ) ;
#56922=CARTESIAN_POINT ( 'NONE',  ( 15.42187500061451821, 2.746126346562643317, 4.756430356249998326 ) ) ;
#56923=FACE_OUTER_BOUND ( 'NONE', #64710, .T. ) ;
#56928=CARTESIAN_POINT ( 'NONE',  ( 17.62500000000000000, 6.123233995736764310E-16, -4.999999999999998224 ) ) ;
#56932=CARTESIAN_POINT ( 'NONE',  ( 25.65937500061451360, 2.746126346562643317, 4.756430356249998326 ) ) ;
#56940=CARTESIAN_POINT ( 'NONE',  ( 24.49687500061451573, -4.119189519843965641, -2.378215178125001383 ) ) ;
#56942=CARTESIAN_POINT ( 'NONE',  ( 11.52187500061451608, 5.824947211148865298E-16, -4.756430356249998326 ) ) ;
#56950=CARTESIAN_POINT ( 'NONE',  ( 17.90625000122903288, 0.000000000000000000, 4.999999999999998224 ) ) ;
#56954=CARTESIAN_POINT ( 'NONE',  ( 13.62187500061451750, -4.119189519843968306, 2.378215178124996054 ) ) ;
#56975=CARTESIAN_POINT ( 'NONE',  ( 22.88437500061451857, 5.824947211148865298E-16, -4.756430356249998326 ) ) ;
#56995=CARTESIAN_POINT ( 'NONE',  ( 16.78125000122903288, 6.123233995736764310E-16, -4.999999999999998224 ) ) ;
#56997=CARTESIAN_POINT ( 'NONE',  ( 10.06875000122903252, 2.886751345948129099, -4.999999999999997335 ) ) ;
#57008=EDGE_CURVE ( 'NONE', #72520, #23570, #41273, .T. ) ;
#57013=CARTESIAN_POINT ( 'NONE',  ( 24.19687500061451857, -2.746126346562642428, -4.756430356249999214 ) ) ;
#57018=CARTESIAN_POINT ( 'NONE',  ( 27.37500000000000000, -4.330127018922194537, 2.499999999999995559 ) ) ;
#57025=CARTESIAN_POINT ( 'NONE',  ( 9.168750001229035718, 2.886751345948129099, -4.999999999999998224 ) ) ;
#57029=CARTESIAN_POINT ( 'NONE',  ( 19.54687500061451289, -4.119189519843965641, -2.378215178125001383 ) ) ;
#57035=CARTESIAN_POINT ( 'NONE',  ( 45.00000000000000000, 0.000000000000000000, 4.999999999999998224 ) ) ;
#57036=CARTESIAN_POINT ( 'NONE',  ( 20.40000000000000213, 4.330127018922192761, -2.499999999999997780 ) ) ;
#57041=CARTESIAN_POINT ( 'NONE',  ( 10.43437500061451395, -2.746126346562646425, 4.756430356249996549 ) ) ;
#57042=ORIENTED_EDGE ( 'NONE', *, *, #67238, .F. ) ;
#57056=ORIENTED_EDGE ( 'NONE', *, *, #20794, .F. ) ;
#57062=CARTESIAN_POINT ( 'NONE',  ( 28.84687500061452425, 5.492252693125287522, 3.363034840372157021E-16 ) ) ;
#57065=CARTESIAN_POINT ( 'NONE',  ( 28.35937500061450933, 2.746126346562643317, 4.756430356249998326 ) ) ;
#57066=CARTESIAN_POINT ( 'NONE',  ( 13.47187500061451537, 2.746126346562645981, -4.756430356249997438 ) ) ;
#57082=CARTESIAN_POINT ( 'NONE',  ( 24.50625000122903074, 4.330127018922192761, -2.499999999999997780 ) ) ;
#57093=EDGE_CURVE ( 'NONE', #38622, #72150, #48826, .T. ) ;
#57107=FACE_OUTER_BOUND ( 'NONE', #31240, .T. ) ;
#57131=CARTESIAN_POINT ( 'NONE',  ( 19.39687500061451786, 0.000000000000000000, 4.756430356249998326 ) ) ;
#57148=CARTESIAN_POINT ( 'NONE',  ( 19.09687500061451360, -2.746126346562646425, 4.756430356249996549 ) ) ;
#57172=DIRECTION ( 'NONE',  ( 0.000000000000000000, 0.000000000000000000, 1.000000000000000000 ) ) ;
#57183=VECTOR ( 'NONE', #66780, 1000.000000000000000 ) ;
#57193=CARTESIAN_POINT ( 'NONE',  ( 8.221875000614518925, 2.746126346562643317, 4.756430356249998326 ) ) ;
#57204=AXIS2_PLACEMENT_3D ( 'NONE', #19444, #47181, #19081 ) ;
#57205=CARTESIAN_POINT ( 'NONE',  ( 24.43125000122903145, 6.123233995736764310E-16, -4.999999999999998224 ) ) ;
#57208=CARTESIAN_POINT ( 'NONE',  ( 45.00000000000000000, 0.000000000000000000, 0.000000000000000000 ) ) ;
#57216=CARTESIAN_POINT ( 'NONE',  ( 16.92187500061451644, 5.824947211148865298E-16, -4.756430356249998326 ) ) ;
#57219=CARTESIAN_POINT ( 'NONE',  ( 26.03437500061451360, 5.492252693125287522, 3.363034840372157021E-16 ) ) ;
#57232=CARTESIAN_POINT ( 'NONE',  ( 27.19687500061451857, -2.746126346562646425, 4.756430356249996549 ) ) ;
#57241=ORIENTED_EDGE ( 'NONE', *, *, #65744, .F. ) ;
#57251=CARTESIAN_POINT ( 'NONE',  ( 14.55937500061451573, 0.000000000000000000, 4.756430356249998326 ) ) ;
#57274=VECTOR ( 'NONE', #44374, 1000.000000000000000 ) ;
#57282=ORIENTED_EDGE ( 'NONE', *, *, #7045, .T. ) ;
#57288=CARTESIAN_POINT ( 'NONE',  ( 16.65937500061452070, 4.119189519843966529, -2.378215178124998275 ) ) ;
#57295=CARTESIAN_POINT ( 'NONE',  ( 17.21249999999999858, 2.886751345948129099, -4.999999999999998224 ) ) ;
#57299=CARTESIAN_POINT ( 'NONE',  ( 23.40937500061451360, 2.746126346562643317, 4.756430356249998326 ) ) ;
#57306=CARTESIAN_POINT ( 'NONE',  ( 25.28437500061451360, -2.746126346562646425, 4.756430356249996549 ) ) ;
#57308=CARTESIAN_POINT ( 'NONE',  ( 10.58437500061451608, -2.746126346562641984, -4.756430356249999214 ) ) ;
#57321=CARTESIAN_POINT ( 'NONE',  ( 10.95937500061451431, -5.492252693125287522, -1.008910452111647106E-15 ) ) ;
#57340=CARTESIAN_POINT ( 'NONE',  ( 22.17187500061451644, 2.746126346562643317, 4.756430356249998326 ) ) ;
#57358=CARTESIAN_POINT ( 'NONE',  ( 15.88125000122903074, 6.123233995736764310E-16, -4.999999999999998224 ) ) ;
#57360=CARTESIAN_POINT ( 'NONE',  ( 9.525000000000002132, 6.123233995736764310E-16, -4.999999999999998224 ) ) ;
#57367=CARTESIAN_POINT ( 'NONE',  ( 10.72500000000000142, -4.330127018922194537, 2.499999999999995559 ) ) ;
#57375=CARTESIAN_POINT ( 'NONE',  ( 23.22187500061451715, -5.492252693125287522, -1.008910452111647106E-15 ) ) ;
#57380=CARTESIAN_POINT ( 'NONE',  ( 25.57499999999999929, -4.330127018922194537, 2.499999999999995559 ) ) ;
#57389=CARTESIAN_POINT ( 'NONE',  ( 10.25625000122903252, 0.000000000000000000, 4.999999999999998224 ) ) ;
#57390=CARTESIAN_POINT ( 'NONE',  ( 13.12500000000000178, 6.123233995736764310E-16, -4.999999999999998224 ) ) ;
#57392=CARTESIAN_POINT ( 'NONE',  ( 17.40937500061451360, 2.746126346562645981, -4.756430356249997438 ) ) ;
#57400=CARTESIAN_POINT ( 'NONE',  ( 10.78125000122903288, -4.330127018922194537, 2.499999999999995559 ) ) ;
#57405=CARTESIAN_POINT ( 'NONE',  ( 9.534375000614517148, -2.746126346562646425, 4.756430356249996549 ) ) ;
#57412=ORIENTED_EDGE ( 'NONE', *, *, #3406, .T. ) ;
#57419=CARTESIAN_POINT ( 'NONE',  ( 10.61250000000000071, 2.886751345948126879, 4.999999999999999112 ) ) ;
#57428=CARTESIAN_POINT ( 'NONE',  ( 29.48437500061451644, -4.119189519843968306, 2.378215178124996054 ) ) ;
#57430=CARTESIAN_POINT ( 'NONE',  ( 27.08437500061451431, -2.746126346562646425, 4.756430356249996549 ) ) ;
#57431=CARTESIAN_POINT ( 'NONE',  ( 12.34687500061452070, -2.746126346562646425, 4.756430356249996549 ) ) ;
#57433=( BOUNDED_CURVE ( )  B_SPLINE_CURVE ( 2, ( #68850, #7505, #40778, #35221, #57742, #24493, #52937 ),
 .UNSPECIFIED., .F., .F. ) 
 B_SPLINE_CURVE_WITH_KNOTS ( ( 3, 2, 2, 3 ),
 ( 0.7399999999999999911, 0.7433333333333332904, 0.7466666666666667007, 0.7500000000000000000 ),
 .UNSPECIFIED. ) 
 CURVE ( )  GEOMETRIC_REPRESENTATION_ITEM ( )  RATIONAL_B_SPLINE_CURVE ( ( 1.000000000000000000, 0.8660254037844387076, 1.000000000000000000, 0.8660254037844387076, 1.000000000000000000, 0.8660254037844387076, 1.000000000000000000 ) ) 
 REPRESENTATION_ITEM ( '' )  );
#57439=LINE ( 'NONE', #6842, #17108 ) ;
#57448=CARTESIAN_POINT ( 'NONE',  ( 23.71875000122903288, 2.886751345948126879, 4.999999999999999112 ) ) ;
#57450=CARTESIAN_POINT ( 'NONE',  ( 22.80000000000000071, 0.000000000000000000, 4.999999999999998224 ) ) ;
#57474=CARTESIAN_POINT ( 'NONE',  ( 45.00000000000000000, -2.499999999999999556, 3.499999999999999556 ) ) ;
#57483=CARTESIAN_POINT ( 'NONE',  ( 19.33125000122903359, -4.330127018922194537, 2.499999999999995559 ) ) ;
#57491=CARTESIAN_POINT ( 'NONE',  ( 11.32500000000000107, 6.123233995736764310E-16, -4.999999999999998224 ) ) ;
#57501=CARTESIAN_POINT ( 'NONE',  ( 18.64687500061451431, -4.119189519843965641, -2.378215178125001383 ) ) ;
#57509=DIRECTION ( 'NONE',  ( -1.000000000000000000, -0.000000000000000000, -0.000000000000000000 ) ) ;
#57514=AXIS2_PLACEMENT_3D ( 'NONE', #18005, #40563, #63082 ) ;
#57519=CARTESIAN_POINT ( 'NONE',  ( 19.95937500061451786, 0.000000000000000000, 4.756430356249998326 ) ) ;
#57532=ORIENTED_EDGE ( 'NONE', *, *, #8491, .F. ) ;
#57541=CARTESIAN_POINT ( 'NONE',  ( 7.809375000614519280, 0.000000000000000000, 4.756430356249998326 ) ) ;
#57560=CARTESIAN_POINT ( 'NONE',  ( 17.75625000122903074, 4.330127018922192761, -2.499999999999997780 ) ) ;
#57561=CARTESIAN_POINT ( 'NONE',  ( 10.24687500061451750, -2.746126346562642428, -4.756430356249999214 ) ) ;
#57572=CARTESIAN_POINT ( 'NONE',  ( 24.35625000122903216, -4.330127018922190985, -2.500000000000001332 ) ) ;
#57573=EDGE_CURVE ( 'NONE', #26559, #8302, #65414, .T. ) ;
#57579=LINE ( 'NONE', #30237, #16283 ) ;
#57582=CARTESIAN_POINT ( 'NONE',  ( 16.58437500061451431, 5.492252693125287522, 3.363034840372157021E-16 ) ) ;
#57585=CARTESIAN_POINT ( 'NONE',  ( 26.85937500061451644, 2.746126346562645981, -4.756430356249997438 ) ) ;
#57589=LINE ( 'NONE', #51697, #72105 ) ;
#57599=CARTESIAN_POINT ( 'NONE',  ( 27.53437500061451360, 4.119189519843966529, 2.378215178124999607 ) ) ;
#57602=FACE_OUTER_BOUND ( 'NONE', #34053, .T. ) ;
#57617=CARTESIAN_POINT ( 'NONE',  ( 14.22187500061451892, -5.492252693125287522, -1.008910452111647106E-15 ) ) ;
#57646=CARTESIAN_POINT ( 'NONE',  ( 16.24687500061451573, 5.492252693125287522, 3.363034840372157021E-16 ) ) ;
#57654=CARTESIAN_POINT ( 'NONE',  ( 17.66249999999999787, 2.886751345948129099, -4.999999999999998224 ) ) ;
#57658=CARTESIAN_POINT ( 'NONE',  ( 23.97187500061451715, -4.119189519843968306, 2.378215178124996054 ) ) ;
#57665=CARTESIAN_POINT ( 'NONE',  ( 24.68437500061451573, 5.492252693125287522, 3.363034840372157021E-16 ) ) ;
#57667=CARTESIAN_POINT ( 'NONE',  ( 11.67187500061451644, 4.119189519843966529, 2.378215178124999607 ) ) ;
#57676=CARTESIAN_POINT ( 'NONE',  ( 29.62500000000000000, -4.330127018922194537, 2.499999999999995559 ) ) ;
#57678=ORIENTED_EDGE ( 'NONE', *, *, #22404, .F. ) ;
#57680=CARTESIAN_POINT ( 'NONE',  ( 11.22187500061451537, 4.119189519843966529, 2.378215178124999607 ) ) ;
#57699=CARTESIAN_POINT ( 'NONE',  ( 22.24687500061451573, -2.746126346562646425, 4.756430356249996549 ) ) ;
#57706=VERTEX_POINT ( 'NONE', #29108 ) ;
#57716=CARTESIAN_POINT ( 'NONE',  ( 45.00000000000000000, 0.000000000000000000, 0.000000000000000000 ) ) ;
#57720=CARTESIAN_POINT ( 'NONE',  ( 45.00000000000000000, 0.000000000000000000, 4.999999999999998224 ) ) ;
#57730=ORIENTED_EDGE ( 'NONE', *, *, #8440, .F. ) ;
#57734=CARTESIAN_POINT ( 'NONE',  ( 22.58437500061451431, 4.119189519843966529, 2.378215178124999607 ) ) ;
#57739=CARTESIAN_POINT ( 'NONE',  ( 24.56250000000000000, 2.886751345948126879, 4.999999999999999112 ) ) ;
#57742=CARTESIAN_POINT ( 'NONE',  ( 12.80625000122903323, 4.330127018922192761, -2.499999999999997780 ) ) ;
#57744=CARTESIAN_POINT ( 'NONE',  ( 24.44999999999999929, 4.330127018922192761, -2.499999999999997780 ) ) ;
#57748=CARTESIAN_POINT ( 'NONE',  ( 10.48125000122903216, 6.123233995736764310E-16, -4.999999999999998224 ) ) ;
#57751=CARTESIAN_POINT ( 'NONE',  ( 17.44687500061451502, 4.119189519843966529, -2.378215178124998275 ) ) ;
#57762=CARTESIAN_POINT ( 'NONE',  ( 10.05937500061451750, -5.492252693125287522, -1.008910452111647106E-15 ) ) ;
#57774=CARTESIAN_POINT ( 'NONE',  ( 11.21250000000000036, -5.773502691896255534, -1.060575238724906372E-15 ) ) ;
#57777=ORIENTED_EDGE ( 'NONE', *, *, #38932, .T. ) ;
#57780=EDGE_CURVE ( 'NONE', #42476, #69693, #39842, .T. ) ;
#57783=CARTESIAN_POINT ( 'NONE',  ( 28.92187500061451644, 2.746126346562643317, 4.756430356249998326 ) ) ;
#57785=CARTESIAN_POINT ( 'NONE',  ( 27.27187500061451786, 5.824947211148865298E-16, -4.756430356249998326 ) ) ;
#57786=CARTESIAN_POINT ( 'NONE',  ( 12.98437500061451821, 5.824947211148865298E-16, -4.756430356249998326 ) ) ;
#57794=DIRECTION ( 'NONE',  ( 0.000000000000000000, 0.000000000000000000, 1.000000000000000000 ) ) ;
#57797=( NAMED_UNIT ( * ) PLANE_ANGLE_UNIT ( ) SI_UNIT ( $, .RADIAN. ) );
#57802=CARTESIAN_POINT ( 'NONE',  ( 24.01875000122903359, 2.886751345948129099, -4.999999999999998224 ) ) ;
#57804=CARTESIAN_POINT ( 'NONE',  ( 22.76249999999999574, 2.886751345948098901, 5.000000000000047073 ) ) ;
#57847=ORIENTED_EDGE ( 'NONE', *, *, #70340, .F. ) ;
#57854=CARTESIAN_POINT ( 'NONE',  ( 18.04687500061451644, 0.000000000000000000, 4.756430356249998326 ) ) ;
#57862=CARTESIAN_POINT ( 'NONE',  ( 11.53125000122903465, 4.330127018922191873, 2.499999999999999556 ) ) ;
#57870=CARTESIAN_POINT ( 'NONE',  ( 45.00000000000000000, 0.000000000000000000, 0.000000000000000000 ) ) ;
#57871=FACE_OUTER_BOUND ( 'NONE', #40946, .T. ) ;
#57872=CARTESIAN_POINT ( 'NONE',  ( 20.25937500061451857, 4.119189519843966529, -2.378215178124998275 ) ) ;
#57883=FACE_OUTER_BOUND ( 'NONE', #39002, .T. ) ;
#57886=CARTESIAN_POINT ( 'NONE',  ( 34.99999999999999289, 2.500000000000000444, 3.499999999999999112 ) ) ;
#57895=CARTESIAN_POINT ( 'NONE',  ( 22.70625000122903003, 4.330127018922192761, -2.499999999999997780 ) ) ;
#57900=CYLINDRICAL_SURFACE ( 'NONE', #55959, 4.999999999999998224 ) ;
#57917=CARTESIAN_POINT ( 'NONE',  ( 9.984375000614518214, 4.119189519843966529, 2.378215178124999607 ) ) ;
#57919=CARTESIAN_POINT ( 'NONE',  ( 20.26875000122903359, -5.773502691896255534, -1.060575238724906372E-15 ) ) ;
#57924=CARTESIAN_POINT ( 'NONE',  ( 11.92500000000000071, 4.330127018922191873, 2.499999999999999556 ) ) ;
#57928=DIRECTION ( 'NONE',  ( -1.000000000000000000, -0.000000000000000000, -0.000000000000000000 ) ) ;
#57937=CARTESIAN_POINT ( 'NONE',  ( 17.74687500061451928, -4.119189519843965641, -2.378215178125001383 ) ) ;
#57940=CARTESIAN_POINT ( 'NONE',  ( 25.92187500061451644, 5.824947211148865298E-16, -4.756430356249998326 ) ) ;
#57954=CARTESIAN_POINT ( 'NONE',  ( 27.00937500061451857, 4.119189519843966529, -2.378215178124998275 ) ) ;
#57962=ORIENTED_EDGE ( 'NONE', *, *, #66859, .T. ) ;
#57972=CARTESIAN_POINT ( 'NONE',  ( 12.83437500061451786, -4.119189519843968306, 2.378215178124996054 ) ) ;
#57985=VERTEX_POINT ( 'NONE', #65906 ) ;
#58003=CARTESIAN_POINT ( 'NONE',  ( 17.22187500061451715, 2.746126346562643317, 4.756430356249998326 ) ) ;
#58009=CARTESIAN_POINT ( 'NONE',  ( 16.57499999999999929, -4.330127018922194537, 2.499999999999995559 ) ) ;
#58013=CARTESIAN_POINT ( 'NONE',  ( 22.73437500061451999, -2.746126346562641984, -4.756430356249999214 ) ) ;
#58020=CARTESIAN_POINT ( 'NONE',  ( 24.72187500061451360, 4.119189519843966529, 2.378215178124999607 ) ) ;
#58022=CARTESIAN_POINT ( 'NONE',  ( 12.27187500061451608, -4.119189519843968306, 2.378215178124996054 ) ) ;
#58034=CARTESIAN_POINT ( 'NONE',  ( 10.73437500061451644, 5.492252693125287522, 3.363034840372157021E-16 ) ) ;
#58042=LINE ( 'NONE', #7816, #21889 ) ;
#58052=CARTESIAN_POINT ( 'NONE',  ( 11.36249999999999716, 2.886751345948073588, -5.000000000000094147 ) ) ;
#58054=CARTESIAN_POINT ( 'NONE',  ( 22.02187500061451786, 2.746126346562645981, -4.756430356249997438 ) ) ;
#58073=ADVANCED_FACE ( 'NONE', ( #69012 ), #57900, .T. ) ;
#58085=ORIENTED_EDGE ( 'NONE', *, *, #40891, .F. ) ;
#58089=CARTESIAN_POINT ( 'NONE',  ( 23.63437500061451502, -4.119189519843968306, 2.378215178124996054 ) ) ;
#58096=CARTESIAN_POINT ( 'NONE',  ( 24.22500000000000142, -4.330127018922194537, 2.499999999999995559 ) ) ;
#58105=CARTESIAN_POINT ( 'NONE',  ( 8.943750001229034297, -2.886751345948129988, 4.999999999999997335 ) ) ;
#58108=CARTESIAN_POINT ( 'NONE',  ( 17.67187500061451644, -4.119189519843968306, 2.378215178124996054 ) ) ;
#58111=ORIENTED_EDGE ( 'NONE', *, *, #72508, .T. ) ;
#58115=LINE ( 'NONE', #64030, #59645 ) ;
#58119=CARTESIAN_POINT ( 'NONE',  ( 10.58437500061451608, -2.746126346562642428, -4.756430356249999214 ) ) ;
#58120=VERTEX_POINT ( 'NONE', #46129 ) ;
#58125=( BOUNDED_CURVE ( )  B_SPLINE_CURVE ( 2, ( #42355, #41990, #59693, #8364, #9468, #36804, #31638 ),
 .UNSPECIFIED., .F., .F. ) 
 B_SPLINE_CURVE_WITH_KNOTS ( ( 3, 2, 2, 3 ),
 ( 0.1599999999999999756, 0.1633333333333333026, 0.1666666666666666019, 0.1699999999999999567 ),
 .UNSPECIFIED. ) 
 CURVE ( )  GEOMETRIC_REPRESENTATION_ITEM ( )  RATIONAL_B_SPLINE_CURVE ( ( 1.000000000000001332, 0.8660254037844377084, 1.000000000000000000, 0.8660254037844387076, 1.000000000000000000, 0.8660254037844409281, 0.9999999999999977796 ) ) 
 REPRESENTATION_ITEM ( '' )  );
#58127=CARTESIAN_POINT ( 'NONE',  ( 19.68750000000000000, -2.886751345948130876, 4.999999999999996447 ) ) ;
#58131=CARTESIAN_POINT ( 'NONE',  ( 28.32187500061451502, 4.119189519843966529, 2.378215178124999607 ) ) ;
#58134=CARTESIAN_POINT ( 'NONE',  ( 9.262499999999999289, 2.886751345948126879, 4.999999999999999112 ) ) ;
#58142=CARTESIAN_POINT ( 'NONE',  ( 29.59687500061451715, -2.746126346562641984, -4.756430356249999214 ) ) ;
#58144=CARTESIAN_POINT ( 'NONE',  ( 27.98437500061450933, -2.746126346562646425, 4.756430356249996549 ) ) ;
#58145=CARTESIAN_POINT ( 'NONE',  ( 10.58437500061451964, -4.119189519843968306, 2.378215178124996054 ) ) ;
#58147=ADVANCED_FACE ( 'NONE', ( #53113 ), #29497, .T. ) ;
#58162=CARTESIAN_POINT ( 'NONE',  ( 23.64375000122903003, 5.773502691896255534, 3.535250795749688894E-16 ) ) ;
#58165=ORIENTED_EDGE ( 'NONE', *, *, #39715, .F. ) ;
#58181=EDGE_CURVE ( 'NONE', #1580, #55986, #49899, .T. ) ;
#58186=CARTESIAN_POINT ( 'NONE',  ( 25.50000000000000000, 0.000000000000000000, 4.999999999999998224 ) ) ;
#58196=CARTESIAN_POINT ( 'NONE',  ( 19.48125000122903216, 6.123233995736764310E-16, -4.999999999999998224 ) ) ;
#58199=VERTEX_POINT ( 'NONE', #35035 ) ;
#58200=CARTESIAN_POINT ( 'NONE',  ( 12.73125000122903394, 6.123233995736764310E-16, -4.999999999999998224 ) ) ;
#58207=EDGE_LOOP ( 'NONE', ( #2021, #20285, #46691, #34287 ) ) ;
#58213=CARTESIAN_POINT ( 'NONE',  ( 15.75937500061451502, 2.746126346562643317, 4.756430356249998326 ) ) ;
#58230=CARTESIAN_POINT ( 'NONE',  ( 17.90625000122903288, 0.000000000000000000, 4.999999999999998224 ) ) ;
#58233=CARTESIAN_POINT ( 'NONE',  ( 20.48437500061451289, -4.119189519843968306, 2.378215178124996054 ) ) ;
#58244=CYLINDRICAL_SURFACE ( 'NONE', #57204, 4.999999999999998224 ) ;
#58247=PLANE ( 'NONE',  #54427 ) ;
#58253=CARTESIAN_POINT ( 'NONE',  ( 7.612500000000000711, -5.773502691896255534, -1.060575238724906372E-15 ) ) ;
#58254=CARTESIAN_POINT ( 'NONE',  ( 22.74375000122903145, 5.773502691896255534, 3.535250795749688401E-16 ) ) ;
#58276=CARTESIAN_POINT ( 'NONE',  ( 29.17500000000000071, -4.330127018922194537, 2.499999999999995559 ) ) ;
#58286=DIRECTION ( 'NONE',  ( -1.000000000000000000, -0.000000000000000000, -0.000000000000000000 ) ) ;
#58296=CARTESIAN_POINT ( 'NONE',  ( 14.97187500061451537, -4.119189519843968306, 2.378215178124996054 ) ) ;
#58299=CARTESIAN_POINT ( 'NONE',  ( 24.72187500061451360, 4.119189519843966529, 2.378215178124999607 ) ) ;
#58313=CARTESIAN_POINT ( 'NONE',  ( 27.94687500061451502, 5.492252693125287522, 3.363034840372157021E-16 ) ) ;
#58331=CARTESIAN_POINT ( 'NONE',  ( 13.02187500061451786, 2.746126346562645981, -4.756430356249997438 ) ) ;
#58362=CARTESIAN_POINT ( 'NONE',  ( 17.10937500061451999, 4.119189519843966529, -2.378215178124998275 ) ) ;
#58370=CARTESIAN_POINT ( 'NONE',  ( 18.63749999999999929, 5.773502691896255534, 3.535250795749688894E-16 ) ) ;
#58373=CARTESIAN_POINT ( 'NONE',  ( 23.78437500061451360, 5.492252693125287522, 3.363034840372157021E-16 ) ) ;
#58376=CARTESIAN_POINT ( 'NONE',  ( 26.39999999999999858, 0.000000000000000000, 4.999999999999998224 ) ) ;
#58381=CARTESIAN_POINT ( 'NONE',  ( 23.55937500061451573, -5.492252693125287522, -1.008910452111647106E-15 ) ) ;
#58383=CARTESIAN_POINT ( 'NONE',  ( 9.646875000614514306, -4.119189519843965641, -2.378215178125001383 ) ) ;
#58392=CARTESIAN_POINT ( 'NONE',  ( 10.20000000000000107, 0.000000000000000000, 4.999999999999998224 ) ) ;
#58395=CARTESIAN_POINT ( 'NONE',  ( 12.42187500061451466, 5.824947211148865298E-16, -4.756430356249998326 ) ) ;
#58407=ORIENTED_EDGE ( 'NONE', *, *, #32675, .T. ) ;
#58416=CARTESIAN_POINT ( 'NONE',  ( 18.45937500061451431, 4.119189519843966529, -2.378215178124998275 ) ) ;
#58418=CARTESIAN_POINT ( 'NONE',  ( 28.66875000122903216, 2.886751345948161962, 4.999999999999938716 ) ) ;
#58451=CARTESIAN_POINT ( 'NONE',  ( 23.29687500061451644, -2.746126346562642428, -4.756430356249999214 ) ) ;
#58457=CARTESIAN_POINT ( 'NONE',  ( 24.97499999999999787, 4.330127018922191873, 2.499999999999999556 ) ) ;
#58458=VECTOR ( 'NONE', #15747, 1000.000000000000000 ) ;
#58467=CARTESIAN_POINT ( 'NONE',  ( 9.281250001229032875, 4.330127018922191873, 2.499999999999999556 ) ) ;
#58469=CARTESIAN_POINT ( 'NONE',  ( 16.20937500061451431, 2.746126346562643317, 4.756430356249998326 ) ) ;
#58473=ORIENTED_EDGE ( 'NONE', *, *, #38317, .T. ) ;
#58478=EDGE_CURVE ( 'NONE', #44169, #46196, #47505, .T. ) ;
#58483=CARTESIAN_POINT ( 'NONE',  ( 10.62187500061451395, 5.824947211148865298E-16, -4.756430356249998326 ) ) ;
#58494=CARTESIAN_POINT ( 'NONE',  ( 28.95937500061451075, -5.492252693125287522, -1.008910452111647106E-15 ) ) ;
#58497=CARTESIAN_POINT ( 'NONE',  ( 9.150000000000002132, 4.330127018922192761, -2.499999999999997780 ) ) ;
#58505=CARTESIAN_POINT ( 'NONE',  ( 26.37187500061451573, -5.492252693125287522, -1.008910452111647106E-15 ) ) ;
#58507=CARTESIAN_POINT ( 'NONE',  ( 11.22187500061451892, 2.746126346562645981, -4.756430356249997438 ) ) ;
#58522=CARTESIAN_POINT ( 'NONE',  ( 20.60625000122902861, 0.000000000000000000, 4.999999999999998224 ) ) ;
#58548=AXIS2_PLACEMENT_3D ( 'NONE', #27595, #21907, #72518 ) ;
#58549=ADVANCED_FACE ( 'NONE', ( #26510 ), #20214, .T. ) ;
#58559=CARTESIAN_POINT ( 'NONE',  ( 19.25625000122903430, 0.000000000000000000, 4.999999999999998224 ) ) ;
#58560=AXIS2_PLACEMENT_3D ( 'NONE', #16319, #45136, #5613 ) ;
#58579=CARTESIAN_POINT ( 'NONE',  ( 16.62187500061451573, 4.119189519843966529, 2.378215178124999607 ) ) ;
#58596=PLANE ( 'NONE',  #20632 ) ;
#58600=CARTESIAN_POINT ( 'NONE',  ( 16.73437500061451644, 4.119189519843966529, 2.378215178124999607 ) ) ;
#58617=CARTESIAN_POINT ( 'NONE',  ( 28.59375000122903288, 5.773502691896255534, 3.535250795749688894E-16 ) ) ;
#58620=AXIS2_PLACEMENT_3D ( 'NONE', #69037, #58286, #7692 ) ;
#58622=CARTESIAN_POINT ( 'NONE',  ( 14.69999999999999929, 0.000000000000000000, 4.999999999999998224 ) ) ;
#58643=CARTESIAN_POINT ( 'NONE',  ( 7.359375000614516438, 0.000000000000000000, 4.756430356249998326 ) ) ;
#58645=CARTESIAN_POINT ( 'NONE',  ( 20.19375000122903430, -2.886751345948074920, 5.000000000000092371 ) ) ;
#58663=CARTESIAN_POINT ( 'NONE',  ( 15.57187500061451679, 5.824947211148865298E-16, -4.756430356249998326 ) ) ;
#58666=CARTESIAN_POINT ( 'NONE',  ( 22.62187500061451573, -4.119189519843968306, 2.378215178124996054 ) ) ;
#58670=CARTESIAN_POINT ( 'NONE',  ( 28.76250000000000284, -5.773502691896255534, -1.060575238724906372E-15 ) ) ;
#58680=CARTESIAN_POINT ( 'NONE',  ( 24.15937500061451715, -4.119189519843965641, -2.378215178125001383 ) ) ;
#58684=DIRECTION ( 'NONE',  ( 0.000000000000000000, 0.000000000000000000, 1.000000000000000000 ) ) ;
#58700=CARTESIAN_POINT ( 'NONE',  ( 12.98437500061451821, 5.824947211148865298E-16, -4.756430356249998326 ) ) ;
#58729=CARTESIAN_POINT ( 'NONE',  ( 15.12187500061451750, -5.492252693125287522, -1.008910452111647106E-15 ) ) ;
#58736=CARTESIAN_POINT ( 'NONE',  ( 16.19999999999999929, -4.330127018922190985, -2.500000000000001332 ) ) ;
#58739=DIRECTION ( 'NONE',  ( -1.000000000000000000, -0.000000000000000000, -0.000000000000000000 ) ) ;
#58740=CARTESIAN_POINT ( 'NONE',  ( 23.52187500061451431, -4.119189519843968306, 2.378215178124996054 ) ) ;
#58748=CARTESIAN_POINT ( 'NONE',  ( 23.14687500061451786, -4.119189519843965641, -2.378215178125001383 ) ) ;
#58750=CARTESIAN_POINT ( 'NONE',  ( 8.371875000614515727, 5.824947211148865298E-16, -4.756430356249998326 ) ) ;
#58757=CARTESIAN_POINT ( 'NONE',  ( 29.66249999999999787, -5.773502691896255534, -1.060575238724906372E-15 ) ) ;
#58761=CARTESIAN_POINT ( 'NONE',  ( 8.521875000614517859, 4.119189519843966529, 2.378215178124999607 ) ) ;
#58784=CARTESIAN_POINT ( 'NONE',  ( 20.10937500061451289, -4.119189519843965641, -2.378215178125001383 ) ) ;
#58810=DIRECTION ( 'NONE',  ( -1.000000000000000000, -0.000000000000000000, -0.000000000000000000 ) ) ;
#58813=ORIENTED_EDGE ( 'NONE', *, *, #24066, .T. ) ;
#58818=CARTESIAN_POINT ( 'NONE',  ( 21.15937500061451715, 4.119189519843966529, -2.378215178124998275 ) ) ;
#58821=ADVANCED_FACE ( 'NONE', ( #66770 ), #34579, .T. ) ;
#58824=CARTESIAN_POINT ( 'NONE',  ( 24.44999999999999929, 4.330127018922192761, -2.499999999999997780 ) ) ;
#58829=DIRECTION ( 'NONE',  ( 0.000000000000000000, 0.000000000000000000, 1.000000000000000000 ) ) ;
#58835=CARTESIAN_POINT ( 'NONE',  ( 28.54687500061451644, -4.119189519843965641, -2.378215178125001383 ) ) ;
#58837=CARTESIAN_POINT ( 'NONE',  ( 15.45937500061451608, -5.492252693125287522, -1.008910452111647106E-15 ) ) ;
#58840=VERTEX_POINT ( 'NONE', #45320 ) ;
#58849=CARTESIAN_POINT ( 'NONE',  ( 8.409375000614517148, 2.746126346562645981, -4.756430356249997438 ) ) ;
#58855=ORIENTED_EDGE ( 'NONE', *, *, #58478, .F. ) ;
#58860=CARTESIAN_POINT ( 'NONE',  ( 29.52187500061451431, 5.824947211148865298E-16, -4.756430356249998326 ) ) ;
#58863=CARTESIAN_POINT ( 'NONE',  ( 7.687500000000000000, -2.886751345948125991, -5.000000000000000000 ) ) ;
#58870=CARTESIAN_POINT ( 'NONE',  ( 25.65937500061451715, 4.119189519843966529, -2.378215178124998275 ) ) ;
#58872=CARTESIAN_POINT ( 'NONE',  ( 10.99687500061451750, -2.746126346562646425, 4.756430356249996549 ) ) ;
#58884=SURFACE_STYLE_USAGE ( .BOTH. , #63355 ) ;
#58889=CARTESIAN_POINT ( 'NONE',  ( 21.95625000122903003, 0.000000000000000000, 4.999999999999998224 ) ) ;
#58904=CARTESIAN_POINT ( 'NONE',  ( 28.43437500061451573, 4.119189519843966529, 2.378215178124999607 ) ) ;
#58941=CARTESIAN_POINT ( 'NONE',  ( 17.52187500061451431, 4.119189519843966529, 2.378215178124999607 ) ) ;
#58961=CARTESIAN_POINT ( 'NONE',  ( 16.58437500061451786, 5.824947211148865298E-16, -4.756430356249998326 ) ) ;
#58970=ADVANCED_FACE ( 'NONE', ( #39787 ), #73029, .T. ) ;
#58973=VERTEX_POINT ( 'NONE', #68220 ) ;
#58980=CARTESIAN_POINT ( 'NONE',  ( 28.70625000122903003, 0.000000000000000000, 4.999999999999998224 ) ) ;
#58982=DIRECTION ( 'NONE',  ( 0.000000000000000000, 0.000000000000000000, 1.000000000000000000 ) ) ;
#59006=CARTESIAN_POINT ( 'NONE',  ( 7.884375000614517681, -4.119189519843968306, 2.378215178124996054 ) ) ;
#59010=EDGE_CURVE ( 'NONE', #18738, #34725, #17227, .T. ) ;
#59016=( BOUNDED_CURVE ( )  B_SPLINE_CURVE ( 2, ( #19120, #13584, #14322, #53118, #19858, #3253, #36857 ),
 .UNSPECIFIED., .F., .F. ) 
 B_SPLINE_CURVE_WITH_KNOTS ( ( 3, 2, 2, 3 ),
 ( 0.1099999999999999312, 0.1133333333333333137, 0.1166666666666666963, 0.1200000000000000788 ),
 .UNSPECIFIED. ) 
 CURVE ( )  GEOMETRIC_REPRESENTATION_ITEM ( )  RATIONAL_B_SPLINE_CURVE ( ( 1.000000000000002887, 0.8660254037844359321, 1.000000000000000000, 0.8660254037844387076, 1.000000000000000000, 0.8660254037844353769, 1.000000000000003331 ) ) 
 REPRESENTATION_ITEM ( '' )  );
#59026=CARTESIAN_POINT ( 'NONE',  ( 16.32187500061451502, -4.119189519843968306, 2.378215178124996054 ) ) ;
#59029=CARTESIAN_POINT ( 'NONE',  ( 22.73437500061451999, -2.746126346562642428, -4.756430356249999214 ) ) ;
#59038=CARTESIAN_POINT ( 'NONE',  ( 24.65625000122903288, 0.000000000000000000, 4.999999999999998224 ) ) ;
#59045=CARTESIAN_POINT ( 'NONE',  ( 25.05937500061451573, -4.119189519843965641, -2.378215178125001383 ) ) ;
#59048=CARTESIAN_POINT ( 'NONE',  ( 25.05000000000000071, 0.000000000000000000, 4.999999999999998224 ) ) ;
#59055=CARTESIAN_POINT ( 'NONE',  ( 25.10625000122903216, 0.000000000000000000, 4.999999999999998224 ) ) ;
#59065=CARTESIAN_POINT ( 'NONE',  ( 12.27187500061451608, 2.746126346562643317, 4.756430356249998326 ) ) ;
#59083=CARTESIAN_POINT ( 'NONE',  ( 14.86875000122903323, -5.773502691896255534, -1.060575238724906372E-15 ) ) ;
#59095=CARTESIAN_POINT ( 'NONE',  ( 13.69687500061451679, -2.746126346562646425, 4.756430356249996549 ) ) ;
#59102=CARTESIAN_POINT ( 'NONE',  ( 16.08749999999999503, -2.886751345948129988, 4.999999999999997335 ) ) ;
#59105=CARTESIAN_POINT ( 'NONE',  ( 15.37500000000000000, 6.123233995736764310E-16, -4.999999999999998224 ) ) ;
#59115=CARTESIAN_POINT ( 'NONE',  ( 22.09687500061451360, 0.000000000000000000, 4.756430356249998326 ) ) ;
#59117=CARTESIAN_POINT ( 'NONE',  ( 7.771875000614516082, -4.119189519843968306, 2.378215178124996054 ) ) ;
#59121=CARTESIAN_POINT ( 'NONE',  ( 9.074999999999999289, 6.123233995736764310E-16, -4.999999999999998224 ) ) ;
#59125=CARTESIAN_POINT ( 'NONE',  ( 10.12500000000000178, 4.330127018922191873, 2.499999999999999556 ) ) ;
#59128=CARTESIAN_POINT ( 'NONE',  ( 8.221875000614515372, -4.119189519843968306, 2.378215178124996054 ) ) ;
#59139=ORIENTED_EDGE ( 'NONE', *, *, #51006, .F. ) ;
#59150=CARTESIAN_POINT ( 'NONE',  ( 18.75937500061451857, -4.119189519843965641, -2.378215178125001383 ) ) ;
#59178=ORIENTED_EDGE ( 'NONE', *, *, #63830, .T. ) ;
#59182=CARTESIAN_POINT ( 'NONE',  ( 21.57187500061451502, 2.746126346562645981, -4.756430356249997438 ) ) ;
#59188=CARTESIAN_POINT ( 'NONE',  ( 22.68750000000000000, 5.773502691896255534, 3.535250795749688894E-16 ) ) ;
#59194=CARTESIAN_POINT ( 'NONE',  ( 19.70625000122903359, 0.000000000000000000, 4.999999999999998224 ) ) ;
#59200=CARTESIAN_POINT ( 'NONE',  ( 7.818750001229033408, 2.886751345948129099, -4.999999999999998224 ) ) ;
#59202=CARTESIAN_POINT ( 'NONE',  ( 16.92187500061451644, 5.824947211148865298E-16, -4.756430356249998326 ) ) ;
#59212=CARTESIAN_POINT ( 'NONE',  ( 16.66875000122903216, -5.773502691896255534, -1.060575238724906372E-15 ) ) ;
#59213=CARTESIAN_POINT ( 'NONE',  ( 7.246875000614514839, 0.000000000000000000, 4.756430356249998326 ) ) ;
#59224=CARTESIAN_POINT ( 'NONE',  ( 28.43437500061451573, -2.746126346562646425, 4.756430356249996549 ) ) ;
#59235=CARTESIAN_POINT ( 'NONE',  ( 27.64687500061452141, -2.746126346562646425, 4.756430356249996549 ) ) ;
#59237=CARTESIAN_POINT ( 'NONE',  ( 9.871875000614517504, 2.746126346562645981, -4.756430356249997438 ) ) ;
#59244=EDGE_CURVE ( 'NONE', #45117, #10316, #12133, .T. ) ;
#59255=CARTESIAN_POINT ( 'NONE',  ( 20.23125000122902861, -4.330127018922194537, 2.499999999999995559 ) ) ;
#59270=CARTESIAN_POINT ( 'NONE',  ( 27.87187500061451573, 2.746126346562645981, -4.756430356249997438 ) ) ;
#59278=CARTESIAN_POINT ( 'NONE',  ( 7.481250001229032165, 4.330127018922191873, 2.499999999999999556 ) ) ;
#59286=CARTESIAN_POINT ( 'NONE',  ( 23.09999999999999787, 4.330127018922192761, -2.499999999999997780 ) ) ;
#59293=CYLINDRICAL_SURFACE ( 'NONE', #61983, 4.999999999999998224 ) ;
#59304=CARTESIAN_POINT ( 'NONE',  ( 17.44687500061451502, 4.119189519843966529, -2.378215178124998275 ) ) ;
#59323=CARTESIAN_POINT ( 'NONE',  ( 17.03437500061451715, 5.824947211148865298E-16, -4.756430356249998326 ) ) ;
#59332=ADVANCED_FACE ( 'NONE', ( #2068 ), #47123, .T. ) ;
#59335=ORIENTED_EDGE ( 'NONE', *, *, #27670, .F. ) ;
#59342=CARTESIAN_POINT ( 'NONE',  ( 27.65625000122902932, 4.330127018922192761, -2.499999999999997780 ) ) ;
#59344=CARTESIAN_POINT ( 'NONE',  ( 45.00000000000000000, 0.000000000000000000, 4.999999999999998224 ) ) ;
#59367=CARTESIAN_POINT ( 'NONE',  ( 28.42499999999999716, 6.123233995736764310E-16, -4.999999999999998224 ) ) ;
#59379=CARTESIAN_POINT ( 'NONE',  ( 22.38749999999999574, -2.886751345948102898, 5.000000000000044409 ) ) ;
#59386=EDGE_CURVE ( 'NONE', #71135, #5961, #18663, .T. ) ;
#59388=CARTESIAN_POINT ( 'NONE',  ( 15.79687500061451644, 0.000000000000000000, 4.756430356249998326 ) ) ;
#59391=CARTESIAN_POINT ( 'NONE',  ( 23.29687500061451644, 4.119189519843966529, -2.378215178124998275 ) ) ;
#59400=ADVANCED_FACE ( 'NONE', ( #987 ), #68938, .T. ) ;
#59401=CARTESIAN_POINT ( 'NONE',  ( 23.56875000122903074, 2.886751345948101122, -5.000000000000046185 ) ) ;
#59402=CARTESIAN_POINT ( 'NONE',  ( 13.42499999999999893, -4.330127018922194537, 2.499999999999995559 ) ) ;
#59410=CARTESIAN_POINT ( 'NONE',  ( 25.24687500061451573, 5.492252693125287522, 3.363034840372157021E-16 ) ) ;
#59421=CARTESIAN_POINT ( 'NONE',  ( 45.00000000000000000, 0.000000000000000000, 4.999999999999998224 ) ) ;
#59431=CARTESIAN_POINT ( 'NONE',  ( 11.67187500061451821, 2.746126346562645981, -4.756430356249997438 ) ) ;
#59445=ORIENTED_EDGE ( 'NONE', *, *, #1067, .T. ) ;
#59457=VERTEX_POINT ( 'NONE', #51945 ) ;
#59460=CARTESIAN_POINT ( 'NONE',  ( 13.47187500061451537, 2.746126346562645981, -4.756430356249997438 ) ) ;
#59468=CARTESIAN_POINT ( 'NONE',  ( 15.15000000000000036, 0.000000000000000000, 4.999999999999998224 ) ) ;
#59473=ORIENTED_EDGE ( 'NONE', *, *, #44600, .F. ) ;
#59481=CARTESIAN_POINT ( 'NONE',  ( 22.92187500061451644, 4.119189519843966529, 2.378215178124999607 ) ) ;
#59483=CARTESIAN_POINT ( 'NONE',  ( 8.334375000614516082, -2.746126346562641984, -4.756430356249999214 ) ) ;
#59492=CARTESIAN_POINT ( 'NONE',  ( 8.831250001229033586, 4.330127018922191873, 2.499999999999999556 ) ) ;
#59494=CARTESIAN_POINT ( 'NONE',  ( 9.609375000614514661, -5.492252693125287522, -1.008910452111647106E-15 ) ) ;
#59504=ORIENTED_EDGE ( 'NONE', *, *, #6481, .T. ) ;
#59515=EDGE_CURVE ( 'NONE', #46954, #3601, #42332, .T. ) ;
#59517=CARTESIAN_POINT ( 'NONE',  ( 20.25937500061451857, 4.119189519843966529, -2.378215178124998275 ) ) ;
#59530=VERTEX_POINT ( 'NONE', #40868 ) ;
#59537=EDGE_CURVE ( 'NONE', #32794, #61283, #35216, .T. ) ;
#59549=VECTOR ( 'NONE', #8237, 1000.000000000000000 ) ;
#59551=CARTESIAN_POINT ( 'NONE',  ( 21.79687500061451644, -2.746126346562646425, 4.756430356249996549 ) ) ;
#59557=CARTESIAN_POINT ( 'NONE',  ( 22.80000000000000071, 0.000000000000000000, 4.999999999999998224 ) ) ;
#59563=FACE_OUTER_BOUND ( 'NONE', #31992, .T. ) ;
#59567=CARTESIAN_POINT ( 'NONE',  ( 7.781250001229034652, 6.123233995736764310E-16, -4.999999999999998224 ) ) ;
#59569=CARTESIAN_POINT ( 'NONE',  ( 17.18437500061451573, -2.746126346562646425, 4.756430356249996549 ) ) ;
#59570=AXIS2_PLACEMENT_3D ( 'NONE', #67904, #34264, #24274 ) ;
#59591=CARTESIAN_POINT ( 'NONE',  ( 27.83437500061451075, 5.492252693125287522, 3.363034840372157021E-16 ) ) ;
#59595=CARTESIAN_POINT ( 'NONE',  ( 8.287499999999999645, 5.773502691896255534, 3.535250795749688894E-16 ) ) ;
#59596=AXIS2_PLACEMENT_3D ( 'NONE', #7201, #29730, #52268 ) ;
#59603=CARTESIAN_POINT ( 'NONE',  ( 26.22187500061451715, 2.746126346562643317, 4.756430356249998326 ) ) ;
#59605=CARTESIAN_POINT ( 'NONE',  ( 9.534375000614517148, 4.119189519843966529, 2.378215178124999607 ) ) ;
#59622=CARTESIAN_POINT ( 'NONE',  ( 20.68125000122903145, -4.330127018922194537, 2.499999999999995559 ) ) ;
#59626=ADVANCED_FACE ( 'NONE', ( #57107 ), #19384, .T. ) ;
#59631=CARTESIAN_POINT ( 'NONE',  ( 23.26875000122903003, 2.886751345948126879, 4.999999999999998224 ) ) ;
#59637=MECHANICAL_DESIGN_GEOMETRIC_PRESENTATION_REPRESENTATION('',(#13649),#65557);
#59639=CARTESIAN_POINT ( 'NONE',  ( 28.58437500061451786, -4.119189519843968306, 2.378215178124996054 ) ) ;
#59645=VECTOR ( 'NONE', #35957, 1000.000000000000000 ) ;
#59663=ORIENTED_EDGE ( 'NONE', *, *, #1636, .F. ) ;
#59664=CARTESIAN_POINT ( 'NONE',  ( 10.48125000122903216, 6.123233995736764310E-16, -4.999999999999998224 ) ) ;
#59678=CARTESIAN_POINT ( 'NONE',  ( 15.79687500061451644, 0.000000000000000000, 4.756430356249998326 ) ) ;
#59683=LINE ( 'NONE', #71143, #29751 ) ;
#59687=VERTEX_POINT ( 'NONE', #13858 ) ;
#59693=CARTESIAN_POINT ( 'NONE',  ( 25.93125000122903145, 4.330127018922191873, 2.499999999999999556 ) ) ;
#59697=DIRECTION ( 'NONE',  ( -0.000000000000000000, -0.000000000000000000, -1.000000000000000000 ) ) ;
#59698=CARTESIAN_POINT ( 'NONE',  ( 18.08437500061451431, 4.119189519843966529, 2.378215178124999607 ) ) ;
#59711=CARTESIAN_POINT ( 'NONE',  ( 25.50000000000000000, 0.000000000000000000, 4.999999999999998224 ) ) ;
#59715=CARTESIAN_POINT ( 'NONE',  ( 28.93125000122903145, 6.123233995736764310E-16, -4.999999999999998224 ) ) ;
#59717=DIRECTION ( 'NONE',  ( -1.000000000000000000, -0.000000000000000000, -0.000000000000000000 ) ) ;
#59719=CARTESIAN_POINT ( 'NONE',  ( 8.400000000000000355, 0.000000000000000000, 4.999999999999998224 ) ) ;
#59739=VECTOR ( 'NONE', #29205, 1000.000000000000000 ) ;
#59740=CARTESIAN_POINT ( 'NONE',  ( 29.02499999999999858, 4.330127018922191873, 2.499999999999999556 ) ) ;
#59745=EDGE_CURVE ( 'NONE', #4778, #67289, #5029, .T. ) ;
#59759=CARTESIAN_POINT ( 'NONE',  ( 15.42187500061451466, -4.119189519843968306, 2.378215178124996054 ) ) ;
#59763=CARTESIAN_POINT ( 'NONE',  ( 24.94687500061451502, -4.119189519843965641, -2.378215178125001383 ) ) ;
#59773=FACE_OUTER_BOUND ( 'NONE', #67065, .T. ) ;
#59774=CARTESIAN_POINT ( 'NONE',  ( 12.63749999999999929, -2.886751345948125991, -5.000000000000000000 ) ) ;
#59781=CARTESIAN_POINT ( 'NONE',  ( 24.38437500061451502, 4.119189519843966529, 2.378215178124999607 ) ) ;
#59785=FACE_OUTER_BOUND ( 'NONE', #69668, .T. ) ;
#59791=CARTESIAN_POINT ( 'NONE',  ( 7.293750001229029500, -2.886751345948237457, -4.999999999999807265 ) ) ;
#59802=CARTESIAN_POINT ( 'NONE',  ( 9.234375000614518214, -4.119189519843968306, 2.378215178124996054 ) ) ;
#59815=CARTESIAN_POINT ( 'NONE',  ( 23.41875000122903216, -5.773502691896255534, -1.060575238724906372E-15 ) ) ;
#59817=VERTEX_POINT ( 'NONE', #31954 ) ;
#59820=CARTESIAN_POINT ( 'NONE',  ( 14.94375000122903252, -2.886751345948126435, -5.000000000000000000 ) ) ;
#59831=CARTESIAN_POINT ( 'NONE',  ( 15.15937500061451715, -4.119189519843965641, -2.378215178125001383 ) ) ;
#59836=AXIS2_PLACEMENT_3D ( 'NONE', #49767, #25766, #14665 ) ;
#59841=CARTESIAN_POINT ( 'NONE',  ( 15.33750000000000036, -2.886751345948125991, -5.000000000000000000 ) ) ;
#59852=( BOUNDED_CURVE ( )  B_SPLINE_CURVE ( 2, ( #9735, #38168, #4571, #60692, #10105, #27101, #21539 ),
 .UNSPECIFIED., .F., .F. ) 
 B_SPLINE_CURVE_WITH_KNOTS ( ( 3, 2, 2, 3 ),
 ( 0.01999999999999995878, 0.02333333333333328583, 0.02666666666666661634, 0.02999999999999993991 ),
 .UNSPECIFIED. ) 
 CURVE ( )  GEOMETRIC_REPRESENTATION_ITEM ( )  RATIONAL_B_SPLINE_CURVE ( ( 1.000000000000001554, 0.8660254037844370423, 1.000000000000000000, 0.8660254037844387076, 1.000000000000000000, 0.8660254037844410391, 0.9999999999999976685 ) ) 
 REPRESENTATION_ITEM ( '' )  );
#59854=CARTESIAN_POINT ( 'NONE',  ( 21.75937500061451502, -5.492252693125287522, -1.008910452111647106E-15 ) ) ;
#59867=CARTESIAN_POINT ( 'NONE',  ( 8.859375000614514661, 2.746126346562645981, -4.756430356249997438 ) ) ;
#59877=VERTEX_POINT ( 'NONE', #48219 ) ;
#59890=CARTESIAN_POINT ( 'NONE',  ( 20.67187500061451289, 2.746126346562645981, -4.756430356249997438 ) ) ;
#59922=CARTESIAN_POINT ( 'NONE',  ( 22.20937500061451431, 0.000000000000000000, 4.756430356249998326 ) ) ;
#59928=CARTESIAN_POINT ( 'NONE',  ( 21.93750000000000000, -2.886751345948129988, 4.999999999999997335 ) ) ;
#59935=CARTESIAN_POINT ( 'NONE',  ( 19.66875000122903216, 2.886751345948126879, 4.999999999999998224 ) ) ;
#59939=CARTESIAN_POINT ( 'NONE',  ( 8.118750001229033231, -5.773502691896255534, -1.060575238724906372E-15 ) ) ;
#59941=CARTESIAN_POINT ( 'NONE',  ( 15.19687500061451502, 4.119189519843966529, -2.378215178124998275 ) ) ;
#59947=FACE_OUTER_BOUND ( 'NONE', #5997, .T. ) ;
#59951=CARTESIAN_POINT ( 'NONE',  ( 8.971875000614515372, 4.119189519843966529, 2.378215178124999607 ) ) ;
#59962=ORIENTED_EDGE ( 'NONE', *, *, #51187, .F. ) ;
#59972=CARTESIAN_POINT ( 'NONE',  ( 26.10937500061451644, 4.119189519843966529, -2.378215178124998275 ) ) ;
#59974=CARTESIAN_POINT ( 'NONE',  ( 7.659375000614518036, 4.119189519843966529, -2.378215178124998275 ) ) ;
#59983=DIRECTION ( 'NONE',  ( -1.000000000000000000, -0.000000000000000000, -0.000000000000000000 ) ) ;
#59991=CARTESIAN_POINT ( 'NONE',  ( 20.75625000122903430, -4.330127018922190985, -2.500000000000001332 ) ) ;
#59999=CARTESIAN_POINT ( 'NONE',  ( 20.92500000000000071, 4.330127018922191873, 2.499999999999999556 ) ) ;
#60007=CARTESIAN_POINT ( 'NONE',  ( 28.84687500061452070, 5.492252693125287522, 3.363034840372157021E-16 ) ) ;
#60032=EDGE_CURVE ( 'NONE', #10316, #52965, #67814, .T. ) ;
#60039=ORIENTED_EDGE ( 'NONE', *, *, #5795, .F. ) ;
#60043=CARTESIAN_POINT ( 'NONE',  ( 14.44687500061451502, 0.000000000000000000, 4.756430356249998326 ) ) ;
#60054=CARTESIAN_POINT ( 'NONE',  ( 45.00000000000000000, -2.499999999999999556, 3.499999999999999556 ) ) ;
#60058=CARTESIAN_POINT ( 'NONE',  ( 14.06249999999999467, 2.886751345948018077, -5.000000000000190070 ) ) ;
#60062=CARTESIAN_POINT ( 'NONE',  ( 15.68437500061451573, 5.824947211148865298E-16, -4.756430356249998326 ) ) ;
#60072=DIRECTION ( 'NONE',  ( 0.000000000000000000, 0.000000000000000000, 1.000000000000000000 ) ) ;
#60075=CARTESIAN_POINT ( 'NONE',  ( 24.65625000122903288, 0.000000000000000000, 4.999999999999998224 ) ) ;
#60079=CARTESIAN_POINT ( 'NONE',  ( 27.99375000122903501, -2.886751345948125991, -5.000000000000000000 ) ) ;
#60083=CARTESIAN_POINT ( 'NONE',  ( -4.999999999999996447, 2.928932188134524051, 4.999999999999996447 ) ) ;
#60087=( BOUNDED_CURVE ( )  B_SPLINE_CURVE ( 2, ( #73086, #22467, #49832, #55372, #45018, #67553, #39471 ),
 .UNSPECIFIED., .F., .F. ) 
 B_SPLINE_CURVE_WITH_KNOTS ( ( 3, 2, 2, 3 ),
 ( 0.5100000000000000089, 0.5133333333333333082, 0.5166666666666667185, 0.5200000000000000178 ),
 .UNSPECIFIED. ) 
 CURVE ( )  GEOMETRIC_REPRESENTATION_ITEM ( )  RATIONAL_B_SPLINE_CURVE ( ( 1.000000000000000000, 0.8660254037844387076, 1.000000000000000000, 0.8660254037844387076, 1.000000000000000000, 0.8660254037844387076, 1.000000000000000000 ) ) 
 REPRESENTATION_ITEM ( '' )  );
#60096=FACE_OUTER_BOUND ( 'NONE', #6130, .T. ) ;
#60105=CARTESIAN_POINT ( 'NONE',  ( 26.66250000000000142, 2.886751345948129099, -4.999999999999998224 ) ) ;
#60110=CARTESIAN_POINT ( 'NONE',  ( 12.63749999999999574, -2.886751345948181946, -4.999999999999904077 ) ) ;
#60114=CARTESIAN_POINT ( 'NONE',  ( 22.46250000000000213, -5.773502691896255534, -1.060575238724906372E-15 ) ) ;
#60122=EDGE_CURVE ( 'NONE', #40700, #51146, #52682, .T. ) ;
#60124=ORIENTED_EDGE ( 'NONE', *, *, #41327, .T. ) ;
#60127=CARTESIAN_POINT ( 'NONE',  ( 21.72187500061451715, -4.119189519843968306, 2.378215178124996054 ) ) ;
#60136=CARTESIAN_POINT ( 'NONE',  ( 13.46249999999999858, -5.773502691896255534, -1.060575238724906372E-15 ) ) ;
#60143=CARTESIAN_POINT ( 'NONE',  ( 25.65937500061451715, 4.119189519843966529, -2.378215178124998275 ) ) ;
#60146=( NAMED_UNIT ( * ) PLANE_ANGLE_UNIT ( ) SI_UNIT ( $, .RADIAN. ) );
#60154=VERTEX_POINT ( 'NONE', #25307 ) ;
#60164=CARTESIAN_POINT ( 'NONE',  ( 10.43437500061451750, 4.119189519843966529, 2.378215178124999607 ) ) ;
#60180=CARTESIAN_POINT ( 'NONE',  ( 16.23750000000000071, -2.886751345948237457, -4.999999999999807265 ) ) ;
#60191=CARTESIAN_POINT ( 'NONE',  ( 10.73437500061451644, 5.824947211148865298E-16, -4.756430356249998326 ) ) ;
#60206=CARTESIAN_POINT ( 'NONE',  ( 9.299999999999998934, 0.000000000000000000, 4.999999999999998224 ) ) ;
#60210=CARTESIAN_POINT ( 'NONE',  ( 20.93437500061451217, -2.746126346562642428, -4.756430356249999214 ) ) ;
#60223=CARTESIAN_POINT ( 'NONE',  ( 9.309375000614515727, 2.746126346562645981, -4.756430356249997438 ) ) ;
#60230=CARTESIAN_POINT ( 'NONE',  ( 14.66249999999999964, 2.886751345948182834, 4.999999999999902300 ) ) ;
#60232=CARTESIAN_POINT ( 'NONE',  ( 15.03749999999999964, 5.773502691896255534, 3.535250795749688401E-16 ) ) ;
#60234=EDGE_LOOP ( 'NONE', ( #38244, #11264, #43054, #53840 ) ) ;
#60246=CARTESIAN_POINT ( 'NONE',  ( 18.19687500061451502, -2.746126346562646425, 4.756430356249996549 ) ) ;
#60250=EDGE_LOOP ( 'NONE', ( #64733, #58813, #27850, #26225 ) ) ;
#60274=ORIENTED_EDGE ( 'NONE', *, *, #59537, .T. ) ;
#60278=CARTESIAN_POINT ( 'NONE',  ( 20.85937500061451644, 0.000000000000000000, 4.756430356249998326 ) ) ;
#60282=( BOUNDED_CURVE ( )  B_SPLINE_CURVE ( 2, ( #39011, #50094, #61170, #45644, #28640, #68177, #17540 ),
 .UNSPECIFIED., .F., .F. ) 
 B_SPLINE_CURVE_WITH_KNOTS ( ( 3, 2, 2, 3 ),
 ( 0.3099999999999999978, 0.3133333333333333526, 0.3166666666666665964, 0.3199999999999999512 ),
 .UNSPECIFIED. ) 
 CURVE ( )  GEOMETRIC_REPRESENTATION_ITEM ( )  RATIONAL_B_SPLINE_CURVE ( ( 1.000000000000000000, 0.8660254037844387076, 1.000000000000000000, 0.8660254037844387076, 1.000000000000000000, 0.8660254037844409281, 0.9999999999999977796 ) ) 
 REPRESENTATION_ITEM ( '' )  );
#60285=CARTESIAN_POINT ( 'NONE',  ( 23.13749999999999929, 5.773502691896255534, 3.535250795749688894E-16 ) ) ;
#60288=CARTESIAN_POINT ( 'NONE',  ( 34.99999999999999289, -2.499999999999999556, 3.499999999999999556 ) ) ;
#60289=CARTESIAN_POINT ( 'NONE',  ( 22.63125000122903430, 6.123233995736764310E-16, -4.999999999999998224 ) ) ;
#60291=CARTESIAN_POINT ( 'NONE',  ( 18.69375000122903430, 5.773502691896255534, 3.535250795749688401E-16 ) ) ;
#60296=CARTESIAN_POINT ( 'NONE',  ( 28.92187500061451644, -4.119189519843968306, 2.378215178124996054 ) ) ;
#60298=CARTESIAN_POINT ( 'NONE',  ( 13.58437500061451431, -2.746126346562646425, 4.756430356249996549 ) ) ;
#60308=CARTESIAN_POINT ( 'NONE',  ( 45.00000000000000000, 0.000000000000000000, 4.999999999999998224 ) ) ;
#60309=CARTESIAN_POINT ( 'NONE',  ( 9.196875000614515017, -4.119189519843965641, -2.378215178125001383 ) ) ;
#60311=VERTEX_POINT ( 'NONE', #38966 ) ;
#60333=CARTESIAN_POINT ( 'NONE',  ( 25.05937500061451573, -4.119189519843965641, -2.378215178125001383 ) ) ;
#60335=CARTESIAN_POINT ( 'NONE',  ( 9.009375000614518569, 4.119189519843966529, -2.378215178124998275 ) ) ;
#60352=CARTESIAN_POINT ( 'NONE',  ( 17.49375000122903145, -2.886751345948129988, 4.999999999999997335 ) ) ;
#60368=CARTESIAN_POINT ( 'NONE',  ( 28.95937500061451431, 0.000000000000000000, 4.756430356249998326 ) ) ;
#60374=VECTOR ( 'NONE', #71468, 1000.000000000000000 ) ;
#60381=CARTESIAN_POINT ( 'NONE',  ( 27.63749999999999929, 5.773502691896255534, 3.535250795749688401E-16 ) ) ;
#60387=CARTESIAN_POINT ( 'NONE',  ( 21.64687500061451431, 0.000000000000000000, 4.756430356249998326 ) ) ;
#60390=ORIENTED_EDGE ( 'NONE', *, *, #8224, .T. ) ;
#60405=CARTESIAN_POINT ( 'NONE',  ( 15.30937500061451573, 2.746126346562643317, 4.756430356249998326 ) ) ;
#60419=CARTESIAN_POINT ( 'NONE',  ( 9.431250001229033231, -4.330127018922194537, 2.499999999999995559 ) ) ;
#60424=CARTESIAN_POINT ( 'NONE',  ( 16.24687500061451573, 5.492252693125287522, 3.363034840372157021E-16 ) ) ;
#60433=VECTOR ( 'NONE', #40023, 1000.000000000000000 ) ;
#60435=CARTESIAN_POINT ( 'NONE',  ( 12.99375000122903323, -2.886751345948130876, 4.999999999999996447 ) ) ;
#60438=CARTESIAN_POINT ( 'NONE',  ( 25.64999999999999858, -4.330127018922190985, -2.500000000000001332 ) ) ;
#60442=CARTESIAN_POINT ( 'NONE',  ( 24.99375000122903145, 5.773502691896255534, 3.535250795749688894E-16 ) ) ;
#60445=EDGE_CURVE ( 'NONE', #34725, #28470, #47953, .T. ) ;
#60474=VECTOR ( 'NONE', #5169, 1000.000000000000000 ) ;
#60478=CARTESIAN_POINT ( 'NONE',  ( 27.39375000122904069, -2.886751345948157965, 4.999999999999948486 ) ) ;
#60482=( BOUNDED_CURVE ( )  B_SPLINE_CURVE ( 2, ( #6195, #56085, #67182, #50544, #33899, #17268, #12100 ),
 .UNSPECIFIED., .F., .F. ) 
 B_SPLINE_CURVE_WITH_KNOTS ( ( 3, 2, 2, 3 ),
 ( 0.7600000000000000089, 0.7633333333333333082, 0.7666666666666668295, 0.7700000000000001288 ),
 .UNSPECIFIED. ) 
 CURVE ( )  GEOMETRIC_REPRESENTATION_ITEM ( )  RATIONAL_B_SPLINE_CURVE ( ( 1.000000000000000000, 0.8660254037844387076, 1.000000000000000000, 0.8660254037844387076, 1.000000000000000000, 0.8660254037844342667, 1.000000000000004441 ) ) 
 REPRESENTATION_ITEM ( '' )  );
#60491=CARTESIAN_POINT ( 'NONE',  ( 22.43437500061451217, 5.492252693125287522, 3.363034840372157021E-16 ) ) ;
#60501=CARTESIAN_POINT ( 'NONE',  ( 12.48750000000000249, -2.886751345948129988, 4.999999999999997335 ) ) ;
#60508=CARTESIAN_POINT ( 'NONE',  ( 23.25937500061451857, -4.119189519843965641, -2.378215178125001383 ) ) ;
#60512=DIRECTION ( 'NONE',  ( -1.000000000000000000, -0.000000000000000000, -0.000000000000000000 ) ) ;
#60519=CARTESIAN_POINT ( 'NONE',  ( 45.00000000000000000, 6.123233995736764310E-16, -4.999999999999998224 ) ) ;
#60531=CARTESIAN_POINT ( 'NONE',  ( 9.871875000614517504, 2.746126346562645981, -4.756430356249997438 ) ) ;
#60556=CARTESIAN_POINT ( 'NONE',  ( 11.89687500061451608, -2.746126346562646425, 4.756430356249996549 ) ) ;
#60571=CARTESIAN_POINT ( 'NONE',  ( 19.53749999999999432, 5.773502691896255534, 3.535250795749688401E-16 ) ) ;
#60577=CARTESIAN_POINT ( 'NONE',  ( 20.07187500061451502, 5.824947211148865298E-16, -4.756430356249998326 ) ) ;
#60580=CARTESIAN_POINT ( 'NONE',  ( 13.18125000122903323, 6.123233995736764310E-16, -4.999999999999998224 ) ) ;
#60593=CARTESIAN_POINT ( 'NONE',  ( 29.14687500061451075, -2.746126346562642428, -4.756430356249999214 ) ) ;
#60614=CARTESIAN_POINT ( 'NONE',  ( 17.03437500061451715, 5.824947211148865298E-16, -4.756430356249998326 ) ) ;
#60628=ORIENTED_EDGE ( 'NONE', *, *, #27801, .T. ) ;
#60645=CARTESIAN_POINT ( 'NONE',  ( 17.59687500061451715, 5.492252693125287522, 3.363034840372157021E-16 ) ) ;
#60652=CARTESIAN_POINT ( 'NONE',  ( 21.67500000000000071, 6.123233995736764310E-16, -4.999999999999998224 ) ) ;
#60655=CARTESIAN_POINT ( 'NONE',  ( 19.03125000122902932, 6.123233995736764310E-16, -4.999999999999998224 ) ) ;
#60664=CARTESIAN_POINT ( 'NONE',  ( 26.48437500061450933, 5.492252693125287522, 3.363034840372157021E-16 ) ) ;
#60666=CARTESIAN_POINT ( 'NONE',  ( 13.02187500061451786, 4.119189519843966529, 2.378215178124999607 ) ) ;
#60669=VERTEX_POINT ( 'NONE', #23760 ) ;
#60672=FACE_OUTER_BOUND ( 'NONE', #17276, .T. ) ;
#60689=AXIS2_PLACEMENT_3D ( 'NONE', #8602, #25214, #1618 ) ;
#60692=CARTESIAN_POINT ( 'NONE',  ( 29.43750000000000000, 5.773502691896255534, 3.535250795749688401E-16 ) ) ;
#60699=CARTESIAN_POINT ( 'NONE',  ( 25.09687500061451715, -2.746126346562641984, -4.756430356249999214 ) ) ;
#60701=CARTESIAN_POINT ( 'NONE',  ( 9.121875000614517504, 2.746126346562643317, 4.756430356249998326 ) ) ;
#60717=VECTOR ( 'NONE', #64379, 1000.000000000000000 ) ;
#60721=CARTESIAN_POINT ( 'NONE',  ( 18.39375000122903003, -2.886751345948129988, 4.999999999999997335 ) ) ;
#60729=CARTESIAN_POINT ( 'NONE',  ( 20.96250000000000213, 2.886751345948154857, 4.999999999999951150 ) ) ;
#60731=( BOUNDED_CURVE ( )  B_SPLINE_CURVE ( 2, ( #4309, #65983, #31642, #70792, #26834, #14269, #66349 ),
 .UNSPECIFIED., .F., .F. ) 
 B_SPLINE_CURVE_WITH_KNOTS ( ( 3, 2, 2, 3 ),
 ( 0.1099999999999999312, 0.1133333333333333137, 0.1166666666666666963, 0.1200000000000000788 ),
 .UNSPECIFIED. ) 
 CURVE ( )  GEOMETRIC_REPRESENTATION_ITEM ( )  RATIONAL_B_SPLINE_CURVE ( ( 1.000000000000002887, 0.8660254037844359321, 1.000000000000000000, 0.8660254037844387076, 1.000000000000000000, 0.8660254037844353769, 1.000000000000003331 ) ) 
 REPRESENTATION_ITEM ( '' )  );
#60738=CARTESIAN_POINT ( 'NONE',  ( 27.08437500061451786, 4.119189519843966529, 2.378215178124999607 ) ) ;
#60755=CARTESIAN_POINT ( 'NONE',  ( 12.16875000122903394, -5.773502691896255534, -1.060575238724906372E-15 ) ) ;
#60759=CARTESIAN_POINT ( 'NONE',  ( 21.53437500061451715, 5.492252693125287522, 3.363034840372157021E-16 ) ) ;
#60764=CARTESIAN_POINT ( 'NONE',  ( 10.63125000122903252, 4.330127018922191873, 2.499999999999999556 ) ) ;
#60770=ORIENTED_EDGE ( 'NONE', *, *, #9282, .F. ) ;
#60776=CARTESIAN_POINT ( 'NONE',  ( 12.33750000000000213, 5.773502691896255534, 3.535250795749688401E-16 ) ) ;
#60777=CARTESIAN_POINT ( 'NONE',  ( 13.95937500061451608, 2.746126346562643317, 4.756430356249998326 ) ) ;
#60784=ORIENTED_EDGE ( 'NONE', *, *, #44946, .F. ) ;
#60795=CARTESIAN_POINT ( 'NONE',  ( 14.07187500061451679, 2.746126346562643317, 4.756430356249998326 ) ) ;
#60801=CARTESIAN_POINT ( 'NONE',  ( 10.53750000000000320, 5.773502691896255534, 3.535250795749688401E-16 ) ) ;
#60808=CARTESIAN_POINT ( 'NONE',  ( 24.43125000122903145, 6.123233995736764310E-16, -4.999999999999998224 ) ) ;
#60812=CARTESIAN_POINT ( 'NONE',  ( 26.90625000122902932, 0.000000000000000000, 4.999999999999998224 ) ) ;
#60816=FACE_OUTER_BOUND ( 'NONE', #8496, .T. ) ;
#60851=AXIS2_PLACEMENT_3D ( 'NONE', #45869, #62845, #1172 ) ;
#60862=ORIENTED_EDGE ( 'NONE', *, *, #18371, .F. ) ;
#60865=CARTESIAN_POINT ( 'NONE',  ( 21.94687500061451146, 4.119189519843966529, -2.378215178124998275 ) ) ;
#60872=CARTESIAN_POINT ( 'NONE',  ( 26.84999999999999787, 0.000000000000000000, 4.999999999999998224 ) ) ;
#60874=CARTESIAN_POINT ( 'NONE',  ( 12.07499999999999929, -4.330127018922194537, 2.499999999999995559 ) ) ;
#60881=CARTESIAN_POINT ( 'NONE',  ( 21.79687500061451644, -2.746126346562646425, 4.756430356249996549 ) ) ;
#60903=CARTESIAN_POINT ( 'NONE',  ( 10.99687500061451928, -2.746126346562646425, 4.756430356249996549 ) ) ;
#60915=DIRECTION ( 'NONE',  ( 1.000000000000000000, -0.000000000000000000, -0.000000000000000000 ) ) ;
#60924=ORIENTED_EDGE ( 'NONE', *, *, #17853, .T. ) ;
#60926=CARTESIAN_POINT ( 'NONE',  ( 10.62187500061451928, -5.492252693125287522, -1.008910452111647106E-15 ) ) ;
#60936=FACE_OUTER_BOUND ( 'NONE', #22251, .T. ) ;
#60937=AXIS2_PLACEMENT_3D ( 'NONE', #50575, #11773, #72740 ) ;
#60942=CARTESIAN_POINT ( 'NONE',  ( 19.46250000000000213, 2.886751345948045611, -5.000000000000141220 ) ) ;
#60948=CARTESIAN_POINT ( 'NONE',  ( 19.50937500061451857, -5.492252693125287522, -1.008910452111647106E-15 ) ) ;
#60951=CARTESIAN_POINT ( 'NONE',  ( 14.45625000122903359, -4.330127018922190985, -2.500000000000001332 ) ) ;
#60960=CARTESIAN_POINT ( 'NONE',  ( 10.70625000122903536, 0.000000000000000000, 4.999999999999998224 ) ) ;
#60969=CARTESIAN_POINT ( 'NONE',  ( 28.88437500061451502, 4.119189519843966529, 2.378215178124999607 ) ) ;
#60974=DIRECTION ( 'NONE',  ( -1.000000000000000000, -0.000000000000000000, -0.000000000000000000 ) ) ;
#60991=CARTESIAN_POINT ( 'NONE',  ( 17.07187500061451502, 2.746126346562645981, -4.756430356249997438 ) ) ;
#61022=VERTEX_POINT ( 'NONE', #71396 ) ;
#61025=CARTESIAN_POINT ( 'NONE',  ( 18.19687500061451502, -2.746126346562646425, 4.756430356249996549 ) ) ;
#61031=CARTESIAN_POINT ( 'NONE',  ( 19.94999999999999929, 4.330127018922192761, -2.499999999999997780 ) ) ;
#61041=CARTESIAN_POINT ( 'NONE',  ( 27.57187500061451502, -4.119189519843968306, 2.378215178124996054 ) ) ;
#61043=CARTESIAN_POINT ( 'NONE',  ( 12.64687500061451786, 0.000000000000000000, 4.756430356249998326 ) ) ;
#61060=EDGE_LOOP ( 'NONE', ( #4740, #58111, #55660, #41765 ) ) ;
#61068=ORIENTED_EDGE ( 'NONE', *, *, #28164, .F. ) ;
#61077=CARTESIAN_POINT ( 'NONE',  ( 24.57187500061451502, -5.492252693125287522, -1.008910452111647106E-15 ) ) ;
#61079=CARTESIAN_POINT ( 'NONE',  ( 8.821875000614518569, -5.492252693125287522, -1.008910452111647106E-15 ) ) ;
#61098=CARTESIAN_POINT ( 'NONE',  ( 19.44375000122903430, -2.886751345948125991, -5.000000000000000000 ) ) ;
#61101=ORIENTED_EDGE ( 'NONE', *, *, #26912, .T. ) ;
#61108=DIRECTION ( 'NONE',  ( -1.000000000000000000, -0.000000000000000000, -0.000000000000000000 ) ) ;
#61116=CARTESIAN_POINT ( 'NONE',  ( 26.10937500061451644, 4.119189519843966529, -2.378215178124998275 ) ) ;
#61129=CARTESIAN_POINT ( 'NONE',  ( 27.52500000000000213, 6.123233995736764310E-16, -4.999999999999998224 ) ) ;
#61131=CARTESIAN_POINT ( 'NONE',  ( 11.30625000122903501, -4.330127018922190985, -2.500000000000001332 ) ) ;
#61133=CARTESIAN_POINT ( 'NONE',  ( 20.82187500061451502, -4.119189519843968306, 2.378215178124996054 ) ) ;
#61141=VECTOR ( 'NONE', #19583, 1000.000000000000000 ) ;
#61145=CARTESIAN_POINT ( 'NONE',  ( 13.02187500061451786, 4.119189519843966529, 2.378215178124999607 ) ) ;
#61154=CARTESIAN_POINT ( 'NONE',  ( 14.25937500061451679, 2.746126346562645981, -4.756430356249997438 ) ) ;
#61170=CARTESIAN_POINT ( 'NONE',  ( 22.55625000122903145, -4.330127018922190985, -2.500000000000001332 ) ) ;
#61171=CARTESIAN_POINT ( 'NONE',  ( 15.45937500061451608, 0.000000000000000000, 4.756430356249998326 ) ) ;
#61180=( BOUNDED_CURVE ( )  B_SPLINE_CURVE ( 2, ( #69223, #905, #17503, #18584, #40417, #7513, #52584 ),
 .UNSPECIFIED., .F., .F. ) 
 B_SPLINE_CURVE_WITH_KNOTS ( ( 3, 2, 2, 3 ),
 ( 0.9300000000000001599, 0.9333333333333334592, 0.9366666666666668695, 0.9400000000000001688 ),
 .UNSPECIFIED. ) 
 CURVE ( )  GEOMETRIC_REPRESENTATION_ITEM ( )  RATIONAL_B_SPLINE_CURVE ( ( 0.9999999999999955591, 0.8660254037844431485, 1.000000000000000000, 0.8660254037844387076, 1.000000000000000000, 0.8660254037844298258, 1.000000000000008882 ) ) 
 REPRESENTATION_ITEM ( '' )  );
#61190=EDGE_CURVE ( 'NONE', #22800, #24417, #38028, .T. ) ;
#61191=CARTESIAN_POINT ( 'NONE',  ( 25.85625000122903216, 4.330127018922192761, -2.499999999999997780 ) ) ;
#61202=CARTESIAN_POINT ( 'NONE',  ( 10.36875000122903323, -5.773502691896255534, -1.060575238724906372E-15 ) ) ;
#61234=ORIENTED_EDGE ( 'NONE', *, *, #47659, .T. ) ;
#61237=CARTESIAN_POINT ( 'NONE',  ( 21.64687500061451431, 0.000000000000000000, 4.756430356249998326 ) ) ;
#61245=ORIENTED_EDGE ( 'NONE', *, *, #34819, .F. ) ;
#61246=CARTESIAN_POINT ( 'NONE',  ( 9.899999999999998579, -4.330127018922190985, -2.500000000000001332 ) ) ;
#61253=CARTESIAN_POINT ( 'NONE',  ( 22.69687500061451857, -2.746126346562646425, 4.756430356249996549 ) ) ;
#61263=CARTESIAN_POINT ( 'NONE',  ( -5.000000000000004441, 6.123233995736764310E-16, -4.999999999999998224 ) ) ;
#61276=CARTESIAN_POINT ( 'NONE',  ( 9.309375000614517504, -4.119189519843965641, -2.378215178125001383 ) ) ;
#61283=VERTEX_POINT ( 'NONE', #3062 ) ;
#61284=VERTEX_POINT ( 'NONE', #1083 ) ;
#61297=CARTESIAN_POINT ( 'NONE',  ( 10.39687500061451786, 5.492252693125287522, 3.363034840372157021E-16 ) ) ;
#61298=DIRECTION ( 'NONE',  ( -1.000000000000000000, -0.000000000000000000, -0.000000000000000000 ) ) ;
#61316=CARTESIAN_POINT ( 'NONE',  ( 21.27187500061451431, -4.119189519843968306, 2.378215178124996054 ) ) ;
#61319=CARTESIAN_POINT ( 'NONE',  ( 15.35625000122903216, -4.330127018922190985, -2.500000000000001332 ) ) ;
#61333=CARTESIAN_POINT ( 'NONE',  ( 7.284375000614517148, -2.746126346562646425, 4.756430356249996549 ) ) ;
#61339=CARTESIAN_POINT ( 'NONE',  ( 45.00000000000000000, 0.000000000000000000, 4.999999999999998224 ) ) ;
#61341=CARTESIAN_POINT ( 'NONE',  ( 15.00000000000000000, 4.330127018922192761, -2.499999999999997780 ) ) ;
#61343=ORIENTED_EDGE ( 'NONE', *, *, #65260, .F. ) ;
#61355=CARTESIAN_POINT ( 'NONE',  ( 18.15937500061451715, 0.000000000000000000, 4.756430356249998326 ) ) ;
#61359=ORIENTED_EDGE ( 'NONE', *, *, #16377, .F. ) ;
#61369=ORIENTED_EDGE ( 'NONE', *, *, #39433, .T. ) ;
#61377=( BOUNDED_CURVE ( )  B_SPLINE_CURVE ( 2, ( #63586, #18867, #46971, #1186, #63223, #52869, #24422 ),
 .UNSPECIFIED., .F., .F. ) 
 B_SPLINE_CURVE_WITH_KNOTS ( ( 3, 2, 2, 3 ),
 ( 0.4700000000000001399, 0.4733333333333334392, 0.4766666666666666829, 0.4799999999999999267 ),
 .UNSPECIFIED. ) 
 CURVE ( )  GEOMETRIC_REPRESENTATION_ITEM ( )  RATIONAL_B_SPLINE_CURVE ( ( 0.9999999999999933387, 0.8660254037844453689, 1.000000000000000000, 0.8660254037844387076, 1.000000000000000000, 0.8660254037844409281, 0.9999999999999977796 ) ) 
 REPRESENTATION_ITEM ( '' )  );
#61387=CARTESIAN_POINT ( 'NONE',  ( 18.08437500061451431, 4.119189519843966529, 2.378215178124999607 ) ) ;
#61395=CARTESIAN_POINT ( 'NONE',  ( 20.17499999999999716, -4.330127018922194537, 2.499999999999995559 ) ) ;
#61398=CARTESIAN_POINT ( 'NONE',  ( 26.25937500061451502, -5.492252693125287522, -1.008910452111647106E-15 ) ) ;
#61401=CARTESIAN_POINT ( 'NONE',  ( 17.39999999999999858, 0.000000000000000000, 4.999999999999998224 ) ) ;
#61404=CARTESIAN_POINT ( 'NONE',  ( 28.05937500061451217, -5.492252693125287522, -1.008910452111647106E-15 ) ) ;
#61407=CARTESIAN_POINT ( 'NONE',  ( 13.05937500061451750, 2.746126346562643317, 4.756430356249998326 ) ) ;
#61410=ORIENTED_EDGE ( 'NONE', *, *, #46133, .T. ) ;
#61418=CARTESIAN_POINT ( 'NONE',  ( 18.75000000000000000, 0.000000000000000000, 4.999999999999998224 ) ) ;
#61419=VERTEX_POINT ( 'NONE', #16955 ) ;
#61440=CARTESIAN_POINT ( 'NONE',  ( 23.63437500061451502, -4.119189519843968306, 2.378215178124996054 ) ) ;
#61442=CARTESIAN_POINT ( 'NONE',  ( 8.146875000614516082, 5.492252693125287522, 3.363034840372157021E-16 ) ) ;
#61459=CARTESIAN_POINT ( 'NONE',  ( 18.13125000122903074, 6.123233995736764310E-16, -4.999999999999998224 ) ) ;
#61462=ORIENTED_EDGE ( 'NONE', *, *, #71351, .T. ) ;
#61475=CARTESIAN_POINT ( 'NONE',  ( 26.18437500061451573, 4.119189519843966529, 2.378215178124999607 ) ) ;
#61481=CARTESIAN_POINT ( 'NONE',  ( 27.89999999999999858, -4.330127018922190985, -2.500000000000001332 ) ) ;
#61487=CARTESIAN_POINT ( 'NONE',  ( 8.775000000000002132, 4.330127018922191873, 2.499999999999999556 ) ) ;
#61489=CARTESIAN_POINT ( 'NONE',  ( 12.88125000122903430, 4.330127018922191873, 2.499999999999999556 ) ) ;
#61493=CARTESIAN_POINT ( 'NONE',  ( 20.59687500061451715, 4.119189519843966529, -2.378215178124998275 ) ) ;
#61503=CARTESIAN_POINT ( 'NONE',  ( 12.60937500061451289, 2.746126346562643317, 4.756430356249998326 ) ) ;
#61509=ORIENTED_EDGE ( 'NONE', *, *, #72508, .F. ) ;
#61517=ORIENTED_EDGE ( 'NONE', *, *, #41396, .F. ) ;
#61524=CARTESIAN_POINT ( 'NONE',  ( 16.94999999999999929, 0.000000000000000000, 4.999999999999998224 ) ) ;
#61527=CARTESIAN_POINT ( 'NONE',  ( 14.89687500061451786, 5.492252693125287522, 3.363034840372157021E-16 ) ) ;
#61537=CARTESIAN_POINT ( 'NONE',  ( 12.90000000000000213, 0.000000000000000000, 4.999999999999998224 ) ) ;
#61544=CARTESIAN_POINT ( 'NONE',  ( 24.84375000122903288, -2.886751345948125991, -5.000000000000000000 ) ) ;
#61556=DIRECTION ( 'NONE',  ( -1.000000000000000000, -0.000000000000000000, -0.000000000000000000 ) ) ;
#61575=CARTESIAN_POINT ( 'NONE',  ( 26.23125000122903216, 6.123233995736764310E-16, -4.999999999999998224 ) ) ;
#61592=CARTESIAN_POINT ( 'NONE',  ( 21.53437500061451360, 5.492252693125287522, 3.363034840372157021E-16 ) ) ;
#61603=CARTESIAN_POINT ( 'NONE',  ( 11.70000000000000284, -4.330127018922190985, -2.500000000000001332 ) ) ;
#61610=CARTESIAN_POINT ( 'NONE',  ( 23.48437500061451644, 4.119189519843966529, 2.378215178124999607 ) ) ;
#61640=DIRECTION ( 'NONE',  ( -1.000000000000000000, -0.000000000000000000, -0.000000000000000000 ) ) ;
#61647=ORIENTED_EDGE ( 'NONE', *, *, #27131, .F. ) ;
#61653=CARTESIAN_POINT ( 'NONE',  ( 12.15937500061451892, 4.119189519843966529, -2.378215178124998275 ) ) ;
#61664=FACE_OUTER_BOUND ( 'NONE', #65579, .T. ) ;
#61669=LINE ( 'NONE', #38795, #60474 ) ;
#61674=CARTESIAN_POINT ( 'NONE',  ( 20.14687500061451786, 4.119189519843966529, -2.378215178124998275 ) ) ;
#61677=CARTESIAN_POINT ( 'NONE',  ( 13.66875000122903216, 2.886751345948129099, -4.999999999999998224 ) ) ;
#61683=CARTESIAN_POINT ( 'NONE',  ( 21.15000000000000213, -4.330127018922190985, -2.500000000000001332 ) ) ;
#61685=FACE_OUTER_BOUND ( 'NONE', #36642, .T. ) ;
#61692=CARTESIAN_POINT ( 'NONE',  ( 28.99687500061451573, -2.746126346562646425, 4.756430356249996549 ) ) ;
#61700=CARTESIAN_POINT ( 'NONE',  ( 45.00000000000000000, 0.000000000000000000, 0.000000000000000000 ) ) ;
#61702=ORIENTED_EDGE ( 'NONE', *, *, #4530, .F. ) ;
#61714=CARTESIAN_POINT ( 'NONE',  ( 16.20937500061451786, 4.119189519843966529, -2.378215178124998275 ) ) ;
#61742=VERTEX_POINT ( 'NONE', #38968 ) ;
#61745=CARTESIAN_POINT ( 'NONE',  ( 19.43437500061451928, 4.119189519843966529, 2.378215178124999607 ) ) ;
#61752=CARTESIAN_POINT ( 'NONE',  ( 19.01249999999999929, 2.886751345948129099, -4.999999999999998224 ) ) ;
#61756=CARTESIAN_POINT ( 'NONE',  ( 24.90937500061451360, -5.492252693125287522, -1.008910452111647106E-15 ) ) ;
#61763=CARTESIAN_POINT ( 'NONE',  ( 26.29687500061451644, -4.119189519843965641, -2.378215178125001383 ) ) ;
#61765=CARTESIAN_POINT ( 'NONE',  ( 13.69687500061451679, -4.119189519843965641, -2.378215178125001383 ) ) ;
#61776=EDGE_LOOP ( 'NONE', ( #36781, #35105, #64546, #38106 ) ) ;
#61800=CARTESIAN_POINT ( 'NONE',  ( 24.42187500061451644, 2.746126346562643317, 4.756430356249998326 ) ) ;
#61808=CARTESIAN_POINT ( 'NONE',  ( 19.94999999999999929, 4.330127018922192761, -2.499999999999997780 ) ) ;
#61819=CARTESIAN_POINT ( 'NONE',  ( 18.20625000122903003, 4.330127018922192761, -2.499999999999997780 ) ) ;
#61836=CARTESIAN_POINT ( 'NONE',  ( 25.99687500061451928, -2.746126346562642428, -4.756430356249999214 ) ) ;
#61842=CARTESIAN_POINT ( 'NONE',  ( 26.77499999999999858, 4.330127018922191873, 2.499999999999999556 ) ) ;
#61850=CARTESIAN_POINT ( 'NONE',  ( 12.69375000122903430, -2.886751345948125991, -5.000000000000000000 ) ) ;
#61853=CARTESIAN_POINT ( 'NONE',  ( 19.95937500061451786, -5.492252693125287522, -1.008910452111647106E-15 ) ) ;
#61854=AXIS2_PLACEMENT_3D ( 'NONE', #52393, #12862, #23942 ) ;
#61860=CYLINDRICAL_SURFACE ( 'NONE', #339, 4.999999999999998224 ) ;
#61866=CARTESIAN_POINT ( 'NONE',  ( 12.23437500061451644, -2.746126346562646425, 4.756430356249996549 ) ) ;
#61873=ORIENTED_EDGE ( 'NONE', *, *, #2515, .F. ) ;
#61874=CARTESIAN_POINT ( 'NONE',  ( 19.16250000000000142, 2.886751345948098901, 5.000000000000047073 ) ) ;
#61880=VECTOR ( 'NONE', #58739, 1000.000000000000000 ) ;
#61892=CARTESIAN_POINT ( 'NONE',  ( 29.70937500061451431, 2.746126346562643317, 4.756430356249998326 ) ) ;
#61893=CARTESIAN_POINT ( 'NONE',  ( 12.08437500061451608, 5.824947211148865298E-16, -4.756430356249998326 ) ) ;
#61910=DIRECTION ( 'NONE',  ( 0.000000000000000000, 0.000000000000000000, 1.000000000000000000 ) ) ;
#61911=CARTESIAN_POINT ( 'NONE',  ( 26.64375000122903003, -2.886751345948125991, -5.000000000000000000 ) ) ;
#61928=ADVANCED_FACE ( 'NONE', ( #23761 ), #8238, .T. ) ;
#61950=CARTESIAN_POINT ( 'NONE',  ( 27.80625000122903145, 0.000000000000000000, 4.999999999999998224 ) ) ;
#61955=VERTEX_POINT ( 'NONE', #64380 ) ;
#61958=CARTESIAN_POINT ( 'NONE',  ( 19.99687500061451217, -4.119189519843965641, -2.378215178125001383 ) ) ;
#61961=VECTOR ( 'NONE', #25648, 1000.000000000000000 ) ;
#61968=VERTEX_POINT ( 'NONE', #12684 ) ;
#61975=CARTESIAN_POINT ( 'NONE',  ( 21.49687500061451573, -2.746126346562642428, -4.756430356249999214 ) ) ;
#61978=CARTESIAN_POINT ( 'NONE',  ( 20.24999999999999645, -4.330127018922190985, -2.500000000000001332 ) ) ;
#61983=AXIS2_PLACEMENT_3D ( 'NONE', #53038, #47870, #25700 ) ;
#61994=LINE ( 'NONE', #11394, #68084 ) ;
#61999=CARTESIAN_POINT ( 'NONE',  ( 7.621875000614519280, 2.746126346562645981, -4.756430356249997438 ) ) ;
#62023=CARTESIAN_POINT ( 'NONE',  ( 9.759375000614516793, -4.119189519843965641, -2.378215178125001383 ) ) ;
#62028=APPLICATION_CONTEXT ( 'automotive_design' ) ;
#62047=CARTESIAN_POINT ( 'NONE',  ( 18.68437500061451573, -2.746126346562642428, -4.756430356249999214 ) ) ;
#62050=CARTESIAN_POINT ( 'NONE',  ( 14.71875000122903465, 2.886751345948126879, 4.999999999999999112 ) ) ;
#62064=CARTESIAN_POINT ( 'NONE',  ( 7.584375000614516971, 5.492252693125287522, 3.363034840372157021E-16 ) ) ;
#62070=CARTESIAN_POINT ( 'NONE',  ( 24.88125000122903074, 6.123233995736764310E-16, -4.999999999999998224 ) ) ;
#62074=VECTOR ( 'NONE', #51292, 1000.000000000000000 ) ;
#62086=CARTESIAN_POINT ( 'NONE',  ( 15.04687500061451644, -2.746126346562646425, 4.756430356249996549 ) ) ;
#62104=EDGE_CURVE ( 'NONE', #9764, #1518, #31131, .T. ) ;
#62117=CARTESIAN_POINT ( 'NONE',  ( 17.85937500061451999, -4.119189519843965641, -2.378215178125001383 ) ) ;
#62123=CARTESIAN_POINT ( 'NONE',  ( 20.99999999999999645, 0.000000000000000000, 4.999999999999998224 ) ) ;
#62127=CARTESIAN_POINT ( 'NONE',  ( 24.87187500061451217, -4.119189519843968306, 2.378215178124996054 ) ) ;
#62134=CARTESIAN_POINT ( 'NONE',  ( 27.34687500061451360, 4.119189519843966529, -2.378215178124998275 ) ) ;
#62136=CARTESIAN_POINT ( 'NONE',  ( 10.88437500061451679, -2.746126346562646425, 4.756430356249996549 ) ) ;
#62145=LINE ( 'NONE', #28886, #1887 ) ;
#62155=FACE_OUTER_BOUND ( 'NONE', #15694, .T. ) ;
#62165=AXIS2_PLACEMENT_3D ( 'NONE', #42447, #60512, #30623 ) ;
#62172=CARTESIAN_POINT ( 'NONE',  ( 21.04687500061451644, -2.746126346562641984, -4.756430356249999214 ) ) ;
#62192=CARTESIAN_POINT ( 'NONE',  ( 16.06875000122903074, 2.886751345948126879, 4.999999999999999112 ) ) ;
#62207=CARTESIAN_POINT ( 'NONE',  ( 26.22187500061451715, 2.746126346562643317, 4.756430356249998326 ) ) ;
#62210=EDGE_CURVE ( 'NONE', #38121, #38724, #57433, .T. ) ;
#62213=CARTESIAN_POINT ( 'NONE',  ( 26.06250000000000000, -5.773502691896255534, -1.060575238724906372E-15 ) ) ;
#62221=CARTESIAN_POINT ( 'NONE',  ( 11.86875000122903145, 2.886751345948129099, -4.999999999999998224 ) ) ;
#62225=CARTESIAN_POINT ( 'NONE',  ( 19.13437500061451857, -2.746126346562641984, -4.756430356249999214 ) ) ;
#62237=CARTESIAN_POINT ( 'NONE',  ( 12.19687500061451502, 0.000000000000000000, 4.756430356249998326 ) ) ;
#62238=ORIENTED_EDGE ( 'NONE', *, *, #46580, .T. ) ;
#62246=CARTESIAN_POINT ( 'NONE',  ( 12.44999999999999929, 0.000000000000000000, 4.999999999999998224 ) ) ;
#62257=CARTESIAN_POINT ( 'NONE',  ( 29.85937500061451644, 0.000000000000000000, 4.756430356249998326 ) ) ;
#62260=CARTESIAN_POINT ( 'NONE',  ( 8.493750001229027902, -2.886751345948019409, 5.000000000000189182 ) ) ;
#62261=CARTESIAN_POINT ( 'NONE',  ( 11.74687500061451573, 5.492252693125287522, 3.363034840372157021E-16 ) ) ;
#62270=CARTESIAN_POINT ( 'NONE',  ( 8.062500000000000000, -5.773502691896255534, -1.060575238724906372E-15 ) ) ;
#62271=( BOUNDED_CURVE ( )  B_SPLINE_CURVE ( 2, ( #28624, #62600, #11996, #51162, #69243, #6817, #29351 ),
 .UNSPECIFIED., .F., .F. ) 
 B_SPLINE_CURVE_WITH_KNOTS ( ( 3, 2, 2, 3 ),
 ( 0.7199999999999999734, 0.7233333333333333837, 0.7266666666666666829, 0.7299999999999999822 ),
 .UNSPECIFIED. ) 
 CURVE ( )  GEOMETRIC_REPRESENTATION_ITEM ( )  RATIONAL_B_SPLINE_CURVE ( ( 1.000000000000000000, 0.8660254037844387076, 1.000000000000000000, 0.8660254037844387076, 1.000000000000000000, 0.8660254037844387076, 1.000000000000000000 ) ) 
 REPRESENTATION_ITEM ( '' )  );
#62280=CARTESIAN_POINT ( 'NONE',  ( 24.20625000122903359, 0.000000000000000000, 4.999999999999998224 ) ) ;
#62310=CARTESIAN_POINT ( 'NONE',  ( 15.59999999999999964, 0.000000000000000000, 4.999999999999998224 ) ) ;
#62322=ORIENTED_EDGE ( 'NONE', *, *, #39433, .F. ) ;
#62325=CARTESIAN_POINT ( 'NONE',  ( 19.54687500061451289, -4.119189519843965641, -2.378215178125001383 ) ) ;
#62342=CARTESIAN_POINT ( 'NONE',  ( 19.47187500061451360, 2.746126346562643317, 4.756430356249998326 ) ) ;
#62351=CYLINDRICAL_SURFACE ( 'NONE', #40721, 4.999999999999998224 ) ;
#62358=CARTESIAN_POINT ( 'NONE',  ( 29.45625000122903003, 4.330127018922192761, -2.499999999999997780 ) ) ;
#62363=CARTESIAN_POINT ( 'NONE',  ( 8.034375000614518925, 5.824947211148865298E-16, -4.756430356249998326 ) ) ;
#62383=CARTESIAN_POINT ( 'NONE',  ( 10.32187500061451679, 2.746126346562645981, -4.756430356249997438 ) ) ;
#62404=CARTESIAN_POINT ( 'NONE',  ( 17.97187500061451360, 4.119189519843966529, 2.378215178124999607 ) ) ;
#62407=CARTESIAN_POINT ( 'NONE',  ( 25.17187500061451644, 4.119189519843966529, 2.378215178124999607 ) ) ;
#62414=CARTESIAN_POINT ( 'NONE',  ( 21.82499999999999574, 4.330127018922191873, 2.499999999999999556 ) ) ;
#62421=CARTESIAN_POINT ( 'NONE',  ( 27.75937500061451502, -4.119189519843965641, -2.378215178125001383 ) ) ;
#62431=ORIENTED_EDGE ( 'NONE', *, *, #63830, .F. ) ;
#62441=CARTESIAN_POINT ( 'NONE',  ( 13.58437500061451786, 4.119189519843966529, 2.378215178124999607 ) ) ;
#62472=CARTESIAN_POINT ( 'NONE',  ( 16.54687500061451644, -2.746126346562642428, -4.756430356249999214 ) ) ;
#62478=CARTESIAN_POINT ( 'NONE',  ( 16.80000000000000071, 4.330127018922192761, -2.499999999999997780 ) ) ;
#62481=DIRECTION ( 'NONE',  ( -1.000000000000000000, -0.000000000000000000, -0.000000000000000000 ) ) ;
#62482=CARTESIAN_POINT ( 'NONE',  ( 24.75937500061451502, 2.746126346562643317, 4.756430356249998326 ) ) ;
#62489=CARTESIAN_POINT ( 'NONE',  ( 23.89687500061451431, 0.000000000000000000, 4.756430356249998326 ) ) ;
#62491=CARTESIAN_POINT ( 'NONE',  ( 10.35937500061451644, 2.746126346562643317, 4.756430356249998326 ) ) ;
#62499=LINE ( 'NONE', #5271, #53758 ) ;
#62501=ORIENTED_EDGE ( 'NONE', *, *, #15601, .F. ) ;
#62503=CARTESIAN_POINT ( 'NONE',  ( 13.39687500061451431, 4.119189519843966529, -2.378215178124998275 ) ) ;
#62525=CARTESIAN_POINT ( 'NONE',  ( 22.69687500061451857, -2.746126346562646425, 4.756430356249996549 ) ) ;
#62527=CARTESIAN_POINT ( 'NONE',  ( 25.10625000122903216, 0.000000000000000000, 4.999999999999998224 ) ) ;
#62545=CARTESIAN_POINT ( 'NONE',  ( 15.46875000122903110, 2.886751345948129099, -4.999999999999998224 ) ) ;
#62548=CARTESIAN_POINT ( 'NONE',  ( 29.41875000122903216, 2.886751345948139313, -4.999999999999980460 ) ) ;
#62562=CARTESIAN_POINT ( 'NONE',  ( 24.72187500061451360, 2.746126346562645981, -4.756430356249997438 ) ) ;
#62568=CARTESIAN_POINT ( 'NONE',  ( 26.88749999999999574, -2.886751345948129988, 4.999999999999997335 ) ) ;
#62577=CARTESIAN_POINT ( 'NONE',  ( 10.03125000122903288, 6.123233995736764310E-16, -4.999999999999998224 ) ) ;
#62581=CARTESIAN_POINT ( 'NONE',  ( 18.12187500061451928, -4.119189519843968306, 2.378215178124996054 ) ) ;
#62589=CARTESIAN_POINT ( 'NONE',  ( 20.47500000000000142, 4.330127018922191873, 2.499999999999999556 ) ) ;
#62593=CARTESIAN_POINT ( 'NONE',  ( 12.34687500061451537, -4.119189519843965641, -2.378215178125001383 ) ) ;
#62594=ORIENTED_EDGE ( 'NONE', *, *, #56020, .T. ) ;
#62600=CARTESIAN_POINT ( 'NONE',  ( 13.76250000000000107, 2.886751345948126879, 4.999999999999998224 ) ) ;
#62615=CARTESIAN_POINT ( 'NONE',  ( 29.48437500061451644, -2.746126346562641984, -4.756430356249999214 ) ) ;
#62616=CARTESIAN_POINT ( 'NONE',  ( 13.43437500061451750, 5.824947211148865298E-16, -4.756430356249998326 ) ) ;
#62634=CARTESIAN_POINT ( 'NONE',  ( 22.33125000122903003, 4.330127018922191873, 2.499999999999999556 ) ) ;
#62659=CARTESIAN_POINT ( 'NONE',  ( 45.00000000000000000, 0.000000000000000000, 0.000000000000000000 ) ) ;
#62669=CARTESIAN_POINT ( 'NONE',  ( 7.837499999999999467, 5.773502691896255534, 3.535250795749688401E-16 ) ) ;
#62685=CARTESIAN_POINT ( 'NONE',  ( 18.53437500061451360, -2.746126346562646425, 4.756430356249996549 ) ) ;
#62689=LINE ( 'NONE', #11725, #43306 ) ;
#62697=EDGE_CURVE ( 'NONE', #67289, #21751, #14496, .T. ) ;
#62701=VECTOR ( 'NONE', #45099, 1000.000000000000000 ) ;
#62703=CARTESIAN_POINT ( 'NONE',  ( 18.87187500061451573, 2.746126346562645981, -4.756430356249997438 ) ) ;
#62721=EDGE_CURVE ( 'NONE', #9134, #69337, #22054, .T. ) ;
#62745=CARTESIAN_POINT ( 'NONE',  ( 17.79375000122903572, 5.773502691896255534, 3.535250795749688401E-16 ) ) ;
#62746=CARTESIAN_POINT ( 'NONE',  ( 8.259375000614518569, 0.000000000000000000, 4.756430356249998326 ) ) ;
#62757=CARTESIAN_POINT ( 'NONE',  ( 9.712500000000002132, 2.886751345948126879, 4.999999999999998224 ) ) ;
#62766=CARTESIAN_POINT ( 'NONE',  ( 16.95937500061451431, 2.746126346562645981, -4.756430356249997438 ) ) ;
#62769=CARTESIAN_POINT ( 'NONE',  ( 26.89687500061451431, 4.119189519843966529, -2.378215178124998275 ) ) ;
#62783=CARTESIAN_POINT ( 'NONE',  ( 26.03437500061451715, 5.824947211148865298E-16, -4.756430356249998326 ) ) ;
#62801=CARTESIAN_POINT ( 'NONE',  ( 15.72187500061451892, 2.746126346562645981, -4.756430356249997438 ) ) ;
#62815=CARTESIAN_POINT ( 'NONE',  ( 21.89999999999999858, 0.000000000000000000, 4.999999999999998224 ) ) ;
#62828=ORIENTED_EDGE ( 'NONE', *, *, #2690, .T. ) ;
#62831=CARTESIAN_POINT ( 'NONE',  ( 16.99687500061451573, -2.746126346562642428, -4.756430356249999214 ) ) ;
#62832=PLANE ( 'NONE',  #58560 ) ;
#62833=EDGE_CURVE ( 'NONE', #29422, #26491, #14366, .T. ) ;
#62839=CARTESIAN_POINT ( 'NONE',  ( 16.27499999999999858, 6.123233995736764310E-16, -4.999999999999998224 ) ) ;
#62842=CARTESIAN_POINT ( 'NONE',  ( 26.10937500061451644, 2.746126346562643317, 4.756430356249998326 ) ) ;
#62845=DIRECTION ( 'NONE',  ( 0.000000000000000000, -1.000000000000000000, 0.000000000000000000 ) ) ;
#62849=CARTESIAN_POINT ( 'NONE',  ( 23.78437500061451360, 5.492252693125287522, 3.363034840372157021E-16 ) ) ;
#62851=CARTESIAN_POINT ( 'NONE',  ( 10.09687500061451715, -4.119189519843965641, -2.378215178125001383 ) ) ;
#62862=CARTESIAN_POINT ( 'NONE',  ( 10.99687500061451573, -4.119189519843965641, -2.378215178125001383 ) ) ;
#62869=CARTESIAN_POINT ( 'NONE',  ( 14.92500000000000071, 6.123233995736764310E-16, -4.999999999999998224 ) ) ;
#62873=EDGE_LOOP ( 'NONE', ( #24873, #45813, #44496, #32485 ) ) ;
#62876=LINE ( 'NONE', #72523, #69119 ) ;
#62881=CARTESIAN_POINT ( 'NONE',  ( 22.80937500061451573, -4.119189519843965641, -2.378215178125001383 ) ) ;
#62894=CARTESIAN_POINT ( 'NONE',  ( 18.35625000122903216, 0.000000000000000000, 4.999999999999998224 ) ) ;
#62902=CARTESIAN_POINT ( 'NONE',  ( 16.48125000122903216, 4.330127018922191873, 2.499999999999999556 ) ) ;
#62904=CARTESIAN_POINT ( 'NONE',  ( 10.10625000122903216, 4.330127018922192761, -2.499999999999997780 ) ) ;
#62918=CARTESIAN_POINT ( 'NONE',  ( 24.15937500061451715, -4.119189519843965641, -2.378215178125001383 ) ) ;
#62924=CARTESIAN_POINT ( 'NONE',  ( 23.47499999999999787, 6.123233995736764310E-16, -4.999999999999998224 ) ) ;
#62929=CYLINDRICAL_SURFACE ( 'NONE', #706, 4.999999999999998224 ) ;
#62933=CARTESIAN_POINT ( 'NONE',  ( 9.243750001229033231, 5.773502691896255534, 3.535250795749688894E-16 ) ) ;
#62936=CARTESIAN_POINT ( 'NONE',  ( 17.63437500061451502, -2.746126346562646425, 4.756430356249996549 ) ) ;
#62943=CARTESIAN_POINT ( 'NONE',  ( 10.81875000122903252, -5.773502691896255534, -1.060575238724906372E-15 ) ) ;
#62947=CARTESIAN_POINT ( 'NONE',  ( 9.571875000614515017, -4.119189519843968306, 2.378215178124996054 ) ) ;
#62960=CARTESIAN_POINT ( 'NONE',  ( 10.20000000000000107, 0.000000000000000000, 4.999999999999998224 ) ) ;
#62972=CARTESIAN_POINT ( 'NONE',  ( 28.28437500061451715, 5.492252693125287522, 3.363034840372157021E-16 ) ) ;
#62973=CARTESIAN_POINT ( 'NONE',  ( 12.42187500061451821, -5.492252693125287522, -1.008910452111647106E-15 ) ) ;
#62990=CARTESIAN_POINT ( 'NONE',  ( 23.23125000122903216, 4.330127018922191873, 2.499999999999999556 ) ) ;
#63016=CARTESIAN_POINT ( 'NONE',  ( 25.27499999999999858, 6.123233995736764310E-16, -4.999999999999998224 ) ) ;
#63037=VERTEX_POINT ( 'NONE', #39464 ) ;
#63040=CARTESIAN_POINT ( 'NONE',  ( 19.58437500061451786, -2.746126346562642428, -4.756430356249999214 ) ) ;
#63048=CARTESIAN_POINT ( 'NONE',  ( 9.750000000000001776, 0.000000000000000000, 4.999999999999998224 ) ) ;
#63056=LINE ( 'NONE', #17621, #46931 ) ;
#63057=CARTESIAN_POINT ( 'NONE',  ( 19.54687500061451644, -2.746126346562646425, 4.756430356249996549 ) ) ;
#63070=EDGE_LOOP ( 'NONE', ( #56601, #41481, #22707, #14567 ) ) ;
#63077=EDGE_CURVE ( 'NONE', #7820, #16810, #26932, .T. ) ;
#63082=DIRECTION ( 'NONE',  ( 0.000000000000000000, 0.000000000000000000, 1.000000000000000000 ) ) ;
#63105=CARTESIAN_POINT ( 'NONE',  ( 8.521875000614516082, 2.746126346562645981, -4.756430356249997438 ) ) ;
#63109=EDGE_CURVE ( 'NONE', #65422, #38854, #49098, .T. ) ;
#63115=DIRECTION ( 'NONE',  ( 0.000000000000000000, 0.000000000000000000, 1.000000000000000000 ) ) ;
#63118=CARTESIAN_POINT ( 'NONE',  ( 9.750000000000001776, 0.000000000000000000, 4.999999999999998224 ) ) ;
#63126=CARTESIAN_POINT ( 'NONE',  ( 16.84687500061451715, -4.119189519843965641, -2.378215178125001383 ) ) ;
#63129=CARTESIAN_POINT ( 'NONE',  ( 27.04687500061451289, 0.000000000000000000, 4.756430356249998326 ) ) ;
#63144=CARTESIAN_POINT ( 'NONE',  ( 26.18437500061451573, 4.119189519843966529, 2.378215178124999607 ) ) ;
#63162=CARTESIAN_POINT ( 'NONE',  ( 15.30937500061451750, 4.119189519843966529, -2.378215178124998275 ) ) ;
#63177=VERTEX_POINT ( 'NONE', #16550 ) ;
#63189=AXIS2_PLACEMENT_3D ( 'NONE', #6133, #44942, #5412 ) ;
#63194=CARTESIAN_POINT ( 'NONE',  ( 17.14687500061451786, 5.492252693125287522, 3.363034840372157021E-16 ) ) ;
#63200=CARTESIAN_POINT ( 'NONE',  ( 16.98750000000000426, -2.886751345948129988, 4.999999999999997335 ) ) ;
#63203=CYLINDRICAL_SURFACE ( 'NONE', #2926, 4.999999999999998224 ) ;
#63204=CARTESIAN_POINT ( 'NONE',  ( 22.88437500061451502, 5.492252693125287522, 3.363034840372157021E-16 ) ) ;
#63206=EDGE_CURVE ( 'NONE', #3601, #4240, #2631, .T. ) ;
#63212=CARTESIAN_POINT ( 'NONE',  ( 24.87187500061451217, -4.119189519843968306, 2.378215178124996054 ) ) ;
#63214=CARTESIAN_POINT ( 'NONE',  ( 11.18437500061451573, 5.492252693125287522, 3.363034840372157021E-16 ) ) ;
#63223=CARTESIAN_POINT ( 'NONE',  ( 19.27500000000000213, -4.330127018922194537, 2.499999999999995559 ) ) ;
#63227=CARTESIAN_POINT ( 'NONE',  ( 11.85937500061451821, -5.492252693125287522, -1.008910452111647106E-15 ) ) ;
#63244=CARTESIAN_POINT ( 'NONE',  ( 29.84999999999999787, 4.330127018922192761, -2.499999999999997780 ) ) ;
#63246=CARTESIAN_POINT ( 'NONE',  ( 21.72187500061451715, 2.746126346562643317, 4.756430356249998326 ) ) ;
#63250=( BOUNDED_CURVE ( )  B_SPLINE_CURVE ( 2, ( #23715, #7461, #18160, #40728, #35889, #7102, #46626 ),
 .UNSPECIFIED., .F., .F. ) 
 B_SPLINE_CURVE_WITH_KNOTS ( ( 3, 2, 2, 3 ),
 ( 0.7700000000000001288, 0.7733333333333334281, 0.7766666666666667274, 0.7800000000000001377 ),
 .UNSPECIFIED. ) 
 CURVE ( )  GEOMETRIC_REPRESENTATION_ITEM ( )  RATIONAL_B_SPLINE_CURVE ( ( 0.9999999999999955591, 0.8660254037844431485, 1.000000000000000000, 0.8660254037844387076, 1.000000000000000000, 0.8660254037844342667, 1.000000000000004441 ) ) 
 REPRESENTATION_ITEM ( '' )  );
#63267=CARTESIAN_POINT ( 'NONE',  ( 17.15625000122903288, -4.330127018922190985, -2.500000000000001332 ) ) ;
#63283=CARTESIAN_POINT ( 'NONE',  ( 24.42187500061451999, 2.746126346562643317, 4.756430356249998326 ) ) ;
#63286=CARTESIAN_POINT ( 'NONE',  ( 29.32499999999999929, 6.123233995736764310E-16, -4.999999999999998224 ) ) ;
#63288=CARTESIAN_POINT ( 'NONE',  ( 24.26249999999999929, -5.773502691896255534, -1.060575238724906372E-15 ) ) ;
#63294=CARTESIAN_POINT ( 'NONE',  ( 24.88125000122903074, 6.123233995736764310E-16, -4.999999999999998224 ) ) ;
#63298=CARTESIAN_POINT ( 'NONE',  ( 10.14375000122903536, 5.773502691896255534, 3.535250795749688894E-16 ) ) ;
#63301=CARTESIAN_POINT ( 'NONE',  ( 18.00937500061451502, 2.746126346562643317, 4.756430356249998326 ) ) ;
#63312=CARTESIAN_POINT ( 'NONE',  ( 45.00000000000000000, 0.000000000000000000, 0.000000000000000000 ) ) ;
#63313=CARTESIAN_POINT ( 'NONE',  ( 11.55937500061451573, 2.746126346562645981, -4.756430356249997438 ) ) ;
#63319=( BOUNDED_CURVE ( )  B_SPLINE_CURVE ( 2, ( #64877, #37901, #20163, #14998, #20903, #65238, #70427 ),
 .UNSPECIFIED., .F., .F. ) 
 B_SPLINE_CURVE_WITH_KNOTS ( ( 3, 2, 2, 3 ),
 ( 0.6300000000000000044, 0.6333333333333333037, 0.6366666666666668251, 0.6400000000000001243 ),
 .UNSPECIFIED. ) 
 CURVE ( )  GEOMETRIC_REPRESENTATION_ITEM ( )  RATIONAL_B_SPLINE_CURVE ( ( 1.000000000000000000, 0.8660254037844387076, 1.000000000000000000, 0.8660254037844387076, 1.000000000000000000, 0.8660254037844342667, 1.000000000000004441 ) ) 
 REPRESENTATION_ITEM ( '' )  );
#63325=AXIS2_PLACEMENT_3D ( 'NONE', #64201, #57928, #35765 ) ;
#63329=CARTESIAN_POINT ( 'NONE',  ( 10.83750000000000036, -2.886751345948125991, -5.000000000000000000 ) ) ;
#63339=CARTESIAN_POINT ( 'NONE',  ( 29.63437500061451502, 5.824947211148865298E-16, -4.756430356249998326 ) ) ;
#63341=CARTESIAN_POINT ( 'NONE',  ( 27.60937500061450933, -5.492252693125287522, -1.008910452111647106E-15 ) ) ;
#63342=CARTESIAN_POINT ( 'NONE',  ( 12.75937500061451857, 0.000000000000000000, 4.756430356249998326 ) ) ;
#63349=EDGE_CURVE ( 'NONE', #26800, #34969, #22460, .T. ) ;
#63352=( BOUNDED_CURVE ( )  B_SPLINE_CURVE ( 2, ( #38513, #32965, #56232, #39610, #4540, #10073, #61401 ),
 .UNSPECIFIED., .F., .F. ) 
 B_SPLINE_CURVE_WITH_KNOTS ( ( 3, 2, 2, 3 ),
 ( 0.5499999999999999334, 0.5533333333333332327, 0.5566666666666666430, 0.5600000000000000533 ),
 .UNSPECIFIED. ) 
 CURVE ( )  GEOMETRIC_REPRESENTATION_ITEM ( )  RATIONAL_B_SPLINE_CURVE ( ( 1.000000000000004441, 0.8660254037844342667, 1.000000000000000000, 0.8660254037844387076, 1.000000000000000000, 0.8660254037844387076, 1.000000000000000000 ) ) 
 REPRESENTATION_ITEM ( '' )  );
#63355=SURFACE_SIDE_STYLE ('',( #51915 ) ) ;
#63360=CARTESIAN_POINT ( 'NONE',  ( 23.30625000122903145, 0.000000000000000000, 4.999999999999998224 ) ) ;
#63362=CARTESIAN_POINT ( 'NONE',  ( 22.68750000000000000, 5.773502691896255534, 3.535250795749688401E-16 ) ) ;
#63385=DIRECTION ( 'NONE',  ( -1.000000000000000000, -0.000000000000000000, -0.000000000000000000 ) ) ;
#63406=ORIENTED_EDGE ( 'NONE', *, *, #17177, .T. ) ;
#63409=CARTESIAN_POINT ( 'NONE',  ( 18.23437500061451644, -2.746126346562642428, -4.756430356249999214 ) ) ;
#63426=CARTESIAN_POINT ( 'NONE',  ( 11.23125000122903216, -4.330127018922194537, 2.499999999999995559 ) ) ;
#63427=CARTESIAN_POINT ( 'NONE',  ( 20.78437500061451715, 4.119189519843966529, 2.378215178124999607 ) ) ;
#63442=CARTESIAN_POINT ( 'NONE',  ( 13.87500000000000178, -4.330127018922194537, 2.499999999999995559 ) ) ;
#63452=CARTESIAN_POINT ( 'NONE',  ( 14.73749999999999893, -2.886751345948074920, 5.000000000000092371 ) ) ;
#63457=DIRECTION ( 'NONE',  ( -1.000000000000000000, -0.000000000000000000, -0.000000000000000000 ) ) ;
#63471=CARTESIAN_POINT ( 'NONE',  ( 27.95625000122903359, -4.330127018922190985, -2.500000000000001332 ) ) ;
#63472=CARTESIAN_POINT ( 'NONE',  ( 8.634375000614518569, 4.119189519843966529, 2.378215178124999607 ) ) ;
#63473=DIRECTION ( 'NONE',  ( -1.000000000000000000, -0.000000000000000000, -0.000000000000000000 ) ) ;
#63483=CARTESIAN_POINT ( 'NONE',  ( 24.39375000122903359, -2.886751345948126435, -5.000000000000000000 ) ) ;
#63491=CARTESIAN_POINT ( 'NONE',  ( 18.42187500061451644, 4.119189519843966529, 2.378215178124999607 ) ) ;
#63494=CARTESIAN_POINT ( 'NONE',  ( 25.54687500061451644, 4.119189519843966529, -2.378215178124998275 ) ) ;
#63510=CARTESIAN_POINT ( 'NONE',  ( 26.44687500061451502, -2.746126346562642428, -4.756430356249999214 ) ) ;
#63513=CARTESIAN_POINT ( 'NONE',  ( 19.42499999999999716, 6.123233995736764310E-16, -4.999999999999998224 ) ) ;
#63518=ORIENTED_EDGE ( 'NONE', *, *, #30034, .T. ) ;
#63528=CARTESIAN_POINT ( 'NONE',  ( 11.44687500061451679, -2.746126346562646425, 4.756430356249996549 ) ) ;
#63541=CARTESIAN_POINT ( 'NONE',  ( 22.05000000000000071, -4.330127018922190985, -2.500000000000001332 ) ) ;
#63554=ORIENTED_EDGE ( 'NONE', *, *, #74, .T. ) ;
#63558=CARTESIAN_POINT ( 'NONE',  ( 15.23437500061451644, 5.824947211148865298E-16, -4.756430356249998326 ) ) ;
#63564=CARTESIAN_POINT ( 'NONE',  ( 17.96250000000000213, -5.773502691896255534, -1.060575238724906372E-15 ) ) ;
#63567=DIRECTION ( 'NONE',  ( 0.000000000000000000, 0.000000000000000000, 1.000000000000000000 ) ) ;
#63568=CARTESIAN_POINT ( 'NONE',  ( 23.82187500061451502, 4.119189519843966529, 2.378215178124999607 ) ) ;
#63573=ADVANCED_FACE ( 'NONE', ( #57883 ), #62351, .T. ) ;
#63576=CARTESIAN_POINT ( 'NONE',  ( 25.32187500061451502, -4.119189519843968306, 2.378215178124996054 ) ) ;
#63578=CARTESIAN_POINT ( 'NONE',  ( 12.04687500061451821, 4.119189519843966529, -2.378215178124998275 ) ) ;
#63586=CARTESIAN_POINT ( 'NONE',  ( 19.42499999999999716, 6.123233995736764310E-16, -4.999999999999998224 ) ) ;
#63590=CARTESIAN_POINT ( 'NONE',  ( 11.03437500061451360, -2.746126346562642428, -4.756430356249999214 ) ) ;
#63607=CARTESIAN_POINT ( 'NONE',  ( 22.20937500061451431, 0.000000000000000000, 4.756430356249998326 ) ) ;
#63613=ORIENTED_EDGE ( 'NONE', *, *, #22395, .T. ) ;
#63627=CARTESIAN_POINT ( 'NONE',  ( 9.449999999999999289, -4.330127018922190985, -2.500000000000001332 ) ) ;
#63632=ADVANCED_FACE ( 'NONE', ( #11747 ), #40192, .T. ) ;
#63642=CARTESIAN_POINT ( 'NONE',  ( 23.33437500061451786, 5.824947211148865298E-16, -4.756430356249998326 ) ) ;
#63647=CARTESIAN_POINT ( 'NONE',  ( 25.46249999999999858, 2.886751345948126879, 4.999999999999999112 ) ) ;
#63654=CARTESIAN_POINT ( 'NONE',  ( 22.93125000122903145, -4.330127018922194537, 2.499999999999995559 ) ) ;
#63656=CARTESIAN_POINT ( 'NONE',  ( 9.131250001229034297, 6.123233995736764310E-16, -4.999999999999998224 ) ) ;
#63659=CARTESIAN_POINT ( 'NONE',  ( 18.45937500061451431, 2.746126346562643317, 4.756430356249998326 ) ) ;
#63671=CARTESIAN_POINT ( 'NONE',  ( 9.421875000614514661, 4.119189519843966529, 2.378215178124999607 ) ) ;
#63682=CARTESIAN_POINT ( 'NONE',  ( 27.75937500061451502, 2.746126346562645981, -4.756430356249997438 ) ) ;
#63685=CARTESIAN_POINT ( 'NONE',  ( 11.58750000000000036, -2.886751345948129988, 4.999999999999997335 ) ) ;
#63693=CARTESIAN_POINT ( 'NONE',  ( 28.39687500061451431, 5.492252693125287522, 3.363034840372157021E-16 ) ) ;
#63695=CARTESIAN_POINT ( 'NONE',  ( 27.45937500061451431, 2.746126346562643317, 4.756430356249998326 ) ) ;
#63696=CARTESIAN_POINT ( 'NONE',  ( 9.796875000614519990, -2.746126346562642428, -4.756430356249999214 ) ) ;
#63710=CARTESIAN_POINT ( 'NONE',  ( 23.56875000122902719, 2.886751345948129099, -4.999999999999998224 ) ) ;
#63734=CARTESIAN_POINT ( 'NONE',  ( 22.25625000122903074, 4.330127018922192761, -2.499999999999997780 ) ) ;
#63739=ADVANCED_FACE ( 'NONE', ( #70803 ), #58244, .T. ) ;
#63740=( BOUNDED_CURVE ( )  B_SPLINE_CURVE ( 2, ( #72658, #43857, #55303, #61202, #21303, #72290, #21668 ),
 .UNSPECIFIED., .F., .F. ) 
 B_SPLINE_CURVE_WITH_KNOTS ( ( 3, 2, 2, 3 ),
 ( 0.8500000000000001998, 0.8533333333333336101, 0.8566666666666669094, 0.8600000000000002087 ),
 .UNSPECIFIED. ) 
 CURVE ( )  GEOMETRIC_REPRESENTATION_ITEM ( )  RATIONAL_B_SPLINE_CURVE ( ( 0.9999999999999911182, 0.8660254037844475894, 1.000000000000000000, 0.8660254037844387076, 1.000000000000000000, 0.8660254037844298258, 1.000000000000008882 ) ) 
 REPRESENTATION_ITEM ( '' )  );
#63741=CARTESIAN_POINT ( 'NONE',  ( 23.77499999999999858, -4.330127018922194537, 2.499999999999995559 ) ) ;
#63745=CARTESIAN_POINT ( 'NONE',  ( 19.18125000122903501, 4.330127018922191873, 2.499999999999999556 ) ) ;
#63759=ORIENTED_EDGE ( 'NONE', *, *, #7133, .T. ) ;
#63762=CARTESIAN_POINT ( 'NONE',  ( 17.10937500061451644, 2.746126346562643317, 4.756430356249998326 ) ) ;
#63779=CARTESIAN_POINT ( 'NONE',  ( 18.11250000000000071, 2.886751345948129099, -4.999999999999997335 ) ) ;
#63782=CARTESIAN_POINT ( 'NONE',  ( 20.93437500061451573, -4.119189519843968306, 2.378215178124996054 ) ) ;
#63793=DIRECTION ( 'NONE',  ( 0.000000000000000000, 0.000000000000000000, 1.000000000000000000 ) ) ;
#63803=DIRECTION ( 'NONE',  ( -1.000000000000000000, -0.000000000000000000, -0.000000000000000000 ) ) ;
#63811=ORIENTED_EDGE ( 'NONE', *, *, #53665, .F. ) ;
#63824=CARTESIAN_POINT ( 'NONE',  ( 29.21249999999999858, -5.773502691896255534, -1.060575238724906372E-15 ) ) ;
#63830=EDGE_CURVE ( 'NONE', #39550, #72150, #69713, .T. ) ;
#63844=CARTESIAN_POINT ( 'NONE',  ( 15.98437500061451644, -2.746126346562642428, -4.756430356249999214 ) ) ;
#63847=CARTESIAN_POINT ( 'NONE',  ( 27.12187500061451573, -4.119189519843968306, 2.378215178124996054 ) ) ;
#63851=CARTESIAN_POINT ( 'NONE',  ( 28.80000000000000071, -4.330127018922190985, -2.500000000000001332 ) ) ;
#63854=CARTESIAN_POINT ( 'NONE',  ( 28.14375000122903359, 5.773502691896255534, 3.535250795749688401E-16 ) ) ;
#63855=DIRECTION ( 'NONE',  ( 0.000000000000000000, 0.000000000000000000, 1.000000000000000000 ) ) ;
#63862=CARTESIAN_POINT ( 'NONE',  ( 26.89687500061451431, -2.746126346562642428, -4.756430356249999214 ) ) ;
#63865=CARTESIAN_POINT ( 'NONE',  ( 25.23750000000000071, -2.886751345948153968, -4.999999999999952038 ) ) ;
#63866=DIRECTION ( 'NONE',  ( -1.000000000000000000, -0.000000000000000000, -0.000000000000000000 ) ) ;
#63880=CARTESIAN_POINT ( 'NONE',  ( 12.15937500061451892, 4.119189519843966529, -2.378215178124998275 ) ) ;
#63894=CARTESIAN_POINT ( 'NONE',  ( 23.49375000122903501, -2.886751345948153968, -4.999999999999952038 ) ) ;
#63895=ORIENTED_EDGE ( 'NONE', *, *, #60122, .F. ) ;
#63913=UNCERTAINTY_MEASURE_WITH_UNIT (LENGTH_MEASURE( 1.000000000000000082E-05 ), #46737, 'distance_accuracy_value', 'NONE');
#63915=CARTESIAN_POINT ( 'NONE',  ( 15.45937500061451608, 0.000000000000000000, 4.756430356249998326 ) ) ;
#63916=ADVANCED_FACE ( 'NONE', ( #14643 ), #48644, .T. ) ;
#63917=CARTESIAN_POINT ( 'NONE',  ( 13.40625000122903288, 0.000000000000000000, 4.999999999999998224 ) ) ;
#63922=CARTESIAN_POINT ( 'NONE',  ( 18.07499999999999929, 6.123233995736764310E-16, -4.999999999999998224 ) ) ;
#63926=CARTESIAN_POINT ( 'NONE',  ( 22.47187500061451360, 4.119189519843966529, 2.378215178124999607 ) ) ;
#63934=CARTESIAN_POINT ( 'NONE',  ( 23.67187500061451289, 5.824947211148865298E-16, -4.756430356249998326 ) ) ;
#63936=CARTESIAN_POINT ( 'NONE',  ( 8.934375000614517504, 5.492252693125287522, 3.363034840372157021E-16 ) ) ;
#63941=CARTESIAN_POINT ( 'NONE',  ( 9.806250001229033231, 0.000000000000000000, 4.999999999999998224 ) ) ;
#63945=CARTESIAN_POINT ( 'NONE',  ( 17.81250000000000355, 2.886751345948182834, 4.999999999999902300 ) ) ;
#63948=CARTESIAN_POINT ( 'NONE',  ( 12.79687500061451466, -4.119189519843965641, -2.378215178125001383 ) ) ;
#63953=( BOUNDED_CURVE ( )  B_SPLINE_CURVE ( 2, ( #9540, #4011, #31342, #53883, #26535, #49074, #3275 ),
 .UNSPECIFIED., .F., .F. ) 
 B_SPLINE_CURVE_WITH_KNOTS ( ( 3, 2, 2, 3 ),
 ( 0.5999999999999999778, 0.6033333333333334991, 0.6066666666666667984, 0.6100000000000002087 ),
 .UNSPECIFIED. ) 
 CURVE ( )  GEOMETRIC_REPRESENTATION_ITEM ( )  RATIONAL_B_SPLINE_CURVE ( ( 1.000000000000000000, 0.8660254037844387076, 1.000000000000000000, 0.8660254037844387076, 1.000000000000000000, 0.8660254037844298258, 1.000000000000008882 ) ) 
 REPRESENTATION_ITEM ( '' )  );
#63956=CARTESIAN_POINT ( 'NONE',  ( 23.51249999999999929, 2.886751345948101122, -5.000000000000046185 ) ) ;
#63968=CARTESIAN_POINT ( 'NONE',  ( 18.90937500061451360, 4.119189519843966529, -2.378215178124998275 ) ) ;
#63970=CARTESIAN_POINT ( 'NONE',  ( 28.48125000122902861, 6.123233995736764310E-16, -4.999999999999998224 ) ) ;
#63975=ORIENTED_EDGE ( 'NONE', *, *, #48303, .T. ) ;
#63978=ADVANCED_FACE ( 'NONE', ( #3583 ), #31653, .T. ) ;
#63989=ADVANCED_FACE ( 'NONE', ( #35722 ), #7648, .T. ) ;
#64001=VERTEX_POINT ( 'NONE', #49379 ) ;
#64004=CARTESIAN_POINT ( 'NONE',  ( 22.99687500061451573, 5.492252693125287522, 3.363034840372157021E-16 ) ) ;
#64010=CARTESIAN_POINT ( 'NONE',  ( 23.73749999999999716, -2.886751345948129988, 4.999999999999997335 ) ) ;
#64020=CARTESIAN_POINT ( 'NONE',  ( 10.44375000122903074, -2.886751345948125991, -5.000000000000000000 ) ) ;
#64022=CARTESIAN_POINT ( 'NONE',  ( 16.09687500061451715, 4.119189519843966529, -2.378215178124998275 ) ) ;
#64030=CARTESIAN_POINT ( 'NONE',  ( 45.00000000000000000, -2.499999999999999556, 3.499999999999999556 ) ) ;
#64034=CARTESIAN_POINT ( 'NONE',  ( 9.759375000614516793, 2.746126346562645981, -4.756430356249997438 ) ) ;
#64045=CARTESIAN_POINT ( 'NONE',  ( 27.72187500061451715, 5.824947211148865298E-16, -4.756430356249998326 ) ) ;
#64048=CARTESIAN_POINT ( 'NONE',  ( 8.474999999999999645, -4.330127018922194537, 2.499999999999995559 ) ) ;
#64051=ORIENTED_EDGE ( 'NONE', *, *, #50505, .F. ) ;
#64056=CARTESIAN_POINT ( 'NONE',  ( 27.60937500061451644, 0.000000000000000000, 4.756430356249998326 ) ) ;
#64058=CARTESIAN_POINT ( 'NONE',  ( 26.85937500061450933, 2.746126346562645981, -4.756430356249997438 ) ) ;
#64059=CARTESIAN_POINT ( 'NONE',  ( 9.984375000614518214, 4.119189519843966529, 2.378215178124999607 ) ) ;
#64066=CARTESIAN_POINT ( 'NONE',  ( 45.00000000000000000, 0.000000000000000000, 0.000000000000000000 ) ) ;
#64073=CARTESIAN_POINT ( 'NONE',  ( 20.86875000122903145, 2.886751345948129099, -4.999999999999998224 ) ) ;
#64075=CARTESIAN_POINT ( 'NONE',  ( 22.64999999999999858, 4.330127018922192761, -2.499999999999997780 ) ) ;
#64081=CARTESIAN_POINT ( 'NONE',  ( 10.87500000000000000, 6.123233995736764310E-16, -4.999999999999998224 ) ) ;
#64115=EDGE_CURVE ( 'NONE', #6077, #38121, #16864, .T. ) ;
#64126=CARTESIAN_POINT ( 'NONE',  ( 17.40937500061451360, 2.746126346562645981, -4.756430356249997438 ) ) ;
#64142=FACE_OUTER_BOUND ( 'NONE', #52148, .T. ) ;
#64145=CARTESIAN_POINT ( 'NONE',  ( 16.95937500061451786, -4.119189519843965641, -2.378215178125001383 ) ) ;
#64162=CARTESIAN_POINT ( 'NONE',  ( 27.58125000122903359, 6.123233995736764310E-16, -4.999999999999998224 ) ) ;
#64166=CARTESIAN_POINT ( 'NONE',  ( 7.687499999999997335, -2.886751345948237457, -4.999999999999807265 ) ) ;
#64177=EDGE_LOOP ( 'NONE', ( #49721, #4373, #32798, #48400 ) ) ;
#64191=CARTESIAN_POINT ( 'NONE',  ( 30.00000000000000000, 0.000000000000000000, 4.999999999999998224 ) ) ;
#64193=CARTESIAN_POINT ( 'NONE',  ( 20.23125000122902861, -4.330127018922194537, 2.499999999999995559 ) ) ;
#64197=CARTESIAN_POINT ( 'NONE',  ( 12.00000000000000000, 0.000000000000000000, 4.999999999999998224 ) ) ;
#64201=CARTESIAN_POINT ( 'NONE',  ( 45.00000000000000000, 0.000000000000000000, 0.000000000000000000 ) ) ;
#64209=CARTESIAN_POINT ( 'NONE',  ( 14.22187500061451537, 5.824947211148865298E-16, -4.756430356249998326 ) ) ;
#64212=CARTESIAN_POINT ( 'NONE',  ( 24.79687500061451644, 0.000000000000000000, 4.756430356249998326 ) ) ;
#64228=CARTESIAN_POINT ( 'NONE',  ( 25.17187500061451644, 2.746126346562645981, -4.756430356249997438 ) ) ;
#64232=CARTESIAN_POINT ( 'NONE',  ( 18.82500000000000284, -4.330127018922194537, 2.499999999999995559 ) ) ;
#64236=VECTOR ( 'NONE', #68413, 1000.000000000000000 ) ;
#64240=ORIENTED_EDGE ( 'NONE', *, *, #61190, .F. ) ;
#64250=CARTESIAN_POINT ( 'NONE',  ( 12.57187500061452035, 2.746126346562645981, -4.756430356249997438 ) ) ;
#64274=EDGE_CURVE ( 'NONE', #19923, #54432, #64556, .T. ) ;
#64281=CARTESIAN_POINT ( 'NONE',  ( 14.55937500061451573, 0.000000000000000000, 4.756430356249998326 ) ) ;
#64288=CARTESIAN_POINT ( 'NONE',  ( 16.23750000000000071, -2.886751345948125991, -5.000000000000000000 ) ) ;
#64291=VECTOR ( 'NONE', #42718, 1000.000000000000000 ) ;
#64293=CARTESIAN_POINT ( 'NONE',  ( 23.14687500061451786, -4.119189519843965641, -2.378215178125001383 ) ) ;
#64301=CARTESIAN_POINT ( 'NONE',  ( 22.54687500061451644, 0.000000000000000000, 4.756430356249998326 ) ) ;
#64303=CARTESIAN_POINT ( 'NONE',  ( 8.671875000614518214, -4.119189519843968306, 2.378215178124996054 ) ) ;
#64307=CARTESIAN_POINT ( 'NONE',  ( 9.993750001229033231, -2.886751345948126435, -5.000000000000000000 ) ) ;
#64314=CARTESIAN_POINT ( 'NONE',  ( 11.74687500061451573, 0.000000000000000000, 4.756430356249998326 ) ) ;
#64332=CYLINDRICAL_SURFACE ( 'NONE', #39250, 4.999999999999998224 ) ;
#64336=CARTESIAN_POINT ( 'NONE',  ( 19.62187500061451573, -5.492252693125287522, -1.008910452111647106E-15 ) ) ;
#64358=CARTESIAN_POINT ( 'NONE',  ( 21.05625000122903145, 0.000000000000000000, 4.999999999999998224 ) ) ;
#64364=FACE_OUTER_BOUND ( 'NONE', #49618, .T. ) ;
#64371=CARTESIAN_POINT ( 'NONE',  ( 21.04687500061451644, -2.746126346562642428, -4.756430356249999214 ) ) ;
#64376=CARTESIAN_POINT ( 'NONE',  ( 25.19999999999999929, -4.330127018922190985, -2.500000000000001332 ) ) ;
#64377=AXIS2_PLACEMENT_3D ( 'NONE', #13774, #31509, #54049 ) ;
#64379=DIRECTION ( 'NONE',  ( -1.000000000000000000, -0.000000000000000000, -0.000000000000000000 ) ) ;
#64380=CARTESIAN_POINT ( 'NONE',  ( 23.08125000122903359, 6.123233995736764310E-16, -4.999999999999998224 ) ) ;
#64381=CYLINDRICAL_SURFACE ( 'NONE', #6858, 4.999999999999998224 ) ;
#64388=CARTESIAN_POINT ( 'NONE',  ( 29.10937500061451999, 2.746126346562645981, -4.756430356249997438 ) ) ;
#64390=CARTESIAN_POINT ( 'NONE',  ( 16.13437500061451502, 5.492252693125287522, 3.363034840372157021E-16 ) ) ;
#64402=CARTESIAN_POINT ( 'NONE',  ( 11.37187500061451573, -4.119189519843968306, 2.378215178124996054 ) ) ;
#64408=ORIENTED_EDGE ( 'NONE', *, *, #49257, .F. ) ;
#64413=CARTESIAN_POINT ( 'NONE',  ( 29.59687500061451360, 4.119189519843966529, -2.378215178124998275 ) ) ;
#64416=CARTESIAN_POINT ( 'NONE',  ( 9.412499999999999645, -5.773502691896255534, -1.060575238724906372E-15 ) ) ;
#64419=ORIENTED_EDGE ( 'NONE', *, *, #65890, .T. ) ;
#64424=CARTESIAN_POINT ( 'NONE',  ( 26.89687500061451431, -2.746126346562641984, -4.756430356249999214 ) ) ;
#64426=CARTESIAN_POINT ( 'NONE',  ( 10.69687500061451679, -2.746126346562642428, -4.756430356249999214 ) ) ;
#64434=DIRECTION ( 'NONE',  ( 0.000000000000000000, 0.000000000000000000, 1.000000000000000000 ) ) ;
#64442=CARTESIAN_POINT ( 'NONE',  ( 21.20625000122903359, -4.330127018922190985, -2.500000000000001332 ) ) ;
#64448=ADVANCED_FACE ( 'NONE', ( #17551 ), #17905, .T. ) ;
#64458=CARTESIAN_POINT ( 'NONE',  ( 29.63437500061451502, 5.824947211148865298E-16, -4.756430356249998326 ) ) ;
#64466=CARTESIAN_POINT ( 'NONE',  ( 25.38749999999999929, 5.773502691896255534, 3.535250795749688401E-16 ) ) ;
#64475=VECTOR ( 'NONE', #52100, 1000.000000000000000 ) ;
#64487=VERTEX_POINT ( 'NONE', #29732 ) ;
#64495=CARTESIAN_POINT ( 'NONE',  ( 15.90937500061451360, -5.492252693125287522, -1.008910452111647106E-15 ) ) ;
#64515=CARTESIAN_POINT ( 'NONE',  ( 17.25937500061451502, 0.000000000000000000, 4.756430356249998326 ) ) ;
#64532=CARTESIAN_POINT ( 'NONE',  ( 27.24375000122903145, 5.773502691896255534, 3.535250795749688894E-16 ) ) ;
#64545=VERTEX_POINT ( 'NONE', #11308 ) ;
#64546=ORIENTED_EDGE ( 'NONE', *, *, #16678, .F. ) ;
#64548=CYLINDRICAL_SURFACE ( 'NONE', #29107, 4.999999999999998224 ) ;
#64556=( BOUNDED_CURVE ( )  B_SPLINE_CURVE ( 2, ( #65625, #32013, #49743, #54548, #21282, #38277, #61537 ),
 .UNSPECIFIED., .F., .F. ) 
 B_SPLINE_CURVE_WITH_KNOTS ( ( 3, 2, 2, 3 ),
 ( 0.7500000000000000000, 0.7533333333333332993, 0.7566666666666667096, 0.7600000000000000089 ),
 .UNSPECIFIED. ) 
 CURVE ( )  GEOMETRIC_REPRESENTATION_ITEM ( )  RATIONAL_B_SPLINE_CURVE ( ( 1.000000000000000000, 0.8660254037844387076, 1.000000000000000000, 0.8660254037844387076, 1.000000000000000000, 0.8660254037844387076, 1.000000000000000000 ) ) 
 REPRESENTATION_ITEM ( '' )  );
#64561=CARTESIAN_POINT ( 'NONE',  ( 7.846875000614518036, -2.746126346562646425, 4.756430356249996549 ) ) ;
#64577=EDGE_CURVE ( 'NONE', #50518, #43273, #51398, .T. ) ;
#64580=CARTESIAN_POINT ( 'NONE',  ( 15.83437500061451253, -2.746126346562646425, 4.756430356249996549 ) ) ;
#64583=CARTESIAN_POINT ( 'NONE',  ( 23.07187500061451502, -4.119189519843968306, 2.378215178124996054 ) ) ;
#64590=CARTESIAN_POINT ( 'NONE',  ( 23.25000000000000000, 0.000000000000000000, 4.999999999999998224 ) ) ;
#64599=CARTESIAN_POINT ( 'NONE',  ( 24.72187500061451360, 2.746126346562645981, -4.756430356249997438 ) ) ;
#64602=CARTESIAN_POINT ( 'NONE',  ( 25.08749999999999858, -2.886751345948130876, 4.999999999999996447 ) ) ;
#64603=DIRECTION ( 'NONE',  ( -1.000000000000000000, -0.000000000000000000, -0.000000000000000000 ) ) ;
#64611=ORIENTED_EDGE ( 'NONE', *, *, #30682, .F. ) ;
#64620=CARTESIAN_POINT ( 'NONE',  ( 12.75937500061451857, 0.000000000000000000, 4.756430356249998326 ) ) ;
#64627=( BOUNDED_CURVE ( )  B_SPLINE_CURVE ( 2, ( #52130, #29950, #19580, #52490, #64662, #14047, #24405 ),
 .UNSPECIFIED., .F., .T. ) 
 B_SPLINE_CURVE_WITH_KNOTS ( ( 3, 2, 2, 3 ),
 ( 0.1599999999999999756, 0.1633333333333333026, 0.1666666666666666019, 0.1699999999999999567 ),
 .UNSPECIFIED. ) 
 CURVE ( )  GEOMETRIC_REPRESENTATION_ITEM ( )  RATIONAL_B_SPLINE_CURVE ( ( 1.000000000000001332, 0.8660254037844377084, 1.000000000000000000, 0.8660254037844387076, 1.000000000000000000, 0.8660254037844409281, 0.9999999999999977796 ) ) 
 REPRESENTATION_ITEM ( '' )  );
#64637=CARTESIAN_POINT ( 'NONE',  ( 16.08749999999999858, -2.886751345948130876, 4.999999999999996447 ) ) ;
#64647=EDGE_LOOP ( 'NONE', ( #63811, #27187, #18354, #34163 ) ) ;
#64650=CARTESIAN_POINT ( 'NONE',  ( 13.39687500061451608, -2.746126346562642428, -4.756430356249999214 ) ) ;
#64657=CARTESIAN_POINT ( 'NONE',  ( 15.22500000000000142, -4.330127018922194537, 2.499999999999995559 ) ) ;
#64661=CARTESIAN_POINT ( 'NONE',  ( 24.19687500061451502, 4.119189519843966529, -2.378215178124998275 ) ) ;
#64662=CARTESIAN_POINT ( 'NONE',  ( 26.25000000000000000, 4.330127018922192761, -2.499999999999997780 ) ) ;
#64670=CARTESIAN_POINT ( 'NONE',  ( 21.34687500061451715, -4.119189519843965641, -2.378215178125001383 ) ) ;
#64672=CARTESIAN_POINT ( 'NONE',  ( 8.409375000614515372, 2.746126346562645981, -4.756430356249997438 ) ) ;
#64683=CARTESIAN_POINT ( 'NONE',  ( 8.296875000614518214, -4.119189519843965641, -2.378215178125001383 ) ) ;
#64702=CARTESIAN_POINT ( 'NONE',  ( 14.08125000122903181, 6.123233995736764310E-16, -4.999999999999998224 ) ) ;
#64705=CARTESIAN_POINT ( 'NONE',  ( 19.24687500061452283, -2.746126346562641984, -4.756430356249999214 ) ) ;
#64710=EDGE_LOOP ( 'NONE', ( #49080, #39660, #30292, #65743 ) ) ;
#64730=CYLINDRICAL_SURFACE ( 'NONE', #55696, 4.999999999999998224 ) ;
#64733=ORIENTED_EDGE ( 'NONE', *, *, #15774, .T. ) ;
#64737=CARTESIAN_POINT ( 'NONE',  ( 21.87187500061451573, -5.492252693125287522, -1.008910452111647106E-15 ) ) ;
#64743=CARTESIAN_POINT ( 'NONE',  ( 22.23750000000000071, 5.773502691896255534, 3.535250795749688894E-16 ) ) ;
#64749=CARTESIAN_POINT ( 'NONE',  ( 18.61875000122903145, 2.886751345948073588, -5.000000000000094147 ) ) ;
#64754=CARTESIAN_POINT ( 'NONE',  ( 29.29687500061451644, 0.000000000000000000, 4.756430356249998326 ) ) ;
#64756=CARTESIAN_POINT ( 'NONE',  ( 14.89687500061451608, 0.000000000000000000, 4.756430356249998326 ) ) ;
#64766=CARTESIAN_POINT ( 'NONE',  ( 45.00000000000000000, 0.000000000000000000, 4.999999999999998224 ) ) ;
#64767=CARTESIAN_POINT ( 'NONE',  ( 7.959375000614516082, 2.746126346562645981, -4.756430356249997438 ) ) ;
#64772=ORIENTED_EDGE ( 'NONE', *, *, #62833, .F. ) ;
#64777=CARTESIAN_POINT ( 'NONE',  ( 28.54687500061451644, -4.119189519843965641, -2.378215178125001383 ) ) ;
#64781=CARTESIAN_POINT ( 'NONE',  ( 7.500000000000000000, 0.000000000000000000, 4.999999999999998224 ) ) ;
#64788=CARTESIAN_POINT ( 'NONE',  ( 27.87187500061451573, 2.746126346562645981, -4.756430356249997438 ) ) ;
#64790=CARTESIAN_POINT ( 'NONE',  ( 10.73437500061451644, 5.824947211148865298E-16, -4.756430356249998326 ) ) ;
#64808=CARTESIAN_POINT ( 'NONE',  ( 20.45625000122903359, 4.330127018922192761, -2.499999999999997780 ) ) ;
#64823=EDGE_CURVE ( 'NONE', #28145, #17484, #47450, .T. ) ;
#64825=CARTESIAN_POINT ( 'NONE',  ( 29.07187500061451502, -5.492252693125287522, -1.008910452111647106E-15 ) ) ;
#64831=( BOUNDED_CURVE ( )  B_SPLINE_CURVE ( 2, ( #35153, #63945, #45885, #46606, #28887, #34785, #12975 ),
 .UNSPECIFIED., .F., .F. ) 
 B_SPLINE_CURVE_WITH_KNOTS ( ( 3, 2, 2, 3 ),
 ( 0.5400000000000001465, 0.5433333333333333348, 0.5466666666666666341, 0.5499999999999999334 ),
 .UNSPECIFIED. ) 
 CURVE ( )  GEOMETRIC_REPRESENTATION_ITEM ( )  RATIONAL_B_SPLINE_CURVE ( ( 0.9999999999999955591, 0.8660254037844431485, 1.000000000000000000, 0.8660254037844387076, 1.000000000000000000, 0.8660254037844431485, 0.9999999999999955591 ) ) 
 REPRESENTATION_ITEM ( '' )  );
#64835=CARTESIAN_POINT ( 'NONE',  ( 7.556250001229035007, 0.000000000000000000, 4.999999999999998224 ) ) ;
#64851=CARTESIAN_POINT ( 'NONE',  ( 45.00000000000000000, 0.000000000000000000, 4.999999999999998224 ) ) ;
#64862=CARTESIAN_POINT ( 'NONE',  ( 17.22187500061451360, -4.119189519843968306, 2.378215178124996054 ) ) ;
#64877=CARTESIAN_POINT ( 'NONE',  ( 15.43125000122903323, 6.123233995736764310E-16, -4.999999999999998224 ) ) ;
#64878=DIRECTION ( 'NONE',  ( 1.000000000000000000, 0.000000000000000000, 0.000000000000000000 ) ) ;
#64879=DIRECTION ( 'NONE',  ( -1.000000000000000000, -0.000000000000000000, -0.000000000000000000 ) ) ;
#64882=CARTESIAN_POINT ( 'NONE',  ( 16.47187500061452070, -5.492252693125287522, -1.008910452111647106E-15 ) ) ;
#64896=CARTESIAN_POINT ( 'NONE',  ( 13.79999999999999893, 0.000000000000000000, 4.999999999999998224 ) ) ;
#64900=CARTESIAN_POINT ( 'NONE',  ( 28.33125000122903359, -4.330127018922194537, 2.499999999999995559 ) ) ;
#64903=CARTESIAN_POINT ( 'NONE',  ( 26.23125000122903216, 6.123233995736764310E-16, -4.999999999999998224 ) ) ;
#64925=CARTESIAN_POINT ( 'NONE',  ( 28.83749999999999858, -2.886751345948125991, -5.000000000000000000 ) ) ;
#64931=CARTESIAN_POINT ( 'NONE',  ( 11.96250000000000213, 2.886751345948126879, 4.999999999999998224 ) ) ;
#64940=ADVANCED_FACE ( 'NONE', ( #24181 ), #70347, .T. ) ;
#64944=CARTESIAN_POINT ( 'NONE',  ( 16.43437500061451573, -2.746126346562642428, -4.756430356249999214 ) ) ;
#64947=CARTESIAN_POINT ( 'NONE',  ( 23.70937500061451075, 2.746126346562645981, -4.756430356249997438 ) ) ;
#64952=CARTESIAN_POINT ( 'NONE',  ( 15.41250000000000142, 2.886751345948129099, -4.999999999999997335 ) ) ;
#64956=CARTESIAN_POINT ( 'NONE',  ( 23.71875000122902577, 2.886751345948154857, 4.999999999999951150 ) ) ;
#64958=CARTESIAN_POINT ( 'NONE',  ( 13.04999999999999893, -4.330127018922190985, -2.500000000000001332 ) ) ;
#64965=CARTESIAN_POINT ( 'NONE',  ( 25.39687500061451431, -2.746126346562646425, 4.756430356249996549 ) ) ;
#64968=CARTESIAN_POINT ( 'NONE',  ( 13.36875000122903323, 2.886751345948126879, 4.999999999999998224 ) ) ;
#64969=DIRECTION ( 'NONE',  ( -1.000000000000000000, -0.000000000000000000, -0.000000000000000000 ) ) ;
#64985=CARTESIAN_POINT ( 'NONE',  ( 11.89687500061451608, -2.746126346562646425, 4.756430356249996549 ) ) ;
#64999=ORIENTED_EDGE ( 'NONE', *, *, #30907, .T. ) ;
#65015=CARTESIAN_POINT ( 'NONE',  ( 13.95937500061451786, 4.119189519843966529, -2.378215178124998275 ) ) ;
#65017=CARTESIAN_POINT ( 'NONE',  ( 13.59375000122903288, -2.886751345948237457, -4.999999999999807265 ) ) ;
#65022=CARTESIAN_POINT ( 'NONE',  ( 14.66249999999999964, 2.886751345948126879, 4.999999999999999112 ) ) ;
#65024=FACE_OUTER_BOUND ( 'NONE', #58207, .T. ) ;
#65028=CARTESIAN_POINT ( 'NONE',  ( 45.00000000000000000, 0.000000000000000000, 0.000000000000000000 ) ) ;
#65033=CARTESIAN_POINT ( 'NONE',  ( 22.69687500061451502, -4.119189519843965641, -2.378215178125001383 ) ) ;
#65035=CARTESIAN_POINT ( 'NONE',  ( 9.721875000614517148, 5.824947211148865298E-16, -4.756430356249998326 ) ) ;
#65047=CARTESIAN_POINT ( 'NONE',  ( 9.196875000614515017, -4.119189519843965641, -2.378215178125001383 ) ) ;
#65057=ORIENTED_EDGE ( 'NONE', *, *, #5869, .T. ) ;
#65069=CARTESIAN_POINT ( 'NONE',  ( 20.55937500061451573, -4.119189519843965641, -2.378215178125001383 ) ) ;
#65091=EDGE_CURVE ( 'NONE', #48096, #24010, #14189, .T. ) ;
#65103=CARTESIAN_POINT ( 'NONE',  ( 20.33437500061451786, 4.119189519843966529, 2.378215178124999607 ) ) ;
#65109=CARTESIAN_POINT ( 'NONE',  ( 21.63749999999999929, -2.886751345948125991, -5.000000000000000000 ) ) ;
#65115=CARTESIAN_POINT ( 'NONE',  ( 18.65625000122902932, 4.330127018922192761, -2.499999999999997780 ) ) ;
#65120=CARTESIAN_POINT ( 'NONE',  ( 29.07187500061451502, 5.824947211148865298E-16, -4.756430356249998326 ) ) ;
#65122=CARTESIAN_POINT ( 'NONE',  ( 16.47187500061451715, 5.824947211148865298E-16, -4.756430356249998326 ) ) ;
#65125=ORIENTED_EDGE ( 'NONE', *, *, #43245, .F. ) ;
#65128=CARTESIAN_POINT ( 'NONE',  ( 17.11875000122903145, -5.773502691896255534, -1.060575238724906372E-15 ) ) ;
#65142=CARTESIAN_POINT ( 'NONE',  ( 27.90937500061451715, 2.746126346562643317, 4.756430356249998326 ) ) ;
#65153=CARTESIAN_POINT ( 'NONE',  ( 27.72187500061451715, -5.492252693125287522, -1.008910452111647106E-15 ) ) ;
#65155=CARTESIAN_POINT ( 'NONE',  ( 10.17187500061451999, -5.492252693125287522, -1.008910452111647106E-15 ) ) ;
#65173=CARTESIAN_POINT ( 'NONE',  ( 19.93125000122903145, 6.123233995736764310E-16, -4.999999999999998224 ) ) ;
#65175=CARTESIAN_POINT ( 'NONE',  ( 21.35625000122903216, 4.330127018922192761, -2.499999999999997780 ) ) ;
#65176=VERTEX_POINT ( 'NONE', #15647 ) ;
#65189=CARTESIAN_POINT ( 'NONE',  ( 27.98437500061451289, 4.119189519843966529, 2.378215178124999607 ) ) ;
#65209=ORIENTED_EDGE ( 'NONE', *, *, #42828, .F. ) ;
#65210=CARTESIAN_POINT ( 'NONE',  ( 10.59375000122903288, 5.773502691896255534, 3.535250795749688401E-16 ) ) ;
#65224=CARTESIAN_POINT ( 'NONE',  ( 16.17187500061451644, 4.119189519843966529, 2.378215178124999607 ) ) ;
#65238=CARTESIAN_POINT ( 'NONE',  ( 15.24375000122903323, -2.886751345948074920, 5.000000000000092371 ) ) ;
#65239=CARTESIAN_POINT ( 'NONE',  ( 18.13125000122903074, 6.123233995736764310E-16, -4.999999999999998224 ) ) ;
#65243=CARTESIAN_POINT ( 'NONE',  ( 17.37187500061451573, -5.492252693125287522, -1.008910452111647106E-15 ) ) ;
#65260=EDGE_CURVE ( 'NONE', #48156, #66756, #38934, .T. ) ;
#65261=CARTESIAN_POINT ( 'NONE',  ( 28.40625000122903288, -4.330127018922190985, -2.500000000000001332 ) ) ;
#65263=CARTESIAN_POINT ( 'NONE',  ( 45.00000000000000000, 0.000000000000000000, 0.000000000000000000 ) ) ;
#65273=ORIENTED_EDGE ( 'NONE', *, *, #37851, .T. ) ;
#65286=CARTESIAN_POINT ( 'NONE',  ( 7.396875000614519635, -2.746126346562646425, 4.756430356249996549 ) ) ;
#65303=ADVANCED_FACE ( 'NONE', ( #54460 ), #33016, .T. ) ;
#65304=CARTESIAN_POINT ( 'NONE',  ( 15.27187500061451608, 4.119189519843966529, 2.378215178124999607 ) ) ;
#65308=CARTESIAN_POINT ( 'NONE',  ( 23.63437500061451502, -2.746126346562642428, -4.756430356249999214 ) ) ;
#65313=LINE ( 'NONE', #42064, #30792 ) ;
#65318=CARTESIAN_POINT ( 'NONE',  ( 45.00000000000000000, -2.499999999999999556, -3.499999999999999556 ) ) ;
#65319=CARTESIAN_POINT ( 'NONE',  ( 13.98750000000000249, -2.886751345948125991, -5.000000000000000000 ) ) ;
#65326=CARTESIAN_POINT ( 'NONE',  ( 24.75937500061451502, 4.119189519843966529, -2.378215178124998275 ) ) ;
#65330=CARTESIAN_POINT ( 'NONE',  ( 13.18125000122903323, 6.123233995736764310E-16, -4.999999999999998224 ) ) ;
#65338=ORIENTED_EDGE ( 'NONE', *, *, #32494, .T. ) ;
#65348=CARTESIAN_POINT ( 'NONE',  ( 8.896875000614517859, -2.746126346562641984, -4.756430356249999214 ) ) ;
#65361=VERTEX_POINT ( 'NONE', #21193 ) ;
#65373=ORIENTED_EDGE ( 'NONE', *, *, #41825, .F. ) ;
#65376=CARTESIAN_POINT ( 'NONE',  ( 12.90937500061451537, -4.119189519843965641, -2.378215178125001383 ) ) ;
#65379=CARTESIAN_POINT ( 'NONE',  ( 13.44375000122903074, -2.886751345948130876, 4.999999999999996447 ) ) ;
#65384=CARTESIAN_POINT ( 'NONE',  ( 14.24999999999999822, 0.000000000000000000, 4.999999999999998224 ) ) ;
#65387=AXIS2_PLACEMENT_3D ( 'NONE', #4990, #6072, #10888 ) ;
#65398=CARTESIAN_POINT ( 'NONE',  ( 22.20937500061451786, -5.492252693125287522, -1.008910452111647106E-15 ) ) ;
#65400=CARTESIAN_POINT ( 'NONE',  ( 8.896875000614517859, 4.119189519843966529, -2.378215178124998275 ) ) ;
#65411=CARTESIAN_POINT ( 'NONE',  ( 10.05937500061451750, -5.492252693125287522, -1.008910452111647106E-15 ) ) ;
#65414=( BOUNDED_CURVE ( )  B_SPLINE_CURVE ( 2, ( #32832, #10662, #27659, #56098, #55731, #39107, #71996 ),
 .UNSPECIFIED., .F., .F. ) 
 B_SPLINE_CURVE_WITH_KNOTS ( ( 3, 2, 2, 3 ),
 ( 0.09999999999999995004, 0.1033333333333332771, 0.1066666666666666041, 0.1099999999999999312 ),
 .UNSPECIFIED. ) 
 CURVE ( )  GEOMETRIC_REPRESENTATION_ITEM ( )  RATIONAL_B_SPLINE_CURVE ( ( 1.000000000000002220, 0.8660254037844364872, 1.000000000000000000, 0.8660254037844387076, 1.000000000000000000, 0.8660254037844414832, 0.9999999999999972244 ) ) 
 REPRESENTATION_ITEM ( '' )  );
#65422=VERTEX_POINT ( 'NONE', #65905 ) ;
#65431=CARTESIAN_POINT ( 'NONE',  ( 22.91250000000000142, -5.773502691896255534, -1.060575238724906372E-15 ) ) ;
#65434=CARTESIAN_POINT ( 'NONE',  ( 20.07187500061451857, -5.492252693125287522, -1.008910452111647106E-15 ) ) ;
#65453=CARTESIAN_POINT ( 'NONE',  ( 20.49375000122903145, 5.773502691896255534, 3.535250795749688401E-16 ) ) ;
#65468=CARTESIAN_POINT ( 'NONE',  ( 21.23437500061451644, 4.119189519843966529, 2.378215178124999607 ) ) ;
#65473=( BOUNDED_CURVE ( )  B_SPLINE_CURVE ( 2, ( #823, #69145, #6718, #18135, #5636, #17063, #39623 ),
 .UNSPECIFIED., .F., .F. ) 
 B_SPLINE_CURVE_WITH_KNOTS ( ( 3, 2, 2, 3 ),
 ( 0.5899999999999999689, 0.5933333333333333792, 0.5966666666666666785, 0.5999999999999999778 ),
 .UNSPECIFIED. ) 
 CURVE ( )  GEOMETRIC_REPRESENTATION_ITEM ( )  RATIONAL_B_SPLINE_CURVE ( ( 1.000000000000000000, 0.8660254037844387076, 1.000000000000000000, 0.8660254037844387076, 1.000000000000000000, 0.8660254037844387076, 1.000000000000000000 ) ) 
 REPRESENTATION_ITEM ( '' )  );
#65476=CARTESIAN_POINT ( 'NONE',  ( 21.41250000000000497, 2.886751345948126879, 4.999999999999999112 ) ) ;
#65487=CARTESIAN_POINT ( 'NONE',  ( 29.03437500061451360, -2.746126346562642428, -4.756430356249999214 ) ) ;
#65489=CARTESIAN_POINT ( 'NONE',  ( 16.58437500061451431, 5.492252693125287522, 3.363034840372157021E-16 ) ) ;
#65492=ORIENTED_EDGE ( 'NONE', *, *, #52283, .T. ) ;
#65495=CARTESIAN_POINT ( 'NONE',  ( 26.13750000000000284, -2.886751345948098013, -5.000000000000047073 ) ) ;
#65502=EDGE_CURVE ( 'NONE', #72010, #21883, #49042, .T. ) ;
#65507=ORIENTED_EDGE ( 'NONE', *, *, #73043, .T. ) ;
#65508=LINE ( 'NONE', #69601, #56075 ) ;
#65517=CARTESIAN_POINT ( 'NONE',  ( 8.587500000000002132, -2.886751345948125991, -5.000000000000000000 ) ) ;
#65525=CARTESIAN_POINT ( 'NONE',  ( 27.83437500061451786, 5.824947211148865298E-16, -4.756430356249998326 ) ) ;
#65527=CARTESIAN_POINT ( 'NONE',  ( 7.846875000614518036, -2.746126346562646425, 4.756430356249996549 ) ) ;
#65544=CARTESIAN_POINT ( 'NONE',  ( 21.99375000122903145, -2.886751345948129988, 4.999999999999997335 ) ) ;
#65557=( GEOMETRIC_REPRESENTATION_CONTEXT ( 3 ) GLOBAL_UNCERTAINTY_ASSIGNED_CONTEXT ( ( #54310 ) ) GLOBAL_UNIT_ASSIGNED_CONTEXT ( ( #71243, #60146, #28365 ) ) REPRESENTATION_CONTEXT ( 'NONE', 'WORKASPACE' ) );
#65559=CARTESIAN_POINT ( 'NONE',  ( 28.92187500061451644, 2.746126346562643317, 4.756430356249998326 ) ) ;
#65574=CARTESIAN_POINT ( 'NONE',  ( 23.21250000000000213, 2.886751345948126879, 4.999999999999998224 ) ) ;
#65579=EDGE_LOOP ( 'NONE', ( #51787, #12571, #35643, #70858 ) ) ;
#65590=EDGE_CURVE ( 'NONE', #11954, #61742, #67398, .T. ) ;
#65595=CARTESIAN_POINT ( 'NONE',  ( 14.52187500061451608, -4.119189519843968306, 2.378215178124996054 ) ) ;
#65611=CARTESIAN_POINT ( 'NONE',  ( 45.00000000000000000, 0.000000000000000000, 0.000000000000000000 ) ) ;
#65614=CARTESIAN_POINT ( 'NONE',  ( 16.77187500061451786, 2.746126346562643317, 4.756430356249998326 ) ) ;
#65625=CARTESIAN_POINT ( 'NONE',  ( 13.12500000000000178, 6.123233995736764310E-16, -4.999999999999998224 ) ) ;
#65632=CARTESIAN_POINT ( 'NONE',  ( 27.91875000122903216, -5.773502691896255534, -1.060575238724906372E-15 ) ) ;
#65656=CARTESIAN_POINT ( 'NONE',  ( 27.78749999999999787, -2.886751345948129988, 4.999999999999997335 ) ) ;
#65680=CARTESIAN_POINT ( 'NONE',  ( 24.87187500061451217, -4.119189519843968306, 2.378215178124996054 ) ) ;
#65690=CARTESIAN_POINT ( 'NONE',  ( 14.13750000000000107, 5.773502691896255534, 3.535250795749688894E-16 ) ) ;
#65697=CARTESIAN_POINT ( 'NONE',  ( 24.27187500061452141, 2.746126346562645981, -4.756430356249997438 ) ) ;
#65705=( BOUNDED_CURVE ( )  B_SPLINE_CURVE ( 2, ( #28012, #1387, #16898, #44648, #1027, #34617, #662 ),
 .UNSPECIFIED., .F., .F. ) 
 B_SPLINE_CURVE_WITH_KNOTS ( ( 3, 2, 2, 3 ),
 ( 0.3400000000000000799, 0.3433333333333333792, 0.3466666666666667895, 0.3500000000000000888 ),
 .UNSPECIFIED. ) 
 CURVE ( )  GEOMETRIC_REPRESENTATION_ITEM ( )  RATIONAL_B_SPLINE_CURVE ( ( 0.9999999999999977796, 0.8660254037844409281, 1.000000000000000000, 0.8660254037844387076, 1.000000000000000000, 0.8660254037844342667, 1.000000000000004441 ) ) 
 REPRESENTATION_ITEM ( '' )  );
#65719=CARTESIAN_POINT ( 'NONE',  ( 8.821875000614518569, -5.492252693125287522, -1.008910452111647106E-15 ) ) ;
#65743=ORIENTED_EDGE ( 'NONE', *, *, #2690, .F. ) ;
#65744=EDGE_CURVE ( 'NONE', #11954, #6463, #28925, .T. ) ;
#65747=CARTESIAN_POINT ( 'NONE',  ( 14.37187500061451928, 2.746126346562645981, -4.756430356249997438 ) ) ;
#65755=CARTESIAN_POINT ( 'NONE',  ( 15.18750000000000000, -2.886751345948129988, 4.999999999999997335 ) ) ;
#65768=CARTESIAN_POINT ( 'NONE',  ( 19.92187500061451289, -4.119189519843968306, 2.378215178124996054 ) ) ;
#65783=CARTESIAN_POINT ( 'NONE',  ( 10.09687500061451715, -4.119189519843965641, -2.378215178125001383 ) ) ;
#65790=CARTESIAN_POINT ( 'NONE',  ( 14.69999999999999929, 0.000000000000000000, 4.999999999999998224 ) ) ;
#65806=CARTESIAN_POINT ( 'NONE',  ( 16.02187500061451786, -5.492252693125287522, -1.008910452111647106E-15 ) ) ;
#65810=VERTEX_POINT ( 'NONE', #62894 ) ;
#65825=CARTESIAN_POINT ( 'NONE',  ( 20.41875000122903572, 2.886751345948157077, -4.999999999999949374 ) ) ;
#65838=CARTESIAN_POINT ( 'NONE',  ( 21.38437500061451502, -4.119189519843968306, 2.378215178124996054 ) ) ;
#65845=CARTESIAN_POINT ( 'NONE',  ( 22.08749999999999858, -2.886751345948125991, -5.000000000000000000 ) ) ;
#65849=CARTESIAN_POINT ( 'NONE',  ( 20.54999999999999716, 0.000000000000000000, 4.999999999999998224 ) ) ;
#65857=CARTESIAN_POINT ( 'NONE',  ( 29.55937500061451217, 2.746126346562645981, -4.756430356249997438 ) ) ;
#65859=CARTESIAN_POINT ( 'NONE',  ( 13.92187500061451644, 4.119189519843966529, 2.378215178124999607 ) ) ;
#65871=CARTESIAN_POINT ( 'NONE',  ( 8.221875000614515372, -4.119189519843968306, 2.378215178124996054 ) ) ;
#65877=CARTESIAN_POINT ( 'NONE',  ( 45.00000000000000000, 0.000000000000000000, 0.000000000000000000 ) ) ;
#65890=EDGE_CURVE ( 'NONE', #17152, #4778, #69305, .T. ) ;
#65894=CARTESIAN_POINT ( 'NONE',  ( 23.48437500061451644, 4.119189519843966529, 2.378215178124999607 ) ) ;
#65896=CARTESIAN_POINT ( 'NONE',  ( 7.996875000614519280, -2.746126346562642428, -4.756430356249999214 ) ) ;
#65905=CARTESIAN_POINT ( 'NONE',  ( 23.53125000122902932, 6.123233995736764310E-16, -4.999999999999998224 ) ) ;
#65906=CARTESIAN_POINT ( 'NONE',  ( 8.175000000000002487, 6.123233995736764310E-16, -4.999999999999998224 ) ) ;
#65913=CARTESIAN_POINT ( 'NONE',  ( 17.98125000122903572, -4.330127018922194537, 2.499999999999995559 ) ) ;
#65929=CARTESIAN_POINT ( 'NONE',  ( 27.83437500061451786, 5.824947211148865298E-16, -4.756430356249998326 ) ) ;
#65965=CARTESIAN_POINT ( 'NONE',  ( 14.89687500061451608, 0.000000000000000000, 4.756430356249998326 ) ) ;
#65979=CARTESIAN_POINT ( 'NONE',  ( 9.506250001229030744, -4.330127018922190985, -2.500000000000001332 ) ) ;
#65983=CARTESIAN_POINT ( 'NONE',  ( 27.09375000122903288, -2.886751345948091796, -5.000000000000060396 ) ) ;
#65984=CARTESIAN_POINT ( 'NONE',  ( 14.55937500061451573, 0.000000000000000000, 4.756430356249998326 ) ) ;
#65997=CARTESIAN_POINT ( 'NONE',  ( 24.61875000122903145, 2.886751345948126879, 4.999999999999998224 ) ) ;
#66001=CARTESIAN_POINT ( 'NONE',  ( 25.70625000122903003, -4.330127018922190985, -2.500000000000001332 ) ) ;
#66012=ORIENTED_EDGE ( 'NONE', *, *, #42665, .T. ) ;
#66048=CARTESIAN_POINT ( 'NONE',  ( 20.22187500061451715, 4.119189519843966529, 2.378215178124999607 ) ) ;
#66057=CARTESIAN_POINT ( 'NONE',  ( 12.67499999999999893, 6.123233995736764310E-16, -4.999999999999998224 ) ) ;
#66064=CARTESIAN_POINT ( 'NONE',  ( 22.92187500061451644, 2.746126346562645981, -4.756430356249997438 ) ) ;
#66067=( BOUNDED_CURVE ( )  B_SPLINE_CURVE ( 2, ( #25002, #8382, #2477, #8020, #63442, #12828, #64896 ),
 .UNSPECIFIED., .F., .F. ) 
 B_SPLINE_CURVE_WITH_KNOTS ( ( 3, 2, 2, 3 ),
 ( 0.7100000000000001865, 0.7133333333333334858, 0.7166666666666667851, 0.7199999999999999734 ),
 .UNSPECIFIED. ) 
 CURVE ( )  GEOMETRIC_REPRESENTATION_ITEM ( )  RATIONAL_B_SPLINE_CURVE ( ( 0.9999999999999911182, 0.8660254037844475894, 1.000000000000000000, 0.8660254037844387076, 1.000000000000000000, 0.8660254037844387076, 1.000000000000000000 ) ) 
 REPRESENTATION_ITEM ( '' )  );
#66086=CARTESIAN_POINT ( 'NONE',  ( 10.09687500061451715, -2.746126346562646425, 4.756430356249996549 ) ) ;
#66112=CARTESIAN_POINT ( 'NONE',  ( 12.72187500061451537, 2.746126346562643317, 4.756430356249998326 ) ) ;
#66132=CARTESIAN_POINT ( 'NONE',  ( 18.94687500061451857, 0.000000000000000000, 4.756430356249998326 ) ) ;
#66135=CARTESIAN_POINT ( 'NONE',  ( 14.60625000122903216, 4.330127018922192761, -2.499999999999997780 ) ) ;
#66149=CARTESIAN_POINT ( 'NONE',  ( 9.046875000614514661, 0.000000000000000000, 4.756430356249998326 ) ) ;
#66172=CARTESIAN_POINT ( 'NONE',  ( 18.12187500061451928, 2.746126346562643317, 4.756430356249998326 ) ) ;
#66185=ORIENTED_EDGE ( 'NONE', *, *, #19403, .T. ) ;
#66204=CARTESIAN_POINT ( 'NONE',  ( 19.17187500061451999, -5.492252693125287522, -1.008910452111647106E-15 ) ) ;
#66210=CARTESIAN_POINT ( 'NONE',  ( 21.82499999999999574, 4.330127018922191873, 2.499999999999999556 ) ) ;
#66213=CARTESIAN_POINT ( 'NONE',  ( 14.53125000122903288, 6.123233995736764310E-16, -4.999999999999998224 ) ) ;
#66215=CARTESIAN_POINT ( 'NONE',  ( 28.19999999999999929, 0.000000000000000000, 4.999999999999998224 ) ) ;
#66220=CARTESIAN_POINT ( 'NONE',  ( 27.15937500061451360, -5.492252693125287522, -1.008910452111647106E-15 ) ) ;
#66222=CARTESIAN_POINT ( 'NONE',  ( 14.22187500061451537, 5.824947211148865298E-16, -4.756430356249998326 ) ) ;
#66256=CARTESIAN_POINT ( 'NONE',  ( 23.78437500061451360, 5.824947211148865298E-16, -4.756430356249998326 ) ) ;
#66258=CARTESIAN_POINT ( 'NONE',  ( 9.046875000614518214, 5.492252693125287522, 3.363034840372157021E-16 ) ) ;
#66277=CARTESIAN_POINT ( 'NONE',  ( 17.86875000122903145, 2.886751345948126879, 4.999999999999999112 ) ) ;
#66280=ORIENTED_EDGE ( 'NONE', *, *, #22854, .F. ) ;
#66286=FACE_OUTER_BOUND ( 'NONE', #1155, .T. ) ;
#66293=CARTESIAN_POINT ( 'NONE',  ( 28.50937500061451502, 0.000000000000000000, 4.756430356249998326 ) ) ;
#66304=CARTESIAN_POINT ( 'NONE',  ( 7.331250001229031810, 6.123233995736764310E-16, -4.999999999999998224 ) ) ;
#66310=CARTESIAN_POINT ( 'NONE',  ( 10.96875000122903465, 2.886751345948129099, -4.999999999999998224 ) ) ;
#66314=CARTESIAN_POINT ( 'NONE',  ( 20.25937500061451502, 2.746126346562643317, 4.756430356249998326 ) ) ;
#66325=ORIENTED_EDGE ( 'NONE', *, *, #14684, .F. ) ;
#66329=CARTESIAN_POINT ( 'NONE',  ( 21.20625000122903359, -4.330127018922190985, -2.500000000000001332 ) ) ;
#66332=CARTESIAN_POINT ( 'NONE',  ( 14.48437500061451644, -2.746126346562646425, 4.756430356249996549 ) ) ;
#66349=CARTESIAN_POINT ( 'NONE',  ( 26.90625000122902932, 0.000000000000000000, 4.999999999999998224 ) ) ;
#66350=CARTESIAN_POINT ( 'NONE',  ( 15.04687500061451644, -2.746126346562646425, 4.756430356249996549 ) ) ;
#66370=CARTESIAN_POINT ( 'NONE',  ( 24.65625000122903288, 0.000000000000000000, 4.999999999999998224 ) ) ;
#66382=CARTESIAN_POINT ( 'NONE',  ( 13.78125000122903288, 4.330127018922191873, 2.499999999999999556 ) ) ;
#66415=ORIENTED_EDGE ( 'NONE', *, *, #3065, .F. ) ;
#66418=CARTESIAN_POINT ( 'NONE',  ( 21.30937500061451217, -5.492252693125287522, -1.008910452111647106E-15 ) ) ;
#66427=CARTESIAN_POINT ( 'NONE',  ( 13.57500000000000107, 6.123233995736764310E-16, -4.999999999999998224 ) ) ;
#66434=CARTESIAN_POINT ( 'NONE',  ( 22.13437500061451502, 4.119189519843966529, 2.378215178124999607 ) ) ;
#66440=EDGE_CURVE ( 'NONE', #31771, #9134, #922, .T. ) ;
#66457=CARTESIAN_POINT ( 'NONE',  ( 10.20937500061451786, -4.119189519843965641, -2.378215178125001383 ) ) ;
#66476=ORIENTED_EDGE ( 'NONE', *, *, #44600, .T. ) ;
#66479=CARTESIAN_POINT ( 'NONE',  ( 11.18437500061451928, 5.824947211148865298E-16, -4.756430356249998326 ) ) ;
#66488=CARTESIAN_POINT ( 'NONE',  ( 45.00000000000000000, 0.000000000000000000, 0.000000000000000000 ) ) ;
#66492=LINE ( 'NONE', #21780, #9985 ) ;
#66497=EDGE_CURVE ( 'NONE', #69242, #28919, #66953, .T. ) ;
#66498=CARTESIAN_POINT ( 'NONE',  ( 20.67187500061451289, 4.119189519843966529, 2.378215178124999607 ) ) ;
#66501=CARTESIAN_POINT ( 'NONE',  ( 13.70625000122903359, 4.330127018922192761, -2.499999999999997780 ) ) ;
#66516=CARTESIAN_POINT ( 'NONE',  ( 28.50937500061451502, 0.000000000000000000, 4.756430356249998326 ) ) ;
#66537=CARTESIAN_POINT ( 'NONE',  ( 18.23437500061451999, -4.119189519843968306, 2.378215178124996054 ) ) ;
#66541=EDGE_CURVE ( 'NONE', #65176, #61955, #72116, .T. ) ;
#66557=LINE ( 'NONE', #15937, #47886 ) ;
#66570=VECTOR ( 'NONE', #23551, 1000.000000000000000 ) ;
#66572=CARTESIAN_POINT ( 'NONE',  ( 19.50937500061451857, 0.000000000000000000, 4.756430356249998326 ) ) ;
#66577=( BOUNDED_CURVE ( )  B_SPLINE_CURVE ( 2, ( #49597, #4895, #43690, #10432, #5254, #9700, #10792 ),
 .UNSPECIFIED., .F., .F. ) 
 B_SPLINE_CURVE_WITH_KNOTS ( ( 3, 2, 2, 3 ),
 ( 0.2399999999999999634, 0.2433333333333333182, 0.2466666666666666452, 0.2499999999999999722 ),
 .UNSPECIFIED. ) 
 CURVE ( )  GEOMETRIC_REPRESENTATION_ITEM ( )  RATIONAL_B_SPLINE_CURVE ( ( 1.000000000000001110, 0.8660254037844374864, 1.000000000000000000, 0.8660254037844387076, 1.000000000000000000, 0.8660254037844398178, 0.9999999999999988898 ) ) 
 REPRESENTATION_ITEM ( '' )  );
#66580=CARTESIAN_POINT ( 'NONE',  ( 20.32499999999999929, 6.123233995736764310E-16, -4.999999999999998224 ) ) ;
#66591=CARTESIAN_POINT ( 'NONE',  ( 27.04687500061451289, 0.000000000000000000, 4.756430356249998326 ) ) ;
#66594=CARTESIAN_POINT ( 'NONE',  ( 14.14687500061451431, -4.119189519843965641, -2.378215178125001383 ) ) ;
#66597=ORIENTED_EDGE ( 'NONE', *, *, #29725, .T. ) ;
#66600=EDGE_CURVE ( 'NONE', #25555, #17152, #71683, .T. ) ;
#66628=CARTESIAN_POINT ( 'NONE',  ( 25.24687500061451573, 5.492252693125287522, 3.363034840372157021E-16 ) ) ;
#66649=CARTESIAN_POINT ( 'NONE',  ( 17.68125000122903501, 6.123233995736764310E-16, -4.999999999999998224 ) ) ;
#66665=CARTESIAN_POINT ( 'NONE',  ( 25.77187500061451075, 2.746126346562643317, 4.756430356249998326 ) ) ;
#66672=AXIS2_PLACEMENT_3D ( 'NONE', #30187, #27574, #60072 ) ;
#66680=CARTESIAN_POINT ( 'NONE',  ( 8.699999999999999289, 4.330127018922192761, -2.499999999999997780 ) ) ;
#66682=CARTESIAN_POINT ( 'NONE',  ( 12.05625000122903145, 0.000000000000000000, 4.999999999999998224 ) ) ;
#66686=CARTESIAN_POINT ( 'NONE',  ( 20.89687500061451786, -4.119189519843965641, -2.378215178125001383 ) ) ;
#66699=CARTESIAN_POINT ( 'NONE',  ( 13.58437500061451431, -2.746126346562646425, 4.756430356249996549 ) ) ;
#66708=CARTESIAN_POINT ( 'NONE',  ( 14.59687500061451537, -4.119189519843965641, -2.378215178125001383 ) ) ;
#66725=CARTESIAN_POINT ( 'NONE',  ( 28.92187500061451644, -4.119189519843968306, 2.378215178124996054 ) ) ;
#66726=CARTESIAN_POINT ( 'NONE',  ( 15.15937500061451715, -4.119189519843965641, -2.378215178125001383 ) ) ;
#66745=CARTESIAN_POINT ( 'NONE',  ( 25.18125000122903145, -4.330127018922194537, 2.499999999999995559 ) ) ;
#66756=VERTEX_POINT ( 'NONE', #14206 ) ;
#66758=CARTESIAN_POINT ( 'NONE',  ( 13.81875000122903074, 2.886751345948238789, 4.999999999999807265 ) ) ;
#66770=FACE_OUTER_BOUND ( 'NONE', #51440, .T. ) ;
#66780=DIRECTION ( 'NONE',  ( -1.000000000000000000, -0.000000000000000000, -0.000000000000000000 ) ) ;
#66794=CARTESIAN_POINT ( 'NONE',  ( 21.68437500061451573, -2.746126346562646425, 4.756430356249996549 ) ) ;
#66802=EDGE_LOOP ( 'NONE', ( #30164, #43942, #5505, #22839 ) ) ;
#66803=CARTESIAN_POINT ( 'NONE',  ( 9.712500000000002132, 2.886751345948126879, 4.999999999999999112 ) ) ;
#66810=CARTESIAN_POINT ( 'NONE',  ( 21.75937500061451502, 0.000000000000000000, 4.756430356249998326 ) ) ;
#66820=VERTEX_POINT ( 'NONE', #64081 ) ;
#66832=CARTESIAN_POINT ( 'NONE',  ( 9.496875000614517504, 5.492252693125287522, 3.363034840372157021E-16 ) ) ;
#66842=ORIENTED_EDGE ( 'NONE', *, *, #51591, .F. ) ;
#66854=CARTESIAN_POINT ( 'NONE',  ( 17.28750000000000142, 5.773502691896255534, 3.535250795749688401E-16 ) ) ;
#66855=CARTESIAN_POINT ( 'NONE',  ( 10.47187500061451715, 2.746126346562643317, 4.756430356249998326 ) ) ;
#66859=EDGE_CURVE ( 'NONE', #34596, #10453, #21616, .T. ) ;
#66874=CARTESIAN_POINT ( 'NONE',  ( 45.00000000000000000, 0.000000000000000000, 0.000000000000000000 ) ) ;
#66876=CARTESIAN_POINT ( 'NONE',  ( 20.97187500061451715, 5.824947211148865298E-16, -4.756430356249998326 ) ) ;
#66879=CARTESIAN_POINT ( 'NONE',  ( 14.75625000122903252, 0.000000000000000000, 4.999999999999998224 ) ) ;
#66895=CARTESIAN_POINT ( 'NONE',  ( 29.59687500061451715, -2.746126346562642428, -4.756430356249999214 ) ) ;
#66916=CARTESIAN_POINT ( 'NONE',  ( 17.40937500061451715, -4.119189519843965641, -2.378215178125001383 ) ) ;
#66920=EDGE_LOOP ( 'NONE', ( #62431, #51485, #32649, #48387 ) ) ;
#66949=CARTESIAN_POINT ( 'NONE',  ( 18.30937500061451928, -4.119189519843965641, -2.378215178125001383 ) ) ;
#66953=( BOUNDED_CURVE ( )  B_SPLINE_CURVE ( 2, ( #69284, #68205, #29748, #52286, #12037, #46750, #40128 ),
 .UNSPECIFIED., .F., .F. ) 
 B_SPLINE_CURVE_WITH_KNOTS ( ( 3, 2, 2, 3 ),
 ( 0.04000000000000007022, 0.04333333333333339726, 0.04666666666666672431, 0.05000000000000005135 ),
 .UNSPECIFIED. ) 
 CURVE ( )  GEOMETRIC_REPRESENTATION_ITEM ( )  RATIONAL_B_SPLINE_CURVE ( ( 0.9999999999999972244, 0.8660254037844414832, 1.000000000000000000, 0.8660254037844387076, 1.000000000000000000, 0.8660254037844367092, 1.000000000000001998 ) ) 
 REPRESENTATION_ITEM ( '' )  );
#66954=EDGE_CURVE ( 'NONE', #38121, #54432, #54838, .T. ) ;
#66957=CARTESIAN_POINT ( 'NONE',  ( 19.68750000000000355, -2.886751345948129988, 4.999999999999997335 ) ) ;
#66960=CARTESIAN_POINT ( 'NONE',  ( 26.18437500061451573, -2.746126346562646425, 4.756430356249996549 ) ) ;
#66961=CARTESIAN_POINT ( 'NONE',  ( 18.88125000122903430, -4.330127018922194537, 2.499999999999995559 ) ) ;
#66967=CARTESIAN_POINT ( 'NONE',  ( 26.37187500061451573, 5.824947211148865298E-16, -4.756430356249998326 ) ) ;
#66969=CARTESIAN_POINT ( 'NONE',  ( 13.77187500061451431, 5.824947211148865298E-16, -4.756430356249998326 ) ) ;
#66977=AXIS2_PLACEMENT_3D ( 'NONE', #56081, #22449, #44998 ) ;
#66995=ORIENTED_EDGE ( 'NONE', *, *, #24066, .F. ) ;
#67005=CARTESIAN_POINT ( 'NONE',  ( 23.89687500061451786, 5.492252693125287522, 3.363034840372157021E-16 ) ) ;
#67007=CARTESIAN_POINT ( 'NONE',  ( 9.159375000614515372, 0.000000000000000000, 4.756430356249998326 ) ) ;
#67016=( BOUNDED_SURFACE ( )  B_SPLINE_SURFACE ( 1, 2, ( 
 ( #35658, #52652, #30118, #2058, #47115, #41932, #64458, #6507, #26038, #42299, #49311, #47844, #54483, #21216, #43769, #3147, #20852, #71845, #48577, #48210, #43030, #64825, #20477, #4254, #60368, #65559, #14948, #60007, #37486, #9417, #54845, #25297, #15673, #31947, #59639, #42664, #66293, #53378, #58904, #14214, #71104, #26779, #36750, #3884, #37847, #26404, #48947, #15309, #71476, #9777, #65189, #43404, #8315, #59270, #65929, #30844, #2774, #31210, #14579, #32311, #70372, #8678, #19750, #53750, #25673, #9051, #70732, #20110, #37112, #31582, #54121, #3517, #50409, #72207, #60738, #38590, #32680, #50763, #5697, #10148, #67756, #67404, #39689, #45223, #28233, #168, #6054, #10513, #11603, #50040, #22672, #44138, #17128, #33040, #21952, #27876, #67043, #62207, #61475, #11241, #61116, #27507, #34120, #61836, #44509, #55580, #56660, #4614, #28589, #66665, #33764, #55219, #27144, #21584, #4973, #49678, #72566, #16403, #10870, #56308, #51126, #523, #16042, #39323, #38957, #23034, #45589, #33403, #55940, #68123, #5336, #38210, #72933, #22315, #44868, #16765, #34483, #62562, #52928, #51489, #889, #6418, #11958, #23753, #18566, #63283, #41484, #7497, #1607, #68476, #40050, #57013, #62918, #12313, #23396, #46302, #34848, #7140, #30025, #28950, #29670, #13384, #45945, #52206, #69563, #24118, #58089, #47028, #52568, #18924, #1248, #35570, #35929, #17838, #63642, #58451, #40399, #57375, #68841, #1975, #6782, #29314, #24484, #64004, #46667, #40769, #7863, #51845, #30399, #18198, #12675, #13031, #69208, #35212, #57734, #41132, #2325, #24841, #47388, #17488, #26317, #25951, #71387, #3795, #59922, #9328, #37760, #42213, #43318, #8591, #54396, #2687, #31861, #64737, #53661, #59551, #25584, #48856, #20021, #42942, #70286, #59182, #20760, #20393, #3053, #19658, #65838, #36304, #15221, #25203, #65468, #19288, #58818, #30757, #14125, #64371, #36663, #31121, #42575, #14859, #60278, #9691, #8229, #71015, #53288, #32224, #54758, #47751, #48123, #4162, #70646, #26692, #41842, #69918, #65103, #14492, #13762, #37026, #8962, #31496, #54036, #3431, #48491, #37398, #50323, #21861, #80, #39233, #33316, #27057, #71759, #43681, #21495, #44048, #55130, #4884, #66572, #38870, #61745, #21128, #5964, #27786, #49950, #32953, #56568, #66204, #11509, #32592, #39593, #16317, #38499, #55854, #4528, #10783, #67669, #50676, #5244, #72847, #22228, #44784, #67317, #45134, #15582, #38124, #16675, #49587, #15951, #72475, #66949, #10060, #72111, #61025, #11147, #55490, #61387, #33677, #44422, #56219, #10422, #28148, #62117, #34031, #5612, #22585, #27419, #17036, #49225, #60645, #1889, #68389, #1159, #22939, #35481, #430, #34390, #797, #18479, #58003, #34753, #63194, #58362, #35838, #23305, #62831, #46214, #12225, #51395, #45854, #17750, #40309, #17401, #29939, #57288, #28498, #51034, #62472, #6694, #13301, #7411, #51759, #68753, #52479, #45499, #57646, #29223, #24394, #23668, #29582, #68030, #39958, #6326, #46943, #18111, #69479, #40674, #12589, #35123, #7053, #52120, #1522, #11869, #18837, #24027, #41400, #63915, #56922, #28855, #46576, #69121, #41044, #63558, #12945, #59831, #58729, #24755, #53200, #37669, #42492, #54311, #36575, #53944, #53567, #70191, #30309, #48767, #20669, #30667, #48037, #64281, #71290, #69835, #3341, #43227, #65747, #25116, #42854, #13669, #19198, #52841, #14034, #8868, #2962, #31774, #70929, #65015, #8141, #2240, #47298, #2596, #47658, #36212, #59095, #19569, #70563, #20300, #41753, #7776, #59460, #8501, #64650, #15131, #42124, #31031, #25492, #19938, #3702, #14403, #36940, #9238, #31404, #48403, #37309, #65376, #26229, #25864, #14765, #56126, #66112, #33222, #5519, #54666, #32501, #43958, #44692, #26596, #15491, #5154, #72752, #49860, #10329, #28057, #32133, #61653, #71664, #32863, #55760, #72384, #21039, #9601, #60556, #4070, #22137, #27689, #49136, #16584, #16227, #11052, #67223, #50227, #39135, #50585, #55035, #33580, #72024, #73113, #38034, #22495, #4438, #66479, #21764, #15857, #45045, #55398, #67580, #9963, #49495, #16946, #10691, #38403, #26966, #60191, #43590, #21401, #60926, #4794, #27326, #44326, #66855, #38779, #61297, #39871, #62383, #12139, #57561, #40957, #52391, #5874, #40585, #50943, #23940, #57917, #342, #17663, #46489, #707, #24309, #62023, #46855, #17311, #28407, #56482, #11422, #1798, #22848, #34664, #28765, #33939, #7324, #69396, #11782, #6608, #45402, #29855, #67938, #35033, #39499, #34298, #56830, #1434, #6237, #29136, #51304, #23582, #23215, #1074, #45768, #63472, #46127, #68665, #63105, #18029, #12505, #35392, #68304, #40224, #6964, #62746, #57193, #51669, #29495, #52031, #69028, #18389, #12860, #2508, #30940, #59006, #64561, #3247, #53111, #70836, #9148, #31684, #70475, #8410, #41668, #42038, #36124, #25775, #65286, #58643 ),
 ( #64191, #8051, #13578, #7684, #20212, #25031, #48677, #18750, #52753, #30585, #3615, #42766, #13950, #53481, #48313, #13217, #47947, #47574, #14674, #70104, #19852, #63824, #58276, #69745, #37218, #19480, #59740, #36487, #2873, #25404, #42403, #64925, #14315, #35755, #54217, #36851, #26136, #41314, #30220, #24667, #19113, #2156, #59367, #8778, #47213, #31313, #53856, #15045, #44515, #28955, #33771, #45597, #27881, #45228, #38964, #39328, #61481, #55946, #21959, #65656, #40055, #16771, #28595, #6061, #68128, #3983, #49048, #23039, #56313, #50770, #57018, #51131, #72572, #37583, #67050, #71201, #5703, #17494, #50415, #67761, #44874, #10875, #20577, #62568, #11964, #16409, #61842, #54579, #34489, #60105, #17134, #6423, #43132, #33408, #34126, #9514, #11246, #5342, #28238, #26508, #173, #32047, #528, #22678, #39694, #62213, #11608, #56665, #72939, #22321, #67409, #1981, #34853, #68846, #52212, #69214, #12318, #29321, #57380, #30033, #35218, #63647, #18572, #24124, #35934, #12681, #30405, #41849, #64376, #52573, #41138, #1254, #1614, #18205, #58457, #24848, #40774, #46674, #45951, #7869, #23402, #6787, #23758, #41490, #52933, #57739, #13038, #8234, #58824, #46309, #7145, #35575, #29676, #63288, #58096, #7502, #24490, #40406, #2330, #47034, #51494, #895, #51850, #69569, #36309, #47394, #18930, #64010, #69925, #68481, #13390, #19294, #13768, #17844, #62924, #2695, #70293, #8598, #32230, #42583, #4169, #37033, #20767, #60285, #14499, #48862, #26698, #36669, #3802, #49232, #25210, #3059, #59557, #15227, #19665, #59188, #71394, #43324, #20399, #54042, #71765, #47757, #54765, #42219, #3438, #26325, #42948, #64743, #53295, #31127, #14133, #65845, #37766, #53668, #9697, #59928, #21135, #43687, #66210, #15588, #38130, #25590, #60652, #65109, #30763, #48129, #70653, #20027, #8970, #65476, #31502, #25957, #48497, #71022, #14865, #37405, #9335, #54402, #31867, #10429, #62123, #49594, #11515, #15957, #5618, #32598, #72119, #44054, #4891, #4535, #32960, #55496, #55860, #28154, #34037, #22946, #21501, #11154, #66580, #67674, #28503, #38506, #61395, #17044, #44428, #68037, #55137, #17407, #61031, #27426, #27063, #49957, #45507, #72481, #21867, #66957, #16323, #38876, #33681, #5249, #56576, #85, #67322, #10788, #33322, #27791, #50328, #72852, #22234, #44790, #16682, #39238, #22590, #61752, #39964, #56225, #50682, #45141, #10067, #39602, #5972, #51041, #437, #58370, #17756, #24035, #41406, #46584, #29945, #18845, #45861, #41051, #46221, #1528, #29588, #35129, #46949, #23674, #63922, #52848, #2246, #63564, #52126, #12231, #12596, #6700, #69486, #35845, #29233, #57654, #56928, #13307, #34400, #68395, #34760, #52485, #7781, #68760, #69127, #19205, #69840, #57295, #18118, #7060, #40682, #51766, #1165, #63200, #18485, #51402, #30318, #12952, #62478, #11876, #23312, #35489, #47305, #24762, #58009, #7417, #6332, #28863, #1896, #24400, #805, #40316, #62839, #64288, #58736, #47665, #9246, #59102, #54320, #31038, #14042, #42499, #36582, #8509, #19575, #13676, #26238, #19946, #37317, #14775, #31781, #2602, #70199, #3711, #36948, #31413, #20678, #59841, #42131, #36220, #64657, #65755, #59468, #48775, #53574, #25872, #48045, #2972, #41759, #8147, #30674, #25500, #53953, #70570, #53206, #65022, #71299, #25123, #14411, #43235, #8878, #3350, #48412, #70938, #20309, #42862, #65384, #48346, #54250, #65690, #20983, #49081, #3280, #65319, #54980, #26540, #9180, #25808, #4385, #42436, #26915, #8811, #71609, #37979, #66427, #43171, #14709, #60136, #59402, #37614, #32809, #70871, #20245, #32079, #4016, #54610, #9545, #71974, #64958, #25436, #43536, #31348, #42797, #3647, #20612, #36884, #53889, #37252, #66057, #59774, #15077, #15435, #48711, #60501, #31715, #49440, #15805, #38346, #9907, #32444, #26170, #71233, #21347, #43903, #60874, #10277, #2905, #70506, #47979, #19883, #14349, #27637, #46349, #12717, #61603, #17884, #13075, #63685, #50172, #16533, #73063, #39086, #5102, #72701, #22083, #44642, #44271, #57774, #11004, #55347, #4741, #16174, #67172, #41176, #35253, #5466, #22444, #63329, #49808, #12355, #33524, #7184, #56074, #57419, #27275, #21713, #33170, #29712, #28006, #52250, #50535, #44993, #68523, #40444, #62960, #34890, #72333, #24161, #6823, #1653, #46714, #69249, #61246, #55708, #18611, #29357, #51890, #66803, #38725, #1288, #10640, #23798, #68883, #18240, #40813, #64416, #8636, #8273, #24887, #58134, #3476, #48535, #58497, #2734, #18969, #25996, #24529, #31165, #71062, #20437, #52973, #7540, #42986, #13428, #47073, #52612, #30073, #65517, #69608, #41529, #64048, #2018, #41888, #36706, #30803, #59595, #25629, #19705, #35977, #7906, #30444, #2369, #47432, #69963, #13809, #19334, #25251, #48166, #36349, #35614, #14172, #58863, #53336, #47799, #70329, #42258, #64781 ) ),
 .UNSPECIFIED., .F., .F., .F. ) 
 B_SPLINE_SURFACE_WITH_KNOTS ( ( 2, 2 ),
 ( 3, 2, 2, 2, 2, 2, 2, 2, 2, 2, 2, 2, 2, 2, 2, 2, 2, 2, 2, 2, 2, 2, 2, 2, 2, 2, 2, 2, 2, 2, 2, 2, 2, 2, 2, 2, 2, 2, 2, 2, 2, 2, 2, 2, 2, 2, 2, 2, 2, 2, 2, 2, 2, 2, 2, 2, 2, 2, 2, 2, 2, 2, 2, 2, 2, 2, 2, 2, 2, 2, 2, 2, 2, 2, 2, 2, 2, 2, 2, 2, 2, 2, 2, 2, 2, 2, 2, 2, 2, 2, 2, 2, 2, 2, 2, 2, 2, 2, 2, 2, 2, 2, 2, 2, 2, 2, 2, 2, 2, 2, 2, 2, 2, 2, 2, 2, 2, 2, 2, 2, 2, 2, 2, 2, 2, 2, 2, 2, 2, 2, 2, 2, 2, 2, 2, 2, 2, 2, 2, 2, 2, 2, 2, 2, 2, 2, 2, 2, 2, 2, 2, 2, 2, 2, 2, 2, 2, 2, 2, 2, 2, 2, 2, 2, 2, 2, 2, 2, 2, 2, 2, 2, 2, 2, 2, 2, 2, 2, 2, 2, 2, 2, 2, 2, 2, 2, 2, 2, 2, 2, 2, 2, 2, 2, 2, 2, 2, 2, 2, 2, 2, 2, 2, 2, 2, 2, 2, 2, 2, 2, 2, 2, 2, 2, 2, 2, 2, 2, 2, 2, 2, 2, 2, 2, 2, 2, 2, 2, 2, 2, 2, 2, 2, 2, 2, 2, 2, 2, 2, 2, 2, 2, 2, 2, 2, 2, 2, 2, 2, 2, 2, 2, 2, 2, 2, 2, 2, 2, 2, 2, 2, 2, 2, 2, 2, 2, 2, 2, 2, 2, 2, 2, 2, 2, 2, 2, 2, 2, 2, 2, 2, 2, 2, 2, 2, 2, 2, 2, 2, 2, 2, 2, 2, 2, 2, 2, 2, 2, 2, 2, 3 ),
 ( 0.000000000000000000, 1.000000000000000000 ),
 ( 0.000000000000000000, 0.003333333333333333547, 0.006666666666666667095, 0.01000000000000000021, 0.01333333333333333419, 0.01666666666666666644, 0.02000000000000000042, 0.02333333333333333440, 0.02666666666666666838, 0.02999999999999999889, 0.03333333333333333287, 0.03666666666666666685, 0.04000000000000000083, 0.04333333333333333481, 0.04666666666666666879, 0.05000000000000000278, 0.05333333333333333676, 0.05666666666666666380, 0.05999999999999999778, 0.06333333333333333870, 0.06666666666666666574, 0.07000000000000000666, 0.07333333333333333370, 0.07666666666666666075, 0.08000000000000000167, 0.08333333333333332871, 0.08666666666666666963, 0.08999999999999999667, 0.09333333333333333759, 0.09666666666666666463, 0.1000000000000000056, 0.1033333333333333326, 0.1066666666666666735, 0.1100000000000000006, 0.1133333333333333276, 0.1166666666666666685, 0.1199999999999999956, 0.1233333333333333365, 0.1266666666666666774, 0.1300000000000000044, 0.1333333333333333315, 0.1366666666666666585, 0.1400000000000000133, 0.1433333333333333404, 0.1466666666666666674, 0.1499999999999999944, 0.1533333333333333215, 0.1566666666666666763, 0.1600000000000000033, 0.1633333333333333304, 0.1666666666666666574, 0.1700000000000000122, 0.1733333333333333393, 0.1766666666666666663, 0.1799999999999999933, 0.1833333333333333204, 0.1866666666666666752, 0.1900000000000000022, 0.1933333333333333293, 0.1966666666666666563, 0.2000000000000000111, 0.2033333333333333381, 0.2066666666666666652, 0.2099999999999999922, 0.2133333333333333470, 0.2166666666666666741, 0.2200000000000000011, 0.2233333333333333282, 0.2266666666666666552, 0.2300000000000000100, 0.2333333333333333370, 0.2366666666666666641, 0.2399999999999999911, 0.2433333333333333459, 0.2466666666666666730, 0.2500000000000000000, 0.2533333333333333548, 0.2566666666666666541, 0.2600000000000000089, 0.2633333333333333082, 0.2666666666666666630, 0.2700000000000000178, 0.2733333333333333171, 0.2766666666666666718, 0.2800000000000000266, 0.2833333333333333259, 0.2866666666666666807, 0.2899999999999999800, 0.2933333333333333348, 0.2966666666666666896, 0.2999999999999999889, 0.3033333333333333437, 0.3066666666666666430, 0.3099999999999999978, 0.3133333333333333526, 0.3166666666666666519, 0.3200000000000000067, 0.3233333333333333059, 0.3266666666666666607, 0.3300000000000000155, 0.3333333333333333148, 0.3366666666666666696, 0.3400000000000000244, 0.3433333333333333237, 0.3466666666666666785, 0.3499999999999999778, 0.3533333333333333326, 0.3566666666666666874, 0.3599999999999999867, 0.3633333333333333415, 0.3666666666666666408, 0.3699999999999999956, 0.3733333333333333504, 0.3766666666666666496, 0.3800000000000000044, 0.3833333333333333592, 0.3866666666666666585, 0.3900000000000000133, 0.3933333333333333126, 0.3966666666666666674, 0.4000000000000000222, 0.4033333333333333215, 0.4066666666666666763, 0.4099999999999999756, 0.4133333333333333304, 0.4166666666666666852, 0.4199999999999999845, 0.4233333333333333393, 0.4266666666666666941, 0.4299999999999999933, 0.4333333333333333481, 0.4366666666666666474, 0.4400000000000000022, 0.4433333333333333570, 0.4466666666666666563, 0.4500000000000000111, 0.4533333333333333104, 0.4566666666666666652, 0.4600000000000000200, 0.4633333333333333193, 0.4666666666666666741, 0.4699999999999999734, 0.4733333333333333282, 0.4766666666666666829, 0.4799999999999999822, 0.4833333333333333370, 0.4866666666666666918, 0.4899999999999999911, 0.4933333333333333459, 0.4966666666666666452, 0.5000000000000000000, 0.5033333333333332993, 0.5066666666666667096, 0.5100000000000000089, 0.5133333333333333082, 0.5166666666666667185, 0.5200000000000000178, 0.5233333333333333171, 0.5266666666666666163, 0.5300000000000000266, 0.5333333333333333259, 0.5366666666666666252, 0.5400000000000000355, 0.5433333333333333348, 0.5466666666666666341, 0.5500000000000000444, 0.5533333333333333437, 0.5566666666666666430, 0.5600000000000000533, 0.5633333333333333526, 0.5666666666666666519, 0.5699999999999999512, 0.5733333333333333615, 0.5766666666666666607, 0.5799999999999999600, 0.5833333333333333703, 0.5866666666666666696, 0.5899999999999999689, 0.5933333333333333792, 0.5966666666666666785, 0.5999999999999999778, 0.6033333333333333881, 0.6066666666666666874, 0.6099999999999999867, 0.6133333333333332860, 0.6166666666666666963, 0.6199999999999999956, 0.6233333333333332948, 0.6266666666666667052, 0.6300000000000000044, 0.6333333333333333037, 0.6366666666666667140, 0.6400000000000000133, 0.6433333333333333126, 0.6466666666666666119, 0.6500000000000000222, 0.6533333333333333215, 0.6566666666666666208, 0.6600000000000000311, 0.6633333333333333304, 0.6666666666666666297, 0.6700000000000000400, 0.6733333333333333393, 0.6766666666666666385, 0.6800000000000000488, 0.6833333333333333481, 0.6866666666666666474, 0.6899999999999999467, 0.6933333333333333570, 0.6966666666666666563, 0.6999999999999999556, 0.7033333333333333659, 0.7066666666666666652, 0.7099999999999999645, 0.7133333333333333748, 0.7166666666666666741, 0.7199999999999999734, 0.7233333333333333837, 0.7266666666666666829, 0.7299999999999999822, 0.7333333333333332815, 0.7366666666666666918, 0.7399999999999999911, 0.7433333333333332904, 0.7466666666666667007, 0.7500000000000000000, 0.7533333333333332993, 0.7566666666666667096, 0.7600000000000000089, 0.7633333333333333082, 0.7666666666666667185, 0.7700000000000000178, 0.7733333333333333171, 0.7766666666666666163, 0.7800000000000000266, 0.7833333333333333259, 0.7866666666666666252, 0.7900000000000000355, 0.7933333333333333348, 0.7966666666666666341, 0.8000000000000000444, 0.8033333333333333437, 0.8066666666666666430, 0.8100000000000000533, 0.8133333333333333526, 0.8166666666666666519, 0.8199999999999999512, 0.8233333333333333615, 0.8266666666666666607, 0.8299999999999999600, 0.8333333333333333703, 0.8366666666666666696, 0.8399999999999999689, 0.8433333333333333792, 0.8466666666666666785, 0.8499999999999999778, 0.8533333333333333881, 0.8566666666666666874, 0.8599999999999999867, 0.8633333333333332860, 0.8666666666666666963, 0.8699999999999999956, 0.8733333333333332948, 0.8766666666666667052, 0.8800000000000000044, 0.8833333333333333037, 0.8866666666666667140, 0.8900000000000000133, 0.8933333333333333126, 0.8966666666666666119, 0.9000000000000000222, 0.9033333333333333215, 0.9066666666666666208, 0.9100000000000000311, 0.9133333333333333304, 0.9166666666666666297, 0.9200000000000000400, 0.9233333333333333393, 0.9266666666666666385, 0.9300000000000000488, 0.9333333333333333481, 0.9366666666666666474, 0.9399999999999999467, 0.9433333333333333570, 0.9466666666666666563, 0.9499999999999999556, 0.9533333333333333659, 0.9566666666666666652, 0.9599999999999999645, 0.9633333333333333748, 0.9666666666666666741, 0.9699999999999999734, 0.9733333333333333837, 0.9766666666666666829, 0.9799999999999999822, 0.9833333333333332815, 0.9866666666666666918, 0.9899999999999999911, 0.9933333333333332904, 0.9966666666666667007, 1.000000000000000000 ),
 .UNSPECIFIED. ) 
 GEOMETRIC_REPRESENTATION_ITEM ( )  RATIONAL_B_SPLINE_SURFACE ( (
 ( 1.000000000000000000, 0.8660254037844387076, 1.000000000000000000, 0.8660254037844387076, 1.000000000000000000, 0.8660254037844387076, 1.000000000000000000, 0.8660254037844387076, 1.000000000000000000, 0.8660254037844387076, 1.000000000000000000, 0.8660254037844387076, 1.000000000000000000, 0.8660254037844387076, 1.000000000000000000, 0.8660254037844387076, 1.000000000000000000, 0.8660254037844387076, 1.000000000000000000, 0.8660254037844387076, 1.000000000000000000, 0.8660254037844387076, 1.000000000000000000, 0.8660254037844387076, 1.000000000000000000, 0.8660254037844387076, 1.000000000000000000, 0.8660254037844387076, 1.000000000000000000, 0.8660254037844387076, 1.000000000000000000, 0.8660254037844387076, 1.000000000000000000, 0.8660254037844387076, 1.000000000000000000, 0.8660254037844387076, 1.000000000000000000, 0.8660254037844387076, 1.000000000000000000, 0.8660254037844387076, 1.000000000000000000, 0.8660254037844387076, 1.000000000000000000, 0.8660254037844387076, 1.000000000000000000, 0.8660254037844387076, 1.000000000000000000, 0.8660254037844387076, 1.000000000000000000, 0.8660254037844387076, 1.000000000000000000, 0.8660254037844387076, 1.000000000000000000, 0.8660254037844387076, 1.000000000000000000, 0.8660254037844387076, 1.000000000000000000, 0.8660254037844387076, 1.000000000000000000, 0.8660254037844387076, 1.000000000000000000, 0.8660254037844387076, 1.000000000000000000, 0.8660254037844387076, 1.000000000000000000, 0.8660254037844387076, 1.000000000000000000, 0.8660254037844387076, 1.000000000000000000, 0.8660254037844387076, 1.000000000000000000, 0.8660254037844387076, 1.000000000000000000, 0.8660254037844387076, 1.000000000000000000, 0.8660254037844387076, 1.000000000000000000, 0.8660254037844387076, 1.000000000000000000, 0.8660254037844387076, 1.000000000000000000, 0.8660254037844387076, 1.000000000000000000, 0.8660254037844387076, 1.000000000000000000, 0.8660254037844387076, 1.000000000000000000, 0.8660254037844387076, 1.000000000000000000, 0.8660254037844387076, 1.000000000000000000, 0.8660254037844387076, 1.000000000000000000, 0.8660254037844387076, 1.000000000000000000, 0.8660254037844387076, 1.000000000000000000, 0.8660254037844387076, 1.000000000000000000, 0.8660254037844387076, 1.000000000000000000, 0.8660254037844387076, 1.000000000000000000, 0.8660254037844387076, 1.000000000000000000, 0.8660254037844387076, 1.000000000000000000, 0.8660254037844387076, 1.000000000000000000, 0.8660254037844387076, 1.000000000000000000, 0.8660254037844387076, 1.000000000000000000, 0.8660254037844387076, 1.000000000000000000, 0.8660254037844387076, 1.000000000000000000, 0.8660254037844387076, 1.000000000000000000, 0.8660254037844387076, 1.000000000000000000, 0.8660254037844387076, 1.000000000000000000, 0.8660254037844387076, 1.000000000000000000, 0.8660254037844387076, 1.000000000000000000, 0.8660254037844387076, 1.000000000000000000, 0.8660254037844387076, 1.000000000000000000, 0.8660254037844387076, 1.000000000000000000, 0.8660254037844387076, 1.000000000000000000, 0.8660254037844387076, 1.000000000000000000, 0.8660254037844387076, 1.000000000000000000, 0.8660254037844387076, 1.000000000000000000, 0.8660254037844387076, 1.000000000000000000, 0.8660254037844387076, 1.000000000000000000, 0.8660254037844387076, 1.000000000000000000, 0.8660254037844387076, 1.000000000000000000, 0.8660254037844387076, 1.000000000000000000, 0.8660254037844387076, 1.000000000000000000, 0.8660254037844387076, 1.000000000000000000, 0.8660254037844387076, 1.000000000000000000, 0.8660254037844387076, 1.000000000000000000, 0.8660254037844387076, 1.000000000000000000, 0.8660254037844387076, 1.000000000000000000, 0.8660254037844387076, 1.000000000000000000, 0.8660254037844387076, 1.000000000000000000, 0.8660254037844387076, 1.000000000000000000, 0.8660254037844387076, 1.000000000000000000, 0.8660254037844387076, 1.000000000000000000, 0.8660254037844387076, 1.000000000000000000, 0.8660254037844387076, 1.000000000000000000, 0.8660254037844387076, 1.000000000000000000, 0.8660254037844387076, 1.000000000000000000, 0.8660254037844387076, 1.000000000000000000, 0.8660254037844387076, 1.000000000000000000, 0.8660254037844387076, 1.000000000000000000, 0.8660254037844387076, 1.000000000000000000, 0.8660254037844387076, 1.000000000000000000, 0.8660254037844387076, 1.000000000000000000, 0.8660254037844387076, 1.000000000000000000, 0.8660254037844387076, 1.000000000000000000, 0.8660254037844387076, 1.000000000000000000, 0.8660254037844387076, 1.000000000000000000, 0.8660254037844387076, 1.000000000000000000, 0.8660254037844387076, 1.000000000000000000, 0.8660254037844387076, 1.000000000000000000, 0.8660254037844387076, 1.000000000000000000, 0.8660254037844387076, 1.000000000000000000, 0.8660254037844387076, 1.000000000000000000, 0.8660254037844387076, 1.000000000000000000, 0.8660254037844387076, 1.000000000000000000, 0.8660254037844387076, 1.000000000000000000, 0.8660254037844387076, 1.000000000000000000, 0.8660254037844387076, 1.000000000000000000, 0.8660254037844387076, 1.000000000000000000, 0.8660254037844387076, 1.000000000000000000, 0.8660254037844387076, 1.000000000000000000, 0.8660254037844387076, 1.000000000000000000, 0.8660254037844387076, 1.000000000000000000, 0.8660254037844387076, 1.000000000000000000, 0.8660254037844387076, 1.000000000000000000, 0.8660254037844387076, 1.000000000000000000, 0.8660254037844387076, 1.000000000000000000, 0.8660254037844387076, 1.000000000000000000, 0.8660254037844387076, 1.000000000000000000, 0.8660254037844387076, 1.000000000000000000, 0.8660254037844387076, 1.000000000000000000, 0.8660254037844387076, 1.000000000000000000, 0.8660254037844387076, 1.000000000000000000, 0.8660254037844387076, 1.000000000000000000, 0.8660254037844387076, 1.000000000000000000, 0.8660254037844387076, 1.000000000000000000, 0.8660254037844387076, 1.000000000000000000, 0.8660254037844387076, 1.000000000000000000, 0.8660254037844387076, 1.000000000000000000, 0.8660254037844387076, 1.000000000000000000, 0.8660254037844387076, 1.000000000000000000, 0.8660254037844387076, 1.000000000000000000, 0.8660254037844387076, 1.000000000000000000, 0.8660254037844387076, 1.000000000000000000, 0.8660254037844387076, 1.000000000000000000, 0.8660254037844387076, 1.000000000000000000, 0.8660254037844387076, 1.000000000000000000, 0.8660254037844387076, 1.000000000000000000, 0.8660254037844387076, 1.000000000000000000, 0.8660254037844387076, 1.000000000000000000, 0.8660254037844387076, 1.000000000000000000, 0.8660254037844387076, 1.000000000000000000, 0.8660254037844387076, 1.000000000000000000, 0.8660254037844387076, 1.000000000000000000, 0.8660254037844387076, 1.000000000000000000, 0.8660254037844387076, 1.000000000000000000, 0.8660254037844387076, 1.000000000000000000, 0.8660254037844387076, 1.000000000000000000, 0.8660254037844387076, 1.000000000000000000, 0.8660254037844387076, 1.000000000000000000, 0.8660254037844387076, 1.000000000000000000, 0.8660254037844387076, 1.000000000000000000, 0.8660254037844387076, 1.000000000000000000, 0.8660254037844387076, 1.000000000000000000, 0.8660254037844387076, 1.000000000000000000, 0.8660254037844387076, 1.000000000000000000, 0.8660254037844387076, 1.000000000000000000, 0.8660254037844387076, 1.000000000000000000, 0.8660254037844387076, 1.000000000000000000, 0.8660254037844387076, 1.000000000000000000, 0.8660254037844387076, 1.000000000000000000, 0.8660254037844387076, 1.000000000000000000, 0.8660254037844387076, 1.000000000000000000, 0.8660254037844387076, 1.000000000000000000, 0.8660254037844387076, 1.000000000000000000, 0.8660254037844387076, 1.000000000000000000, 0.8660254037844387076, 1.000000000000000000, 0.8660254037844387076, 1.000000000000000000, 0.8660254037844387076, 1.000000000000000000, 0.8660254037844387076, 1.000000000000000000, 0.8660254037844387076, 1.000000000000000000, 0.8660254037844387076, 1.000000000000000000, 0.8660254037844387076, 1.000000000000000000, 0.8660254037844387076, 1.000000000000000000, 0.8660254037844387076, 1.000000000000000000, 0.8660254037844387076, 1.000000000000000000, 0.8660254037844387076, 1.000000000000000000, 0.8660254037844387076, 1.000000000000000000, 0.8660254037844387076, 1.000000000000000000, 0.8660254037844387076, 1.000000000000000000, 0.8660254037844387076, 1.000000000000000000, 0.8660254037844387076, 1.000000000000000000, 0.8660254037844387076, 1.000000000000000000, 0.8660254037844387076, 1.000000000000000000, 0.8660254037844387076, 1.000000000000000000, 0.8660254037844387076, 1.000000000000000000, 0.8660254037844387076, 1.000000000000000000, 0.8660254037844387076, 1.000000000000000000, 0.8660254037844387076, 1.000000000000000000, 0.8660254037844387076, 1.000000000000000000, 0.8660254037844387076, 1.000000000000000000, 0.8660254037844387076, 1.000000000000000000, 0.8660254037844387076, 1.000000000000000000, 0.8660254037844387076, 1.000000000000000000, 0.8660254037844387076, 1.000000000000000000, 0.8660254037844387076, 1.000000000000000000, 0.8660254037844387076, 1.000000000000000000, 0.8660254037844387076, 1.000000000000000000, 0.8660254037844387076, 1.000000000000000000, 0.8660254037844387076, 1.000000000000000000, 0.8660254037844387076, 1.000000000000000000, 0.8660254037844387076, 1.000000000000000000, 0.8660254037844387076, 1.000000000000000000, 0.8660254037844387076, 1.000000000000000000, 0.8660254037844387076, 1.000000000000000000, 0.8660254037844387076, 1.000000000000000000, 0.8660254037844387076, 1.000000000000000000, 0.8660254037844387076, 1.000000000000000000, 0.8660254037844387076, 1.000000000000000000, 0.8660254037844387076, 1.000000000000000000, 0.8660254037844387076, 1.000000000000000000, 0.8660254037844387076, 1.000000000000000000, 0.8660254037844387076, 1.000000000000000000, 0.8660254037844387076, 1.000000000000000000, 0.8660254037844387076, 1.000000000000000000, 0.8660254037844387076, 1.000000000000000000, 0.8660254037844387076, 1.000000000000000000, 0.8660254037844387076, 1.000000000000000000, 0.8660254037844387076, 1.000000000000000000, 0.8660254037844387076, 1.000000000000000000, 0.8660254037844387076, 1.000000000000000000, 0.8660254037844387076, 1.000000000000000000, 0.8660254037844387076, 1.000000000000000000, 0.8660254037844387076, 1.000000000000000000, 0.8660254037844387076, 1.000000000000000000, 0.8660254037844387076, 1.000000000000000000, 0.8660254037844387076, 1.000000000000000000, 0.8660254037844387076, 1.000000000000000000, 0.8660254037844387076, 1.000000000000000000, 0.8660254037844387076, 1.000000000000000000, 0.8660254037844387076, 1.000000000000000000, 0.8660254037844387076, 1.000000000000000000, 0.8660254037844387076, 1.000000000000000000, 0.8660254037844387076, 1.000000000000000000, 0.8660254037844387076, 1.000000000000000000, 0.8660254037844387076, 1.000000000000000000, 0.8660254037844387076, 1.000000000000000000, 0.8660254037844387076, 1.000000000000000000, 0.8660254037844387076, 1.000000000000000000, 0.8660254037844387076, 1.000000000000000000, 0.8660254037844387076, 1.000000000000000000, 0.8660254037844387076, 1.000000000000000000, 0.8660254037844387076, 1.000000000000000000, 0.8660254037844387076, 1.000000000000000000, 0.8660254037844387076, 1.000000000000000000, 0.8660254037844387076, 1.000000000000000000, 0.8660254037844387076, 1.000000000000000000, 0.8660254037844387076, 1.000000000000000000, 0.8660254037844387076, 1.000000000000000000, 0.8660254037844387076, 1.000000000000000000, 0.8660254037844387076, 1.000000000000000000, 0.8660254037844387076, 1.000000000000000000, 0.8660254037844387076, 1.000000000000000000, 0.8660254037844387076, 1.000000000000000000, 0.8660254037844387076, 1.000000000000000000, 0.8660254037844387076, 1.000000000000000000, 0.8660254037844387076, 1.000000000000000000, 0.8660254037844387076, 1.000000000000000000, 0.8660254037844387076, 1.000000000000000000, 0.8660254037844387076, 1.000000000000000000, 0.8660254037844387076, 1.000000000000000000, 0.8660254037844387076, 1.000000000000000000, 0.8660254037844387076, 1.000000000000000000, 0.8660254037844387076, 1.000000000000000000, 0.8660254037844387076, 1.000000000000000000, 0.8660254037844387076, 1.000000000000000000, 0.8660254037844387076, 1.000000000000000000, 0.8660254037844387076, 1.000000000000000000, 0.8660254037844387076, 1.000000000000000000, 0.8660254037844387076, 1.000000000000000000, 0.8660254037844387076, 1.000000000000000000, 0.8660254037844387076, 1.000000000000000000, 0.8660254037844387076, 1.000000000000000000, 0.8660254037844387076, 1.000000000000000000, 0.8660254037844387076, 1.000000000000000000, 0.8660254037844387076, 1.000000000000000000, 0.8660254037844387076, 1.000000000000000000, 0.8660254037844387076, 1.000000000000000000, 0.8660254037844387076, 1.000000000000000000, 0.8660254037844387076, 1.000000000000000000, 0.8660254037844387076, 1.000000000000000000, 0.8660254037844387076, 1.000000000000000000, 0.8660254037844387076, 1.000000000000000000, 0.8660254037844387076, 1.000000000000000000, 0.8660254037844387076, 1.000000000000000000, 0.8660254037844387076, 1.000000000000000000, 0.8660254037844387076, 1.000000000000000000, 0.8660254037844387076, 1.000000000000000000, 0.8660254037844387076, 1.000000000000000000, 0.8660254037844387076, 1.000000000000000000, 0.8660254037844387076, 1.000000000000000000, 0.8660254037844387076, 1.000000000000000000, 0.8660254037844387076, 1.000000000000000000, 0.8660254037844387076, 1.000000000000000000, 0.8660254037844387076, 1.000000000000000000, 0.8660254037844387076, 1.000000000000000000, 0.8660254037844387076, 1.000000000000000000),
 ( 1.000000000000000000, 0.8660254037844387076, 1.000000000000000000, 0.8660254037844387076, 1.000000000000000000, 0.8660254037844387076, 1.000000000000000000, 0.8660254037844387076, 1.000000000000000000, 0.8660254037844387076, 1.000000000000000000, 0.8660254037844387076, 1.000000000000000000, 0.8660254037844387076, 1.000000000000000000, 0.8660254037844387076, 1.000000000000000000, 0.8660254037844387076, 1.000000000000000000, 0.8660254037844387076, 1.000000000000000000, 0.8660254037844387076, 1.000000000000000000, 0.8660254037844387076, 1.000000000000000000, 0.8660254037844387076, 1.000000000000000000, 0.8660254037844387076, 1.000000000000000000, 0.8660254037844387076, 1.000000000000000000, 0.8660254037844387076, 1.000000000000000000, 0.8660254037844387076, 1.000000000000000000, 0.8660254037844387076, 1.000000000000000000, 0.8660254037844387076, 1.000000000000000000, 0.8660254037844387076, 1.000000000000000000, 0.8660254037844387076, 1.000000000000000000, 0.8660254037844387076, 1.000000000000000000, 0.8660254037844387076, 1.000000000000000000, 0.8660254037844387076, 1.000000000000000000, 0.8660254037844387076, 1.000000000000000000, 0.8660254037844387076, 1.000000000000000000, 0.8660254037844387076, 1.000000000000000000, 0.8660254037844387076, 1.000000000000000000, 0.8660254037844387076, 1.000000000000000000, 0.8660254037844387076, 1.000000000000000000, 0.8660254037844387076, 1.000000000000000000, 0.8660254037844387076, 1.000000000000000000, 0.8660254037844387076, 1.000000000000000000, 0.8660254037844387076, 1.000000000000000000, 0.8660254037844387076, 1.000000000000000000, 0.8660254037844387076, 1.000000000000000000, 0.8660254037844387076, 1.000000000000000000, 0.8660254037844387076, 1.000000000000000000, 0.8660254037844387076, 1.000000000000000000, 0.8660254037844387076, 1.000000000000000000, 0.8660254037844387076, 1.000000000000000000, 0.8660254037844387076, 1.000000000000000000, 0.8660254037844387076, 1.000000000000000000, 0.8660254037844387076, 1.000000000000000000, 0.8660254037844387076, 1.000000000000000000, 0.8660254037844387076, 1.000000000000000000, 0.8660254037844387076, 1.000000000000000000, 0.8660254037844387076, 1.000000000000000000, 0.8660254037844387076, 1.000000000000000000, 0.8660254037844387076, 1.000000000000000000, 0.8660254037844387076, 1.000000000000000000, 0.8660254037844387076, 1.000000000000000000, 0.8660254037844387076, 1.000000000000000000, 0.8660254037844387076, 1.000000000000000000, 0.8660254037844387076, 1.000000000000000000, 0.8660254037844387076, 1.000000000000000000, 0.8660254037844387076, 1.000000000000000000, 0.8660254037844387076, 1.000000000000000000, 0.8660254037844387076, 1.000000000000000000, 0.8660254037844387076, 1.000000000000000000, 0.8660254037844387076, 1.000000000000000000, 0.8660254037844387076, 1.000000000000000000, 0.8660254037844387076, 1.000000000000000000, 0.8660254037844387076, 1.000000000000000000, 0.8660254037844387076, 1.000000000000000000, 0.8660254037844387076, 1.000000000000000000, 0.8660254037844387076, 1.000000000000000000, 0.8660254037844387076, 1.000000000000000000, 0.8660254037844387076, 1.000000000000000000, 0.8660254037844387076, 1.000000000000000000, 0.8660254037844387076, 1.000000000000000000, 0.8660254037844387076, 1.000000000000000000, 0.8660254037844387076, 1.000000000000000000, 0.8660254037844387076, 1.000000000000000000, 0.8660254037844387076, 1.000000000000000000, 0.8660254037844387076, 1.000000000000000000, 0.8660254037844387076, 1.000000000000000000, 0.8660254037844387076, 1.000000000000000000, 0.8660254037844387076, 1.000000000000000000, 0.8660254037844387076, 1.000000000000000000, 0.8660254037844387076, 1.000000000000000000, 0.8660254037844387076, 1.000000000000000000, 0.8660254037844387076, 1.000000000000000000, 0.8660254037844387076, 1.000000000000000000, 0.8660254037844387076, 1.000000000000000000, 0.8660254037844387076, 1.000000000000000000, 0.8660254037844387076, 1.000000000000000000, 0.8660254037844387076, 1.000000000000000000, 0.8660254037844387076, 1.000000000000000000, 0.8660254037844387076, 1.000000000000000000, 0.8660254037844387076, 1.000000000000000000, 0.8660254037844387076, 1.000000000000000000, 0.8660254037844387076, 1.000000000000000000, 0.8660254037844387076, 1.000000000000000000, 0.8660254037844387076, 1.000000000000000000, 0.8660254037844387076, 1.000000000000000000, 0.8660254037844387076, 1.000000000000000000, 0.8660254037844387076, 1.000000000000000000, 0.8660254037844387076, 1.000000000000000000, 0.8660254037844387076, 1.000000000000000000, 0.8660254037844387076, 1.000000000000000000, 0.8660254037844387076, 1.000000000000000000, 0.8660254037844387076, 1.000000000000000000, 0.8660254037844387076, 1.000000000000000000, 0.8660254037844387076, 1.000000000000000000, 0.8660254037844387076, 1.000000000000000000, 0.8660254037844387076, 1.000000000000000000, 0.8660254037844387076, 1.000000000000000000, 0.8660254037844387076, 1.000000000000000000, 0.8660254037844387076, 1.000000000000000000, 0.8660254037844387076, 1.000000000000000000, 0.8660254037844387076, 1.000000000000000000, 0.8660254037844387076, 1.000000000000000000, 0.8660254037844387076, 1.000000000000000000, 0.8660254037844387076, 1.000000000000000000, 0.8660254037844387076, 1.000000000000000000, 0.8660254037844387076, 1.000000000000000000, 0.8660254037844387076, 1.000000000000000000, 0.8660254037844387076, 1.000000000000000000, 0.8660254037844387076, 1.000000000000000000, 0.8660254037844387076, 1.000000000000000000, 0.8660254037844387076, 1.000000000000000000, 0.8660254037844387076, 1.000000000000000000, 0.8660254037844387076, 1.000000000000000000, 0.8660254037844387076, 1.000000000000000000, 0.8660254037844387076, 1.000000000000000000, 0.8660254037844387076, 1.000000000000000000, 0.8660254037844387076, 1.000000000000000000, 0.8660254037844387076, 1.000000000000000000, 0.8660254037844387076, 1.000000000000000000, 0.8660254037844387076, 1.000000000000000000, 0.8660254037844387076, 1.000000000000000000, 0.8660254037844387076, 1.000000000000000000, 0.8660254037844387076, 1.000000000000000000, 0.8660254037844387076, 1.000000000000000000, 0.8660254037844387076, 1.000000000000000000, 0.8660254037844387076, 1.000000000000000000, 0.8660254037844387076, 1.000000000000000000, 0.8660254037844387076, 1.000000000000000000, 0.8660254037844387076, 1.000000000000000000, 0.8660254037844387076, 1.000000000000000000, 0.8660254037844387076, 1.000000000000000000, 0.8660254037844387076, 1.000000000000000000, 0.8660254037844387076, 1.000000000000000000, 0.8660254037844387076, 1.000000000000000000, 0.8660254037844387076, 1.000000000000000000, 0.8660254037844387076, 1.000000000000000000, 0.8660254037844387076, 1.000000000000000000, 0.8660254037844387076, 1.000000000000000000, 0.8660254037844387076, 1.000000000000000000, 0.8660254037844387076, 1.000000000000000000, 0.8660254037844387076, 1.000000000000000000, 0.8660254037844387076, 1.000000000000000000, 0.8660254037844387076, 1.000000000000000000, 0.8660254037844387076, 1.000000000000000000, 0.8660254037844387076, 1.000000000000000000, 0.8660254037844387076, 1.000000000000000000, 0.8660254037844387076, 1.000000000000000000, 0.8660254037844387076, 1.000000000000000000, 0.8660254037844387076, 1.000000000000000000, 0.8660254037844387076, 1.000000000000000000, 0.8660254037844387076, 1.000000000000000000, 0.8660254037844387076, 1.000000000000000000, 0.8660254037844387076, 1.000000000000000000, 0.8660254037844387076, 1.000000000000000000, 0.8660254037844387076, 1.000000000000000000, 0.8660254037844387076, 1.000000000000000000, 0.8660254037844387076, 1.000000000000000000, 0.8660254037844387076, 1.000000000000000000, 0.8660254037844387076, 1.000000000000000000, 0.8660254037844387076, 1.000000000000000000, 0.8660254037844387076, 1.000000000000000000, 0.8660254037844387076, 1.000000000000000000, 0.8660254037844387076, 1.000000000000000000, 0.8660254037844387076, 1.000000000000000000, 0.8660254037844387076, 1.000000000000000000, 0.8660254037844387076, 1.000000000000000000, 0.8660254037844387076, 1.000000000000000000, 0.8660254037844387076, 1.000000000000000000, 0.8660254037844387076, 1.000000000000000000, 0.8660254037844387076, 1.000000000000000000, 0.8660254037844387076, 1.000000000000000000, 0.8660254037844387076, 1.000000000000000000, 0.8660254037844387076, 1.000000000000000000, 0.8660254037844387076, 1.000000000000000000, 0.8660254037844387076, 1.000000000000000000, 0.8660254037844387076, 1.000000000000000000, 0.8660254037844387076, 1.000000000000000000, 0.8660254037844387076, 1.000000000000000000, 0.8660254037844387076, 1.000000000000000000, 0.8660254037844387076, 1.000000000000000000, 0.8660254037844387076, 1.000000000000000000, 0.8660254037844387076, 1.000000000000000000, 0.8660254037844387076, 1.000000000000000000, 0.8660254037844387076, 1.000000000000000000, 0.8660254037844387076, 1.000000000000000000, 0.8660254037844387076, 1.000000000000000000, 0.8660254037844387076, 1.000000000000000000, 0.8660254037844387076, 1.000000000000000000, 0.8660254037844387076, 1.000000000000000000, 0.8660254037844387076, 1.000000000000000000, 0.8660254037844387076, 1.000000000000000000, 0.8660254037844387076, 1.000000000000000000, 0.8660254037844387076, 1.000000000000000000, 0.8660254037844387076, 1.000000000000000000, 0.8660254037844387076, 1.000000000000000000, 0.8660254037844387076, 1.000000000000000000, 0.8660254037844387076, 1.000000000000000000, 0.8660254037844387076, 1.000000000000000000, 0.8660254037844387076, 1.000000000000000000, 0.8660254037844387076, 1.000000000000000000, 0.8660254037844387076, 1.000000000000000000, 0.8660254037844387076, 1.000000000000000000, 0.8660254037844387076, 1.000000000000000000, 0.8660254037844387076, 1.000000000000000000, 0.8660254037844387076, 1.000000000000000000, 0.8660254037844387076, 1.000000000000000000, 0.8660254037844387076, 1.000000000000000000, 0.8660254037844387076, 1.000000000000000000, 0.8660254037844387076, 1.000000000000000000, 0.8660254037844387076, 1.000000000000000000, 0.8660254037844387076, 1.000000000000000000, 0.8660254037844387076, 1.000000000000000000, 0.8660254037844387076, 1.000000000000000000, 0.8660254037844387076, 1.000000000000000000, 0.8660254037844387076, 1.000000000000000000, 0.8660254037844387076, 1.000000000000000000, 0.8660254037844387076, 1.000000000000000000, 0.8660254037844387076, 1.000000000000000000, 0.8660254037844387076, 1.000000000000000000, 0.8660254037844387076, 1.000000000000000000, 0.8660254037844387076, 1.000000000000000000, 0.8660254037844387076, 1.000000000000000000, 0.8660254037844387076, 1.000000000000000000, 0.8660254037844387076, 1.000000000000000000, 0.8660254037844387076, 1.000000000000000000, 0.8660254037844387076, 1.000000000000000000, 0.8660254037844387076, 1.000000000000000000, 0.8660254037844387076, 1.000000000000000000, 0.8660254037844387076, 1.000000000000000000, 0.8660254037844387076, 1.000000000000000000, 0.8660254037844387076, 1.000000000000000000, 0.8660254037844387076, 1.000000000000000000, 0.8660254037844387076, 1.000000000000000000, 0.8660254037844387076, 1.000000000000000000, 0.8660254037844387076, 1.000000000000000000, 0.8660254037844387076, 1.000000000000000000, 0.8660254037844387076, 1.000000000000000000, 0.8660254037844387076, 1.000000000000000000, 0.8660254037844387076, 1.000000000000000000, 0.8660254037844387076, 1.000000000000000000, 0.8660254037844387076, 1.000000000000000000, 0.8660254037844387076, 1.000000000000000000, 0.8660254037844387076, 1.000000000000000000, 0.8660254037844387076, 1.000000000000000000, 0.8660254037844387076, 1.000000000000000000, 0.8660254037844387076, 1.000000000000000000, 0.8660254037844387076, 1.000000000000000000, 0.8660254037844387076, 1.000000000000000000, 0.8660254037844387076, 1.000000000000000000, 0.8660254037844387076, 1.000000000000000000, 0.8660254037844387076, 1.000000000000000000, 0.8660254037844387076, 1.000000000000000000, 0.8660254037844387076, 1.000000000000000000, 0.8660254037844387076, 1.000000000000000000, 0.8660254037844387076, 1.000000000000000000, 0.8660254037844387076, 1.000000000000000000, 0.8660254037844387076, 1.000000000000000000, 0.8660254037844387076, 1.000000000000000000, 0.8660254037844387076, 1.000000000000000000, 0.8660254037844387076, 1.000000000000000000, 0.8660254037844387076, 1.000000000000000000, 0.8660254037844387076, 1.000000000000000000, 0.8660254037844387076, 1.000000000000000000, 0.8660254037844387076, 1.000000000000000000, 0.8660254037844387076, 1.000000000000000000, 0.8660254037844387076, 1.000000000000000000, 0.8660254037844387076, 1.000000000000000000, 0.8660254037844387076, 1.000000000000000000, 0.8660254037844387076, 1.000000000000000000, 0.8660254037844387076, 1.000000000000000000, 0.8660254037844387076, 1.000000000000000000, 0.8660254037844387076, 1.000000000000000000, 0.8660254037844387076, 1.000000000000000000, 0.8660254037844387076, 1.000000000000000000, 0.8660254037844387076, 1.000000000000000000, 0.8660254037844387076, 1.000000000000000000, 0.8660254037844387076, 1.000000000000000000, 0.8660254037844387076, 1.000000000000000000, 0.8660254037844387076, 1.000000000000000000, 0.8660254037844387076, 1.000000000000000000, 0.8660254037844387076, 1.000000000000000000, 0.8660254037844387076, 1.000000000000000000, 0.8660254037844387076, 1.000000000000000000, 0.8660254037844387076, 1.000000000000000000, 0.8660254037844387076, 1.000000000000000000, 0.8660254037844387076, 1.000000000000000000, 0.8660254037844387076, 1.000000000000000000, 0.8660254037844387076, 1.000000000000000000, 0.8660254037844387076, 1.000000000000000000) ) ) 
 REPRESENTATION_ITEM ( '' )  SURFACE ( )  );
#67018=DIRECTION ( 'NONE',  ( 0.000000000000000000, 0.000000000000000000, 1.000000000000000000 ) ) ;
#67026=CARTESIAN_POINT ( 'NONE',  ( 19.21875000122902932, 2.886751345948126879, 4.999999999999999112 ) ) ;
#67043=CARTESIAN_POINT ( 'NONE',  ( 26.25937500061451857, 0.000000000000000000, 4.756430356249998326 ) ) ;
#67050=CARTESIAN_POINT ( 'NONE',  ( 27.22499999999999787, 4.330127018922191873, 2.499999999999999556 ) ) ;
#67056=CARTESIAN_POINT ( 'NONE',  ( 8.662499999999997868, 2.886751345948073588, -5.000000000000094147 ) ) ;
#67058=CARTESIAN_POINT ( 'NONE',  ( 12.43125000122903145, 4.330127018922191873, 2.499999999999999556 ) ) ;
#67062=CARTESIAN_POINT ( 'NONE',  ( 21.45937500061451786, 2.746126346562645981, -4.756430356249997438 ) ) ;
#67065=EDGE_LOOP ( 'NONE', ( #37653, #41154, #21941, #51619 ) ) ;
#67072=CARTESIAN_POINT ( 'NONE',  ( 11.78437500061451360, -2.746126346562646425, 4.756430356249996549 ) ) ;
#67096=CARTESIAN_POINT ( 'NONE',  ( 16.02187500061451786, -5.492252693125287522, -1.008910452111647106E-15 ) ) ;
#67102=CARTESIAN_POINT ( 'NONE',  ( 10.49999999999999822, 4.330127018922192761, -2.499999999999997780 ) ) ;
#67115=CARTESIAN_POINT ( 'NONE',  ( 25.33125000122903003, 6.123233995736764310E-16, -4.999999999999998224 ) ) ;
#67122=ADVANCED_FACE ( 'NONE', ( #66286 ), #15664, .T. ) ;
#67141=CARTESIAN_POINT ( 'NONE',  ( 45.00000000000000000, 0.000000000000000000, 0.000000000000000000 ) ) ;
#67154=CARTESIAN_POINT ( 'NONE',  ( 28.96875000122903288, 2.886751345948158409, -4.999999999999947597 ) ) ;
#67162=CARTESIAN_POINT ( 'NONE',  ( 21.15937500061451715, 2.746126346562643317, 4.756430356249998326 ) ) ;
#67170=ORIENTED_EDGE ( 'NONE', *, *, #49427, .F. ) ;
#67172=CARTESIAN_POINT ( 'NONE',  ( 11.02500000000000036, 4.330127018922191873, 2.499999999999999556 ) ) ;
#67179=CARTESIAN_POINT ( 'NONE',  ( 22.02187500061452141, 2.746126346562645981, -4.756430356249997438 ) ) ;
#67182=CARTESIAN_POINT ( 'NONE',  ( 12.82499999999999929, 4.330127018922191873, 2.499999999999999556 ) ) ;
#67201=CARTESIAN_POINT ( 'NONE',  ( 8.709375000614517859, 0.000000000000000000, 4.756430356249998326 ) ) ;
#67209=ORIENTED_EDGE ( 'NONE', *, *, #17293, .F. ) ;
#67223=CARTESIAN_POINT ( 'NONE',  ( 11.59687500061451892, -2.746126346562642428, -4.756430356249999214 ) ) ;
#67237=LINE ( 'NONE', #39149, #38348 ) ;
#67238=EDGE_CURVE ( 'NONE', #56470, #9094, #22309, .T. ) ;
#67245=CARTESIAN_POINT ( 'NONE',  ( 19.35937500061451644, 2.746126346562643317, 4.756430356249998326 ) ) ;
#67248=CARTESIAN_POINT ( 'NONE',  ( 14.94375000122903252, -2.886751345948125991, -5.000000000000000000 ) ) ;
#67256=CARTESIAN_POINT ( 'NONE',  ( 17.39999999999999858, 0.000000000000000000, 4.999999999999998224 ) ) ;
#67263=CARTESIAN_POINT ( 'NONE',  ( 7.959375000614516082, 2.746126346562645981, -4.756430356249997438 ) ) ;
#67285=CARTESIAN_POINT ( 'NONE',  ( 17.25937500061451502, 0.000000000000000000, 4.756430356249998326 ) ) ;
#67289=VERTEX_POINT ( 'NONE', #52199 ) ;
#67290=EDGE_CURVE ( 'NONE', #66820, #26491, #16433, .T. ) ;
#67317=CARTESIAN_POINT ( 'NONE',  ( 18.60937500061451644, 0.000000000000000000, 4.756430356249998326 ) ) ;
#67322=CARTESIAN_POINT ( 'NONE',  ( 19.42499999999999716, 6.123233995736764310E-16, -4.999999999999998224 ) ) ;
#67326=CARTESIAN_POINT ( 'NONE',  ( 26.48437500061450933, 5.492252693125287522, 3.363034840372157021E-16 ) ) ;
#67333=CARTESIAN_POINT ( 'NONE',  ( 28.39687500061451431, 0.000000000000000000, 4.756430356249998326 ) ) ;
#67335=CARTESIAN_POINT ( 'NONE',  ( 14.67187500061451644, 5.824947211148865298E-16, -4.756430356249998326 ) ) ;
#67338=VERTEX_POINT ( 'NONE', #17481 ) ;
#67344=CARTESIAN_POINT ( 'NONE',  ( 20.83125000122903359, 6.123233995736764310E-16, -4.999999999999998224 ) ) ;
#67358=DIRECTION ( 'NONE',  ( -1.000000000000000000, -0.000000000000000000, -0.000000000000000000 ) ) ;
#67368=CARTESIAN_POINT ( 'NONE',  ( 23.37187500061451573, 2.746126346562645981, -4.756430356249997438 ) ) ;
#67375=VERTEX_POINT ( 'NONE', #6775 ) ;
#67376=CARTESIAN_POINT ( 'NONE',  ( 20.06250000000000000, 2.886751345948126879, 4.999999999999998224 ) ) ;
#67387=CARTESIAN_POINT ( 'NONE',  ( 19.14375000122903003, 5.773502691896255534, 3.535250795749688894E-16 ) ) ;
#67398=( BOUNDED_CURVE ( )  B_SPLINE_CURVE ( 2, ( #34823, #17464, #50741, #5676, #865, #6393, #16742 ),
 .UNSPECIFIED., .F., .F. ) 
 B_SPLINE_CURVE_WITH_KNOTS ( ( 3, 2, 2, 3 ),
 ( 0.6400000000000001243, 0.6433333333333334236, 0.6466666666666666119, 0.6500000000000000222 ),
 .UNSPECIFIED. ) 
 CURVE ( )  GEOMETRIC_REPRESENTATION_ITEM ( )  RATIONAL_B_SPLINE_CURVE ( ( 0.9999999999999955591, 0.8660254037844431485, 1.000000000000000000, 0.8660254037844387076, 1.000000000000000000, 0.8660254037844387076, 1.000000000000000000 ) ) 
 REPRESENTATION_ITEM ( '' )  );
#67404=CARTESIAN_POINT ( 'NONE',  ( 26.82187500061451857, -5.492252693125287522, -1.008910452111647106E-15 ) ) ;
#67409=CARTESIAN_POINT ( 'NONE',  ( 25.87500000000000000, 4.330127018922191873, 2.499999999999999556 ) ) ;
#67415=CARTESIAN_POINT ( 'NONE',  ( 45.00000000000000000, 6.123233995736764310E-16, -4.999999999999998224 ) ) ;
#67417=CARTESIAN_POINT ( 'NONE',  ( 12.28125000122903110, 6.123233995736764310E-16, -4.999999999999998224 ) ) ;
#67419=CARTESIAN_POINT ( 'NONE',  ( 14.04375000122903216, -2.886751345948181946, -4.999999999999904077 ) ) ;
#67421=CARTESIAN_POINT ( 'NONE',  ( 21.83437500061451786, -2.746126346562641984, -4.756430356249999214 ) ) ;
#67433=CARTESIAN_POINT ( 'NONE',  ( 13.77187500061451431, 5.824947211148865298E-16, -4.756430356249998326 ) ) ;
#67437=( BOUNDED_CURVE ( )  B_SPLINE_CURVE ( 2, ( #30163, #34610, #57862, #2102, #69692, #12803, #52696 ),
 .UNSPECIFIED., .F., .F. ) 
 B_SPLINE_CURVE_WITH_KNOTS ( ( 3, 2, 2, 3 ),
 ( 0.8000000000000000444, 0.8033333333333333437, 0.8066666666666666430, 0.8100000000000000533 ),
 .UNSPECIFIED. ) 
 CURVE ( )  GEOMETRIC_REPRESENTATION_ITEM ( )  RATIONAL_B_SPLINE_CURVE ( ( 1.000000000000000000, 0.8660254037844387076, 1.000000000000000000, 0.8660254037844387076, 1.000000000000000000, 0.8660254037844387076, 1.000000000000000000 ) ) 
 REPRESENTATION_ITEM ( '' )  );
#67457=CARTESIAN_POINT ( 'NONE',  ( 15.75937500061451857, 4.119189519843966529, -2.378215178124998275 ) ) ;
#67468=CARTESIAN_POINT ( 'NONE',  ( 11.68125000122903145, -4.330127018922194537, 2.499999999999995559 ) ) ;
#67475=CARTESIAN_POINT ( 'NONE',  ( 25.48125000122903216, 4.330127018922191873, 2.499999999999999556 ) ) ;
#67498=DIRECTION ( 'NONE',  ( 0.000000000000000000, 0.000000000000000000, 1.000000000000000000 ) ) ;
#67504=CARTESIAN_POINT ( 'NONE',  ( 26.19375000122903074, -2.886751345948126435, -5.000000000000000000 ) ) ;
#67519=CARTESIAN_POINT ( 'NONE',  ( 18.87187500061451573, 4.119189519843966529, 2.378215178124999607 ) ) ;
#67527=EDGE_CURVE ( 'NONE', #675, #38481, #22666, .T. ) ;
#67536=CARTESIAN_POINT ( 'NONE',  ( 22.65937500061451715, 0.000000000000000000, 4.756430356249998326 ) ) ;
#67546=DIRECTION ( 'NONE',  ( -1.000000000000000000, -0.000000000000000000, -0.000000000000000000 ) ) ;
#67553=CARTESIAN_POINT ( 'NONE',  ( 18.33749999999999858, -2.886751345948130876, 4.999999999999996447 ) ) ;
#67576=ORIENTED_EDGE ( 'NONE', *, *, #48137, .F. ) ;
#67579=CARTESIAN_POINT ( 'NONE',  ( 17.32499999999999929, 4.330127018922191873, 2.499999999999999556 ) ) ;
#67580=CARTESIAN_POINT ( 'NONE',  ( 10.99687500061451750, -2.746126346562646425, 4.756430356249996549 ) ) ;
#67581=CARTESIAN_POINT ( 'NONE',  ( 45.00000000000000000, 0.000000000000000000, 0.000000000000000000 ) ) ;
#67592=CARTESIAN_POINT ( 'NONE',  ( 12.69375000122903430, -2.886751345948126435, -5.000000000000000000 ) ) ;
#67600=CARTESIAN_POINT ( 'NONE',  ( 17.37187500061451573, 5.824947211148865298E-16, -4.756430356249998326 ) ) ;
#67603=CARTESIAN_POINT ( 'NONE',  ( 15.09375000122903110, 5.773502691896255534, 3.535250795749688894E-16 ) ) ;
#67609=CARTESIAN_POINT ( 'NONE',  ( 21.11250000000000071, -5.773502691896255534, -1.060575238724906372E-15 ) ) ;
#67616=CARTESIAN_POINT ( 'NONE',  ( 29.52187500061451431, -5.492252693125287522, -1.008910452111647106E-15 ) ) ;
#67624=CARTESIAN_POINT ( 'NONE',  ( 11.30625000122903501, -4.330127018922190985, -2.500000000000001332 ) ) ;
#67626=ORIENTED_EDGE ( 'NONE', *, *, #51739, .F. ) ;
#67638=CARTESIAN_POINT ( 'NONE',  ( 13.80937500061451750, -4.119189519843965641, -2.378215178125001383 ) ) ;
#67652=ORIENTED_EDGE ( 'NONE', *, *, #13859, .T. ) ;
#67669=CARTESIAN_POINT ( 'NONE',  ( 18.83437500061451431, 5.824947211148865298E-16, -4.756430356249998326 ) ) ;
#67674=CARTESIAN_POINT ( 'NONE',  ( 20.28750000000000142, -2.886751345948125991, -5.000000000000000000 ) ) ;
#67677=LINE ( 'NONE', #40319, #35927 ) ;
#67678=CARTESIAN_POINT ( 'NONE',  ( 26.70937500061451075, -5.492252693125287522, -1.008910452111647106E-15 ) ) ;
#67685=CARTESIAN_POINT ( 'NONE',  ( 28.32187500061451502, 4.119189519843966529, 2.378215178124999607 ) ) ;
#67687=CARTESIAN_POINT ( 'NONE',  ( 11.25937500061451679, 2.746126346562643317, 4.756430356249998326 ) ) ;
#67690=ORIENTED_EDGE ( 'NONE', *, *, #63077, .F. ) ;
#67710=ORIENTED_EDGE ( 'NONE', *, *, #16678, .T. ) ;
#67720=CARTESIAN_POINT ( 'NONE',  ( 21.75937500061451502, 0.000000000000000000, 4.756430356249998326 ) ) ;
#67722=CARTESIAN_POINT ( 'NONE',  ( 24.88125000122903074, 6.123233995736764310E-16, -4.999999999999998224 ) ) ;
#67730=CARTESIAN_POINT ( 'NONE',  ( 17.23125000122903572, 6.123233995736764310E-16, -4.999999999999998224 ) ) ;
#67732=AXIS2_PLACEMENT_3D ( 'NONE', #62659, #10609, #67498 ) ;
#67740=CARTESIAN_POINT ( 'NONE',  ( 15.65625000122903465, 0.000000000000000000, 4.999999999999998224 ) ) ;
#67750=CARTESIAN_POINT ( 'NONE',  ( 10.76250000000000107, -5.773502691896255534, -1.060575238724906372E-15 ) ) ;
#67756=CARTESIAN_POINT ( 'NONE',  ( 26.85937500061451644, -4.119189519843965641, -2.378215178125001383 ) ) ;
#67761=CARTESIAN_POINT ( 'NONE',  ( 27.03750000000000142, -2.886751345948125991, -5.000000000000000000 ) ) ;
#67767=ADVANCED_FACE ( 'NONE', ( #8221 ), #64730, .T. ) ;
#67770=CARTESIAN_POINT ( 'NONE',  ( 10.63125000122903252, 4.330127018922191873, 2.499999999999999556 ) ) ;
#67774=CARTESIAN_POINT ( 'NONE',  ( 21.90937500061451715, 2.746126346562645981, -4.756430356249997438 ) ) ;
#67786=CARTESIAN_POINT ( 'NONE',  ( 12.27187500061451608, -4.119189519843968306, 2.378215178124996054 ) ) ;
#67787=ORIENTED_EDGE ( 'NONE', *, *, #5869, .F. ) ;
#67792=ORIENTED_EDGE ( 'NONE', *, *, #44624, .T. ) ;
#67793=CARTESIAN_POINT ( 'NONE',  ( 45.00000000000000000, 0.000000000000000000, 4.999999999999998224 ) ) ;
#67801=VERTEX_POINT ( 'NONE', #14116 ) ;
#67810=CARTESIAN_POINT ( 'NONE',  ( 29.10937500061452354, 2.746126346562645981, -4.756430356249997438 ) ) ;
#67811=CARTESIAN_POINT ( 'NONE',  ( 11.78437500061451892, 4.119189519843966529, 2.378215178124999607 ) ) ;
#67814=( BOUNDED_CURVE ( )  B_SPLINE_CURVE ( 2, ( #20860, #3525, #37494, #31591, #37856, #26046, #71112 ),
 .UNSPECIFIED., .F., .F. ) 
 B_SPLINE_CURVE_WITH_KNOTS ( ( 3, 2, 2, 3 ),
 ( 0.3300000000000000711, 0.3333333333333333703, 0.3366666666666667251, 0.3400000000000000799 ),
 .UNSPECIFIED. ) 
 CURVE ( )  GEOMETRIC_REPRESENTATION_ITEM ( )  RATIONAL_B_SPLINE_CURVE ( ( 0.9999999999999977796, 0.8660254037844409281, 1.000000000000000000, 0.8660254037844387076, 1.000000000000000000, 0.8660254037844364872, 1.000000000000002220 ) ) 
 REPRESENTATION_ITEM ( '' )  );
#67829=CARTESIAN_POINT ( 'NONE',  ( 23.08125000122903359, 6.123233995736764310E-16, -4.999999999999998224 ) ) ;
#67871=ORIENTED_EDGE ( 'NONE', *, *, #5151, .T. ) ;
#67874=ORIENTED_EDGE ( 'NONE', *, *, #27421, .F. ) ;
#67877=CARTESIAN_POINT ( 'NONE',  ( 19.95937500061451786, -5.492252693125287522, -1.008910452111647106E-15 ) ) ;
#67893=CARTESIAN_POINT ( 'NONE',  ( 20.97187500061451715, -5.492252693125287522, -1.008910452111647106E-15 ) ) ;
#67896=FACE_OUTER_BOUND ( 'NONE', #28902, .T. ) ;
#67904=CARTESIAN_POINT ( 'NONE',  ( 45.00000000000000000, 0.000000000000000000, 0.000000000000000000 ) ) ;
#67917=CARTESIAN_POINT ( 'NONE',  ( 8.371875000614515727, -5.492252693125287522, -1.008910452111647106E-15 ) ) ;
#67927=ORIENTED_EDGE ( 'NONE', *, *, #8491, .T. ) ;
#67937=AXIS2_PLACEMENT_3D ( 'NONE', #69721, #40935, #58982 ) ;
#67938=CARTESIAN_POINT ( 'NONE',  ( 9.121875000614517504, 2.746126346562643317, 4.756430356249998326 ) ) ;
#67950=VECTOR ( 'NONE', #19039, 1000.000000000000000 ) ;
#67951=CARTESIAN_POINT ( 'NONE',  ( 9.562500000000001776, 2.886751345948129099, -4.999999999999997335 ) ) ;
#67959=CARTESIAN_POINT ( 'NONE',  ( 18.79687500061451289, 4.119189519843966529, -2.378215178124998275 ) ) ;
#67962=CARTESIAN_POINT ( 'NONE',  ( 25.32187500061451502, -4.119189519843968306, 2.378215178124996054 ) ) ;
#67976=CARTESIAN_POINT ( 'NONE',  ( 28.65937500061451715, -4.119189519843965641, -2.378215178125001383 ) ) ;
#67982=CARTESIAN_POINT ( 'NONE',  ( 14.47499999999999964, 6.123233995736764310E-16, -4.999999999999998224 ) ) ;
#67997=CARTESIAN_POINT ( 'NONE',  ( 14.74687500061451750, -2.746126346562641984, -4.756430356249999214 ) ) ;
#68029=AXIS2_PLACEMENT_3D ( 'NONE', #26181, #64969, #37990 ) ;
#68030=CARTESIAN_POINT ( 'NONE',  ( 16.05937500061451573, -4.119189519843965641, -2.378215178125001383 ) ) ;
#68037=CARTESIAN_POINT ( 'NONE',  ( 20.06250000000000000, 2.886751345948126879, 4.999999999999999112 ) ) ;
#68041=CARTESIAN_POINT ( 'NONE',  ( 25.58437500061451431, 5.492252693125287522, 3.363034840372157021E-16 ) ) ;
#68049=CARTESIAN_POINT ( 'NONE',  ( 25.24687500061451217, 0.000000000000000000, 4.756430356249998326 ) ) ;
#68051=CARTESIAN_POINT ( 'NONE',  ( 11.78437500061451537, -2.746126346562646425, 4.756430356249996549 ) ) ;
#68056=CARTESIAN_POINT ( 'NONE',  ( 8.156250001229034652, -4.330127018922190985, -2.500000000000001332 ) ) ;
#68058=( BOUNDED_CURVE ( )  B_SPLINE_CURVE ( 2, ( #39870, #45401, #28405, #62745, #57560, #29135, #7323 ),
 .UNSPECIFIED., .F., .F. ) 
 B_SPLINE_CURVE_WITH_KNOTS ( ( 3, 2, 2, 3 ),
 ( 0.5200000000000000178, 0.5233333333333333171, 0.5266666666666666163, 0.5300000000000000266 ),
 .UNSPECIFIED. ) 
 CURVE ( )  GEOMETRIC_REPRESENTATION_ITEM ( )  RATIONAL_B_SPLINE_CURVE ( ( 1.000000000000000000, 0.8660254037844387076, 1.000000000000000000, 0.8660254037844387076, 1.000000000000000000, 0.8660254037844387076, 1.000000000000000000 ) ) 
 REPRESENTATION_ITEM ( '' )  );
#68061=CARTESIAN_POINT ( 'NONE',  ( 12.31875000122903430, 2.886751345948073588, -5.000000000000094147 ) ) ;
#68062=ORIENTED_EDGE ( 'NONE', *, *, #57008, .F. ) ;
#68064=CARTESIAN_POINT ( 'NONE',  ( 14.40937500061451537, 2.746126346562643317, 4.756430356249998326 ) ) ;
#68074=CARTESIAN_POINT ( 'NONE',  ( 18.78749999999999432, -2.886751345948074920, 5.000000000000092371 ) ) ;
#68084=VECTOR ( 'NONE', #17283, 1000.000000000000000 ) ;
#68086=CARTESIAN_POINT ( 'NONE',  ( 20.74687500061452283, 5.492252693125287522, 3.363034840372157021E-16 ) ) ;
#68106=CARTESIAN_POINT ( 'NONE',  ( 15.61875000122903323, 2.886751345948126879, 4.999999999999999112 ) ) ;
#68116=ADVANCED_FACE ( 'NONE', ( #64364 ), #54029, .T. ) ;
#68123=CARTESIAN_POINT ( 'NONE',  ( 25.02187500061451431, -5.492252693125287522, -1.008910452111647106E-15 ) ) ;
#68128=CARTESIAN_POINT ( 'NONE',  ( 27.59999999999999787, 4.330127018922192761, -2.499999999999997780 ) ) ;
#68138=CARTESIAN_POINT ( 'NONE',  ( 9.956250001229033586, -4.330127018922190985, -2.500000000000001332 ) ) ;
#68142=CARTESIAN_POINT ( 'NONE',  ( 18.42187500061451644, 4.119189519843966529, 2.378215178124999607 ) ) ;
#68154=CARTESIAN_POINT ( 'NONE',  ( 12.90937500061451537, 2.746126346562645981, -4.756430356249997438 ) ) ;
#68160=VERTEX_POINT ( 'NONE', #37753 ) ;
#68174=CARTESIAN_POINT ( 'NONE',  ( 27.98437500061451289, 4.119189519843966529, 2.378215178124999607 ) ) ;
#68177=CARTESIAN_POINT ( 'NONE',  ( 22.44375000122903785, -2.886751345948157965, 4.999999999999948486 ) ) ;
#68179=CARTESIAN_POINT ( 'NONE',  ( 11.89687500061451608, -2.746126346562646425, 4.756430356249996549 ) ) ;
#68187=CARTESIAN_POINT ( 'NONE',  ( 11.71875000122903465, -5.773502691896255534, -1.060575238724906372E-15 ) ) ;
#68190=DIRECTION ( 'NONE',  ( 0.000000000000000000, 0.000000000000000000, 1.000000000000000000 ) ) ;
#68195=CARTESIAN_POINT ( 'NONE',  ( 23.34375000122903288, -2.886751345948129988, 4.999999999999997335 ) ) ;
#68205=CARTESIAN_POINT ( 'NONE',  ( 29.06249999999999289, 2.886751345948161962, 4.999999999999938716 ) ) ;
#68220=CARTESIAN_POINT ( 'NONE',  ( 15.65625000122903465, 0.000000000000000000, 4.999999999999998224 ) ) ;
#68243=CARTESIAN_POINT ( 'NONE',  ( 17.82187500061451502, 5.824947211148865298E-16, -4.756430356249998326 ) ) ;
#68259=DIRECTION ( 'NONE',  ( -1.000000000000000000, -0.000000000000000000, -0.000000000000000000 ) ) ;
#68260=CARTESIAN_POINT ( 'NONE',  ( 19.77187500061451786, 2.746126346562645981, -4.756430356249997438 ) ) ;
#68263=CARTESIAN_POINT ( 'NONE',  ( 28.36875000122903145, -5.773502691896255534, -1.060575238724906372E-15 ) ) ;
#68282=CARTESIAN_POINT ( 'NONE',  ( 7.546875000614515550, -2.746126346562641984, -4.756430356249999214 ) ) ;
#68302=CARTESIAN_POINT ( 'NONE',  ( 11.55000000000000071, 0.000000000000000000, 4.999999999999998224 ) ) ;
#68304=CARTESIAN_POINT ( 'NONE',  ( 8.371875000614515727, -5.492252693125287522, -1.008910452111647106E-15 ) ) ;
#68322=FACE_OUTER_BOUND ( 'NONE', #22895, .T. ) ;
#68324=CARTESIAN_POINT ( 'NONE',  ( 18.72187500061451360, 5.824947211148865298E-16, -4.756430356249998326 ) ) ;
#68327=CARTESIAN_POINT ( 'NONE',  ( 26.22187500061451360, -4.119189519843968306, 2.378215178124996054 ) ) ;
#68341=CARTESIAN_POINT ( 'NONE',  ( 26.70937500061451431, 0.000000000000000000, 4.756430356249998326 ) ) ;
#68359=CARTESIAN_POINT ( 'NONE',  ( 15.38437500061451679, 4.119189519843966529, 2.378215178124999607 ) ) ;
#68363=VERTEX_POINT ( 'NONE', #3189 ) ;
#68389=CARTESIAN_POINT ( 'NONE',  ( 17.52187500061451431, 2.746126346562645981, -4.756430356249997438 ) ) ;
#68395=CARTESIAN_POINT ( 'NONE',  ( 17.51249999999999929, -5.773502691896255534, -1.060575238724906372E-15 ) ) ;
#68399=CARTESIAN_POINT ( 'NONE',  ( 26.55937500061451573, 2.746126346562643317, 4.756430356249998326 ) ) ;
#68402=FACE_OUTER_BOUND ( 'NONE', #66802, .T. ) ;
#68406=CARTESIAN_POINT ( 'NONE',  ( 26.03437500061451360, 5.492252693125287522, 3.363034840372157021E-16 ) ) ;
#68408=CARTESIAN_POINT ( 'NONE',  ( 10.69687500061451679, 4.119189519843966529, -2.378215178124998275 ) ) ;
#68411=ORIENTED_EDGE ( 'NONE', *, *, #53665, .T. ) ;
#68413=DIRECTION ( 'NONE',  ( -1.000000000000000000, -0.000000000000000000, -0.000000000000000000 ) ) ;
#68420=CARTESIAN_POINT ( 'NONE',  ( 11.29687500061451644, 0.000000000000000000, 4.756430356249998326 ) ) ;
#68439=CARTESIAN_POINT ( 'NONE',  ( 22.73437500061451644, -4.119189519843968306, 2.378215178124996054 ) ) ;
#68460=CARTESIAN_POINT ( 'NONE',  ( 16.18125000122903145, -4.330127018922194537, 2.499999999999995559 ) ) ;
#68462=LINE ( 'NONE', #24468, #56173 ) ;
#68476=CARTESIAN_POINT ( 'NONE',  ( 24.27187500061452141, 2.746126346562645981, -4.756430356249997438 ) ) ;
#68481=CARTESIAN_POINT ( 'NONE',  ( 23.66250000000000142, 2.886751345948126879, 4.999999999999999112 ) ) ;
#68485=( BOUNDED_CURVE ( )  B_SPLINE_CURVE ( 2, ( #72875, #51064, #45531, #27816, #10451, #17068, #56950 ),
 .UNSPECIFIED., .F., .F. ) 
 B_SPLINE_CURVE_WITH_KNOTS ( ( 3, 2, 2, 3 ),
 ( 0.5100000000000000089, 0.5133333333333333082, 0.5166666666666667185, 0.5200000000000000178 ),
 .UNSPECIFIED. ) 
 CURVE ( )  GEOMETRIC_REPRESENTATION_ITEM ( )  RATIONAL_B_SPLINE_CURVE ( ( 1.000000000000000000, 0.8660254037844387076, 1.000000000000000000, 0.8660254037844387076, 1.000000000000000000, 0.8660254037844387076, 1.000000000000000000 ) ) 
 REPRESENTATION_ITEM ( '' )  );
#68492=CARTESIAN_POINT ( 'NONE',  ( 10.33125000122903359, -4.330127018922194537, 2.499999999999995559 ) ) ;
#68496=CARTESIAN_POINT ( 'NONE',  ( 17.82187500061451502, 5.824947211148865298E-16, -4.756430356249998326 ) ) ;
#68503=EDGE_CURVE ( 'NONE', #41603, #44765, #59683, .T. ) ;
#68508=CARTESIAN_POINT ( 'NONE',  ( 11.18437500061451573, 5.492252693125287522, 3.363034840372157021E-16 ) ) ;
#68516=VERTEX_POINT ( 'NONE', #42707 ) ;
#68523=CARTESIAN_POINT ( 'NONE',  ( 10.27499999999999858, -4.330127018922194537, 2.499999999999995559 ) ) ;
#68532=CARTESIAN_POINT ( 'NONE',  ( 28.43437500061451573, 4.119189519843966529, 2.378215178124999607 ) ) ;
#68535=CARTESIAN_POINT ( 'NONE',  ( 28.80937500061451217, 2.746126346562643317, 4.756430356249998326 ) ) ;
#68536=CARTESIAN_POINT ( 'NONE',  ( 12.79687500061451821, -2.746126346562646425, 4.756430356249996549 ) ) ;
#68545=CARTESIAN_POINT ( 'NONE',  ( 11.79375000122903039, -2.886751345948181946, -4.999999999999904077 ) ) ;
#68546=( BOUNDED_CURVE ( )  B_SPLINE_CURVE ( 2, ( #19736, #48196, #32665, #37473, #65175, #43391, #15295 ),
 .UNSPECIFIED., .F., .F. ) 
 B_SPLINE_CURVE_WITH_KNOTS ( ( 3, 2, 2, 3 ),
 ( 0.3599999999999999867, 0.3633333333333333415, 0.3666666666666666408, 0.3699999999999999956 ),
 .UNSPECIFIED. ) 
 CURVE ( )  GEOMETRIC_REPRESENTATION_ITEM ( )  RATIONAL_B_SPLINE_CURVE ( ( 1.000000000000000000, 0.8660254037844387076, 1.000000000000000000, 0.8660254037844387076, 1.000000000000000000, 0.8660254037844387076, 1.000000000000000000 ) ) 
 REPRESENTATION_ITEM ( '' )  );
#68554=CARTESIAN_POINT ( 'NONE',  ( 24.05625000122903145, 4.330127018922192761, -2.499999999999997780 ) ) ;
#68592=CARTESIAN_POINT ( 'NONE',  ( 11.13750000000000107, -2.886751345948130876, 4.999999999999996447 ) ) ;
#68594=ORIENTED_EDGE ( 'NONE', *, *, #15556, .T. ) ;
#68602=CARTESIAN_POINT ( 'NONE',  ( 19.47187500061451360, -4.119189519843968306, 2.378215178124996054 ) ) ;
#68620=CARTESIAN_POINT ( 'NONE',  ( 20.33437500061451786, 4.119189519843966529, 2.378215178124999607 ) ) ;
#68631=CARTESIAN_POINT ( 'NONE',  ( 45.00000000000000000, 0.000000000000000000, 0.000000000000000000 ) ) ;
#68638=DIRECTION ( 'NONE',  ( -1.000000000000000000, -0.000000000000000000, -0.000000000000000000 ) ) ;
#68642=CYLINDRICAL_SURFACE ( 'NONE', #57514, 4.999999999999998224 ) ;
#68665=CARTESIAN_POINT ( 'NONE',  ( 8.559375000614515727, 4.119189519843966529, -2.378215178124998275 ) ) ;
#68671=( BOUNDED_CURVE ( )  B_SPLINE_CURVE ( 2, ( #28417, #5528, #11063, #33589, #56842, #16236, #11792 ),
 .UNSPECIFIED., .F., .F. ) 
 B_SPLINE_CURVE_WITH_KNOTS ( ( 3, 2, 2, 3 ),
 ( 0.7900000000000001465, 0.7933333333333334458, 0.7966666666666666341, 0.8000000000000000444 ),
 .UNSPECIFIED. ) 
 CURVE ( )  GEOMETRIC_REPRESENTATION_ITEM ( )  RATIONAL_B_SPLINE_CURVE ( ( 0.9999999999999955591, 0.8660254037844431485, 1.000000000000000000, 0.8660254037844387076, 1.000000000000000000, 0.8660254037844387076, 1.000000000000000000 ) ) 
 REPRESENTATION_ITEM ( '' )  );
#68685=ADVANCED_FACE ( 'NONE', ( #72612 ), #72246, .T. ) ;
#68687=CARTESIAN_POINT ( 'NONE',  ( 18.83437500061451786, 5.492252693125287522, 3.363034840372157021E-16 ) ) ;
#68690=CARTESIAN_POINT ( 'NONE',  ( 25.80937500061451217, -5.492252693125287522, -1.008910452111647106E-15 ) ) ;
#68698=CARTESIAN_POINT ( 'NONE',  ( 27.80625000122903145, 0.000000000000000000, 4.999999999999998224 ) ) ;
#68704=CARTESIAN_POINT ( 'NONE',  ( 26.48437500061451644, 5.824947211148865298E-16, -4.756430356249998326 ) ) ;
#68710=DIRECTION ( 'NONE',  ( -1.000000000000000000, -0.000000000000000000, -0.000000000000000000 ) ) ;
#68722=CARTESIAN_POINT ( 'NONE',  ( 14.63437500061451679, -4.119189519843968306, 2.378215178124996054 ) ) ;
#68729=( BOUNDED_CURVE ( )  B_SPLINE_CURVE ( 2, ( #4897, #38512, #54769, #49237, #72126, #3808, #66215 ),
 .UNSPECIFIED., .F., .F. ) 
 B_SPLINE_CURVE_WITH_KNOTS ( ( 3, 2, 2, 3 ),
 ( 0.07000000000000000666, 0.07333333333333333370, 0.07666666666666664687, 0.07999999999999998779 ),
 .UNSPECIFIED. ) 
 CURVE ( )  GEOMETRIC_REPRESENTATION_ITEM ( )  RATIONAL_B_SPLINE_CURVE ( ( 1.000000000000000000, 0.8660254037844387076, 1.000000000000000000, 0.8660254037844387076, 1.000000000000000000, 0.8660254037844392627, 0.9999999999999994449 ) ) 
 REPRESENTATION_ITEM ( '' )  );
#68731=AXIS2_PLACEMENT_3D ( 'NONE', #4998, #27169, #44892 ) ;
#68736=CARTESIAN_POINT ( 'NONE',  ( 22.01249999999999574, -5.773502691896255534, -1.060575238724906372E-15 ) ) ;
#68753=CARTESIAN_POINT ( 'NONE',  ( 16.35937500061451644, 0.000000000000000000, 4.756430356249998326 ) ) ;
#68760=CARTESIAN_POINT ( 'NONE',  ( 17.36249999999999716, 2.886751345948126879, 4.999999999999999112 ) ) ;
#68763=LINE ( 'NONE', #1531, #56039 ) ;
#68764=CARTESIAN_POINT ( 'NONE',  ( 23.55937500061451573, -5.492252693125287522, -1.008910452111647106E-15 ) ) ;
#68772=CARTESIAN_POINT ( 'NONE',  ( 25.35937500061451644, -5.492252693125287522, -1.008910452111647106E-15 ) ) ;
#68774=CARTESIAN_POINT ( 'NONE',  ( 11.44687500061451679, -4.119189519843965641, -2.378215178125001383 ) ) ;
#68779=DIRECTION ( 'NONE',  ( -1.000000000000000000, -0.000000000000000000, -0.000000000000000000 ) ) ;
#68783=CARTESIAN_POINT ( 'NONE',  ( 12.43125000122903145, 4.330127018922191873, 2.499999999999999556 ) ) ;
#68784=ORIENTED_EDGE ( 'NONE', *, *, #30682, .T. ) ;
#68786=CARTESIAN_POINT ( 'NONE',  ( 11.44687500061451679, -4.119189519843965641, -2.378215178125001383 ) ) ;
#68789=EDGE_CURVE ( 'NONE', #26491, #69693, #21184, .T. ) ;
#68806=CARTESIAN_POINT ( 'NONE',  ( 21.98437500061451644, 5.824947211148865298E-16, -4.756430356249998326 ) ) ;
#68826=CARTESIAN_POINT ( 'NONE',  ( 16.40625000122903643, 4.330127018922192761, -2.499999999999997780 ) ) ;
#68828=CARTESIAN_POINT ( 'NONE',  ( 9.299999999999998934, 0.000000000000000000, 4.999999999999998224 ) ) ;
#68837=ORIENTED_EDGE ( 'NONE', *, *, #39594, .F. ) ;
#68841=CARTESIAN_POINT ( 'NONE',  ( 23.18437500061451573, -4.119189519843968306, 2.378215178124996054 ) ) ;
#68846=CARTESIAN_POINT ( 'NONE',  ( 25.76249999999999929, 2.886751345948129099, -4.999999999999998224 ) ) ;
#68850=CARTESIAN_POINT ( 'NONE',  ( 12.95625000122903359, 0.000000000000000000, 4.999999999999998224 ) ) ;
#68854=CARTESIAN_POINT ( 'NONE',  ( 15.37500000000000000, 6.123233995736764310E-16, -4.999999999999998224 ) ) ;
#68856=CARTESIAN_POINT ( 'NONE',  ( 8.681250001229031454, 6.123233995736764310E-16, -4.999999999999998224 ) ) ;
#68859=CARTESIAN_POINT ( 'NONE',  ( 19.09687500061451360, -4.119189519843965641, -2.378215178125001383 ) ) ;
#68870=CARTESIAN_POINT ( 'NONE',  ( 11.07187500061451679, 5.824947211148865298E-16, -4.756430356249998326 ) ) ;
#68883=CARTESIAN_POINT ( 'NONE',  ( 9.525000000000002132, 6.123233995736764310E-16, -4.999999999999998224 ) ) ;
#68892=CARTESIAN_POINT ( 'NONE',  ( 29.33437500061451431, 4.119189519843966529, 2.378215178124999607 ) ) ;
#68894=CARTESIAN_POINT ( 'NONE',  ( 28.69687500061451502, 4.119189519843966529, -2.378215178124998275 ) ) ;
#68895=CARTESIAN_POINT ( 'NONE',  ( 13.17187500061451999, 2.746126346562643317, 4.756430356249998326 ) ) ;
#68911=CARTESIAN_POINT ( 'NONE',  ( 22.89375000122903359, -2.886751345948129988, 4.999999999999997335 ) ) ;
#68932=( BOUNDED_CURVE ( )  B_SPLINE_CURVE ( 2, ( #67344, #38529, #44811, #16705, #11178, #33702, #44076 ),
 .UNSPECIFIED., .F., .F. ) 
 B_SPLINE_CURVE_WITH_KNOTS ( ( 3, 2, 2, 3 ),
 ( 0.3900000000000000133, 0.3933333333333333126, 0.3966666666666667229, 0.4000000000000000777 ),
 .UNSPECIFIED. ) 
 CURVE ( )  GEOMETRIC_REPRESENTATION_ITEM ( )  RATIONAL_B_SPLINE_CURVE ( ( 1.000000000000000000, 0.8660254037844387076, 1.000000000000000000, 0.8660254037844387076, 1.000000000000000000, 0.8660254037844364872, 1.000000000000002220 ) ) 
 REPRESENTATION_ITEM ( '' )  );
#68938=CYLINDRICAL_SURFACE ( 'NONE', #25304, 4.999999999999998224 ) ;
#68947=CARTESIAN_POINT ( 'NONE',  ( 7.800000000000001599, 4.330127018922192761, -2.499999999999997780 ) ) ;
#68962=ORIENTED_EDGE ( 'NONE', *, *, #21957, .T. ) ;
#68965=CARTESIAN_POINT ( 'NONE',  ( 19.69687500061451502, 4.119189519843966529, -2.378215178124998275 ) ) ;
#68967=( BOUNDED_CURVE ( )  B_SPLINE_CURVE ( 2, ( #4960, #56295, #50394, #22659, #55206, #62548, #72191 ),
 .UNSPECIFIED., .F., .F. ) 
 B_SPLINE_CURVE_WITH_KNOTS ( ( 3, 2, 2, 3 ),
 ( 0.000000000000000000, 0.003333333333333326608, 0.006666666666666653217, 0.009999999999999979391 ),
 .UNSPECIFIED. ) 
 CURVE ( )  GEOMETRIC_REPRESENTATION_ITEM ( )  RATIONAL_B_SPLINE_CURVE ( ( 1.000000000000000000, 0.8660254037844387076, 1.000000000000000000, 0.8660254037844387076, 1.000000000000000000, 0.8660254037844395958, 0.9999999999999991118 ) ) 
 REPRESENTATION_ITEM ( '' )  );
#68983=CARTESIAN_POINT ( 'NONE',  ( 20.74687500061451573, 5.492252693125287522, 3.363034840372157021E-16 ) ) ;
#69010=AXIS2_PLACEMENT_3D ( 'NONE', #53428, #37160, #48621 ) ;
#69012=FACE_OUTER_BOUND ( 'NONE', #42711, .T. ) ;
#69023=ADVANCED_FACE ( 'NONE', ( #8154 ), #19952, .T. ) ;
#69028=CARTESIAN_POINT ( 'NONE',  ( 8.071875000614518569, 2.746126346562645981, -4.756430356249997438 ) ) ;
#69037=CARTESIAN_POINT ( 'NONE',  ( 45.00000000000000000, 0.000000000000000000, 0.000000000000000000 ) ) ;
#69048=CARTESIAN_POINT ( 'NONE',  ( 16.54687500061451644, 4.119189519843966529, -2.378215178124998275 ) ) ;
#69051=CARTESIAN_POINT ( 'NONE',  ( 26.07187500061451146, 4.119189519843966529, 2.378215178124999607 ) ) ;
#69069=CARTESIAN_POINT ( 'NONE',  ( 26.85937500061451644, -4.119189519843965641, -2.378215178125001383 ) ) ;
#69087=CARTESIAN_POINT ( 'NONE',  ( 15.45937500061451608, 0.000000000000000000, 4.756430356249998326 ) ) ;
#69101=EDGE_LOOP ( 'NONE', ( #41383, #8548, #72964, #53551 ) ) ;
#69108=AXIS2_PLACEMENT_3D ( 'NONE', #38448, #60974, #10374 ) ;
#69119=VECTOR ( 'NONE', #12272, 1000.000000000000000 ) ;
#69121=CARTESIAN_POINT ( 'NONE',  ( 15.30937500061451750, 4.119189519843966529, -2.378215178124998275 ) ) ;
#69127=CARTESIAN_POINT ( 'NONE',  ( 17.32499999999999929, 4.330127018922191873, 2.499999999999999556 ) ) ;
#69131=CARTESIAN_POINT ( 'NONE',  ( 22.84687500061451360, 4.119189519843966529, -2.378215178124998275 ) ) ;
#69132=ORIENTED_EDGE ( 'NONE', *, *, #4558, .F. ) ;
#69134=CARTESIAN_POINT ( 'NONE',  ( 26.58749999999999858, -2.886751345948126435, -5.000000000000000000 ) ) ;
#69138=CARTESIAN_POINT ( 'NONE',  ( 25.73437500061451644, -2.746126346562646425, 4.756430356249996549 ) ) ;
#69140=CARTESIAN_POINT ( 'NONE',  ( 10.17187500061451644, 5.824947211148865298E-16, -4.756430356249998326 ) ) ;
#69143=ORIENTED_EDGE ( 'NONE', *, *, #5554, .T. ) ;
#69145=CARTESIAN_POINT ( 'NONE',  ( 16.68750000000000000, -2.886751345948126435, -5.000000000000000000 ) ) ;
#69148=CARTESIAN_POINT ( 'NONE',  ( 26.41875000122903216, 2.886751345948126879, 4.999999999999998224 ) ) ;
#69149=DIRECTION ( 'NONE',  ( -1.000000000000000000, -0.000000000000000000, -0.000000000000000000 ) ) ;
#69152=CARTESIAN_POINT ( 'NONE',  ( 12.83437500061451786, -2.746126346562642428, -4.756430356249999214 ) ) ;
#69157=( BOUNDED_CURVE ( )  B_SPLINE_CURVE ( 2, ( #23609, #24694, #63851, #58670, #736, #17691, #34693 ),
 .UNSPECIFIED., .F., .F. ) 
 B_SPLINE_CURVE_WITH_KNOTS ( ( 3, 2, 2, 3 ),
 ( 0.05000000000000005135, 0.05333333333333338533, 0.05666666666666670543, 0.06000000000000003941 ),
 .UNSPECIFIED. ) 
 CURVE ( )  GEOMETRIC_REPRESENTATION_ITEM ( )  RATIONAL_B_SPLINE_CURVE ( ( 0.9999999999999981126, 0.8660254037844407060, 1.000000000000000000, 0.8660254037844387076, 1.000000000000000000, 0.8660254037844370423, 1.000000000000001776 ) ) 
 REPRESENTATION_ITEM ( '' )  );
#69164=ORIENTED_EDGE ( 'NONE', *, *, #51006, .T. ) ;
#69171=CARTESIAN_POINT ( 'NONE',  ( 21.23437500061451644, 4.119189519843966529, 2.378215178124999607 ) ) ;
#69192=DIRECTION ( 'NONE',  ( -1.000000000000000000, -0.000000000000000000, -0.000000000000000000 ) ) ;
#69208=CARTESIAN_POINT ( 'NONE',  ( 22.65937500061451715, 0.000000000000000000, 4.756430356249998326 ) ) ;
#69214=CARTESIAN_POINT ( 'NONE',  ( 25.68750000000000000, -2.886751345948125991, -5.000000000000000000 ) ) ;
#69222=CARTESIAN_POINT ( 'NONE',  ( 10.10625000122903216, 4.330127018922192761, -2.499999999999997780 ) ) ;
#69223=CARTESIAN_POINT ( 'NONE',  ( 9.074999999999999289, 6.123233995736764310E-16, -4.999999999999998224 ) ) ;
#69225=CARTESIAN_POINT ( 'NONE',  ( 18.49687500061451573, 0.000000000000000000, 4.756430356249998326 ) ) ;
#69236=CARTESIAN_POINT ( 'NONE',  ( 9.946875000614516793, 0.000000000000000000, 4.756430356249998326 ) ) ;
#69242=VERTEX_POINT ( 'NONE', #56140 ) ;
#69243=CARTESIAN_POINT ( 'NONE',  ( 13.64999999999999858, 4.330127018922192761, -2.499999999999997780 ) ) ;
#69249=CARTESIAN_POINT ( 'NONE',  ( 9.937500000000001776, -2.886751345948125991, -5.000000000000000000 ) ) ;
#69257=CARTESIAN_POINT ( 'NONE',  ( 28.99687500061451573, -2.746126346562646425, 4.756430356249996549 ) ) ;
#69259=CARTESIAN_POINT ( 'NONE',  ( 27.15937500061451360, -5.492252693125287522, -1.008910452111647106E-15 ) ) ;
#69260=CARTESIAN_POINT ( 'NONE',  ( 13.39687500061451608, -2.746126346562642428, -4.756430356249999214 ) ) ;
#69266=DIRECTION ( 'NONE',  ( -1.000000000000000000, -0.000000000000000000, -0.000000000000000000 ) ) ;
#69276=CARTESIAN_POINT ( 'NONE',  ( 23.90625000122903288, -4.330127018922190985, -2.500000000000001332 ) ) ;
#69278=CARTESIAN_POINT ( 'NONE',  ( 22.61249999999999361, 2.886751345948101122, -5.000000000000046185 ) ) ;
#69284=CARTESIAN_POINT ( 'NONE',  ( 29.09999999999999787, 0.000000000000000000, 4.999999999999998224 ) ) ;
#69305=( BOUNDED_CURVE ( )  B_SPLINE_CURVE ( 2, ( #56636, #33380, #50385, #55916, #72910, #36914, #35546 ),
 .UNSPECIFIED., .F., .F. ) 
 B_SPLINE_CURVE_WITH_KNOTS ( ( 3, 2, 2, 3 ),
 ( 0.9699999999999999734, 0.9733333333333333837, 0.9766666666666666829, 0.9799999999999999822 ),
 .UNSPECIFIED. ) 
 CURVE ( )  GEOMETRIC_REPRESENTATION_ITEM ( )  RATIONAL_B_SPLINE_CURVE ( ( 1.000000000000000000, 0.8660254037844387076, 1.000000000000000000, 0.8660254037844387076, 1.000000000000000000, 0.8660254037844387076, 1.000000000000000000 ) ) 
 REPRESENTATION_ITEM ( '' )  );
#69317=CARTESIAN_POINT ( 'NONE',  ( 45.00000000000000000, 6.123233995736764310E-16, -4.999999999999998224 ) ) ;
#69324=EDGE_CURVE ( 'NONE', #24785, #44627, #9332, .T. ) ;
#69328=CARTESIAN_POINT ( 'NONE',  ( 15.60937500061451644, 2.746126346562645981, -4.756430356249997438 ) ) ;
#69337=VERTEX_POINT ( 'NONE', #28421 ) ;
#69348=CARTESIAN_POINT ( 'NONE',  ( 19.28437500061451360, 5.824947211148865298E-16, -4.756430356249998326 ) ) ;
#69361=ORIENTED_EDGE ( 'NONE', *, *, #19740, .T. ) ;
#69363=FACE_OUTER_BOUND ( 'NONE', #11770, .T. ) ;
#69367=EDGE_CURVE ( 'NONE', #59457, #31892, #61669, .T. ) ;
#69370=CARTESIAN_POINT ( 'NONE',  ( 45.00000000000000000, 0.000000000000000000, 4.999999999999998224 ) ) ;
#69373=CARTESIAN_POINT ( 'NONE',  ( 45.00000000000000000, 0.000000000000000000, 0.000000000000000000 ) ) ;
#69396=CARTESIAN_POINT ( 'NONE',  ( 9.309375000614517504, -4.119189519843965641, -2.378215178125001383 ) ) ;
#69413=CARTESIAN_POINT ( 'NONE',  ( 15.00937500061451502, -5.492252693125287522, -1.008910452111647106E-15 ) ) ;
#69416=CARTESIAN_POINT ( 'NONE',  ( 27.30937500061451217, 2.746126346562645981, -4.756430356249997438 ) ) ;
#69430=CARTESIAN_POINT ( 'NONE',  ( 28.39687500061452141, 5.492252693125287522, 3.363034840372157021E-16 ) ) ;
#69449=CARTESIAN_POINT ( 'NONE',  ( 11.18437500061451928, 5.824947211148865298E-16, -4.756430356249998326 ) ) ;
#69461=CARTESIAN_POINT ( 'NONE',  ( 22.08749999999999503, -2.886751345948181946, -4.999999999999904077 ) ) ;
#69462=ORIENTED_EDGE ( 'NONE', *, *, #21683, .F. ) ;
#69475=VERTEX_POINT ( 'NONE', #68302 ) ;
#69479=CARTESIAN_POINT ( 'NONE',  ( 15.87187500061451573, 2.746126346562643317, 4.756430356249998326 ) ) ;
#69486=CARTESIAN_POINT ( 'NONE',  ( 17.77499999999999858, 4.330127018922191873, 2.499999999999999556 ) ) ;
#69490=CARTESIAN_POINT ( 'NONE',  ( 22.62187500061451573, -4.119189519843968306, 2.378215178124996054 ) ) ;
#69497=CARTESIAN_POINT ( 'NONE',  ( 24.45937500061451786, -5.492252693125287522, -1.008910452111647106E-15 ) ) ;
#69499=CARTESIAN_POINT ( 'NONE',  ( 8.859375000614514661, 2.746126346562645981, -4.756430356249997438 ) ) ;
#69504=CARTESIAN_POINT ( 'NONE',  ( 15.43125000122903323, 6.123233995736764310E-16, -4.999999999999998224 ) ) ;
#69510=CARTESIAN_POINT ( 'NONE',  ( 12.45937500061451608, 2.746126346562645981, -4.756430356249997438 ) ) ;
#69529=CARTESIAN_POINT ( 'NONE',  ( 19.05937500061451928, 0.000000000000000000, 4.756430356249998326 ) ) ;
#69563=CARTESIAN_POINT ( 'NONE',  ( 23.70937500061451786, -4.119189519843965641, -2.378215178125001383 ) ) ;
#69569=CARTESIAN_POINT ( 'NONE',  ( 23.88749999999999929, -2.886751345948125991, -5.000000000000000000 ) ) ;
#69578=CARTESIAN_POINT ( 'NONE',  ( 8.268750001229031810, 2.886751345948129099, -4.999999999999998224 ) ) ;
#69581=CARTESIAN_POINT ( 'NONE',  ( 15.08437500061451431, -2.746126346562641984, -4.756430356249999214 ) ) ;
#69588=CARTESIAN_POINT ( 'NONE',  ( 22.12500000000000000, 6.123233995736764310E-16, -4.999999999999998224 ) ) ;
#69592=CYLINDRICAL_SURFACE ( 'NONE', #23055, 4.999999999999998224 ) ;
#69593=CARTESIAN_POINT ( 'NONE',  ( 9.346875000614517148, 4.119189519843966529, -2.378215178124998275 ) ) ;
#69600=ORIENTED_EDGE ( 'NONE', *, *, #5067, .F. ) ;
#69601=CARTESIAN_POINT ( 'NONE',  ( 45.00000000000000000, 6.123233995736764310E-16, -4.999999999999998224 ) ) ;
#69605=CARTESIAN_POINT ( 'NONE',  ( 28.99687500061451217, -4.119189519843965641, -2.378215178125001383 ) ) ;
#69608=CARTESIAN_POINT ( 'NONE',  ( 8.550000000000002487, -4.330127018922190985, -2.500000000000001332 ) ) ;
#69617=CARTESIAN_POINT ( 'NONE',  ( 26.93437500061451573, 5.492252693125287522, 3.363034840372157021E-16 ) ) ;
#69618=CARTESIAN_POINT ( 'NONE',  ( 11.25937500061451679, 4.119189519843966529, -2.378215178124998275 ) ) ;
#69632=CARTESIAN_POINT ( 'NONE',  ( 22.18125000122903145, 6.123233995736764310E-16, -4.999999999999998224 ) ) ;
#69634=LINE ( 'NONE', #18996, #31323 ) ;
#69659=DIRECTION ( 'NONE',  ( 0.000000000000000000, 0.000000000000000000, 1.000000000000000000 ) ) ;
#69664=CARTESIAN_POINT ( 'NONE',  ( 18.07499999999999929, 6.123233995736764310E-16, -4.999999999999998224 ) ) ;
#69668=EDGE_LOOP ( 'NONE', ( #54964, #9960, #71090, #14751 ) ) ;
#69673=CARTESIAN_POINT ( 'NONE',  ( 11.28749999999999432, -2.886751345948181946, -4.999999999999904077 ) ) ;
#69684=CARTESIAN_POINT ( 'NONE',  ( 17.63437500061451502, -2.746126346562646425, 4.756430356249996549 ) ) ;
#69692=CARTESIAN_POINT ( 'NONE',  ( 11.45625000122903181, 4.330127018922192761, -2.499999999999997780 ) ) ;
#69693=VERTEX_POINT ( 'NONE', #9442 ) ;
#69700=CARTESIAN_POINT ( 'NONE',  ( 45.00000000000000000, 0.000000000000000000, 4.999999999999998224 ) ) ;
#69703=CARTESIAN_POINT ( 'NONE',  ( 17.07187500061451502, 2.746126346562645981, -4.756430356249997438 ) ) ;
#69713=LINE ( 'NONE', #42370, #19446 ) ;
#69716=DIRECTION ( 'NONE',  ( 0.000000000000000000, 1.000000000000000000, -6.195440985631455317E-17 ) ) ;
#69721=CARTESIAN_POINT ( 'NONE',  ( 45.00000000000000000, 0.000000000000000000, 0.000000000000000000 ) ) ;
#69722=LINE ( 'NONE', #18728, #48090 ) ;
#69745=CARTESIAN_POINT ( 'NONE',  ( 29.13749999999999929, -2.886751345948129988, 4.999999999999997335 ) ) ;
#69751=DIRECTION ( 'NONE',  ( 0.000000000000000000, 0.000000000000000000, 1.000000000000000000 ) ) ;
#69754=CARTESIAN_POINT ( 'NONE',  ( 15.43125000122903323, 6.123233995736764310E-16, -4.999999999999998224 ) ) ;
#69764=CARTESIAN_POINT ( 'NONE',  ( 15.12187500061451573, 5.824947211148865298E-16, -4.756430356249998326 ) ) ;
#69767=CARTESIAN_POINT ( 'NONE',  ( 22.84687500061451360, 4.119189519843966529, -2.378215178124998275 ) ) ;
#69777=( BOUNDED_CURVE ( )  B_SPLINE_CURVE ( 2, ( #27446, #65495, #54422, #37785, #3822, #42966, #14885 ),
 .UNSPECIFIED., .F., .F. ) 
 B_SPLINE_CURVE_WITH_KNOTS ( ( 3, 2, 2, 3 ),
 ( 0.1699999999999999567, 0.1733333333333332837, 0.1766666666666666108, 0.1799999999999999378 ),
 .UNSPECIFIED. ) 
 CURVE ( )  GEOMETRIC_REPRESENTATION_ITEM ( )  RATIONAL_B_SPLINE_CURVE ( ( 1.000000000000002220, 0.8660254037844364872, 1.000000000000000000, 0.8660254037844387076, 1.000000000000000000, 0.8660254037844409281, 0.9999999999999977796 ) ) 
 REPRESENTATION_ITEM ( '' )  );
#69783=CARTESIAN_POINT ( 'NONE',  ( 25.73437500061451644, 4.119189519843966529, 2.378215178124999607 ) ) ;
#69786=CYLINDRICAL_SURFACE ( 'NONE', #56135, 4.999999999999998224 ) ;
#69803=CARTESIAN_POINT ( 'NONE',  ( 12.72187500061451537, 2.746126346562643317, 4.756430356249998326 ) ) ;
#69810=( BOUNDED_CURVE ( )  B_SPLINE_CURVE ( 2, ( #62070, #384, #39546, #22539, #51349, #56524, #40268 ),
 .UNSPECIFIED., .F., .F. ) 
 B_SPLINE_CURVE_WITH_KNOTS ( ( 3, 2, 2, 3 ),
 ( 0.2100000000000000477, 0.2133333333333333748, 0.2166666666666667018, 0.2200000000000000011 ),
 .UNSPECIFIED. ) 
 CURVE ( )  GEOMETRIC_REPRESENTATION_ITEM ( )  RATIONAL_B_SPLINE_CURVE ( ( 0.9999999999999977796, 0.8660254037844409281, 1.000000000000000000, 0.8660254037844387076, 1.000000000000000000, 0.8660254037844387076, 1.000000000000000000 ) ) 
 REPRESENTATION_ITEM ( '' )  );
#69830=ORIENTED_EDGE ( 'NONE', *, *, #15774, .F. ) ;
#69835=CARTESIAN_POINT ( 'NONE',  ( 14.48437500061451821, 4.119189519843966529, 2.378215178124999607 ) ) ;
#69840=CARTESIAN_POINT ( 'NONE',  ( 17.25000000000000000, 4.330127018922192761, -2.499999999999997780 ) ) ;
#69843=CARTESIAN_POINT ( 'NONE',  ( 22.24687500061451573, -4.119189519843965641, -2.378215178125001383 ) ) ;
#69851=CARTESIAN_POINT ( 'NONE',  ( 21.79687500061451644, -4.119189519843965641, -2.378215178125001383 ) ) ;
#69853=CARTESIAN_POINT ( 'NONE',  ( 9.159375000614515372, -5.492252693125287522, -1.008910452111647106E-15 ) ) ;
#69861=CARTESIAN_POINT ( 'NONE',  ( 45.00000000000000000, 0.000000000000000000, 4.999999999999998224 ) ) ;
#69864=CARTESIAN_POINT ( 'NONE',  ( 12.75937500061451502, -5.492252693125287522, -1.008910452111647106E-15 ) ) ;
#69885=CARTESIAN_POINT ( 'NONE',  ( 20.63437500061451857, 5.824947211148865298E-16, -4.756430356249998326 ) ) ;
#69900=EDGE_LOOP ( 'NONE', ( #59445, #52228, #56687, #57042 ) ) ;
#69906=CARTESIAN_POINT ( 'NONE',  ( 9.337500000000002132, -2.886751345948074920, 5.000000000000092371 ) ) ;
#69918=CARTESIAN_POINT ( 'NONE',  ( 20.37187500061451573, 2.746126346562643317, 4.756430356249998326 ) ) ;
#69925=CARTESIAN_POINT ( 'NONE',  ( 23.69999999999999929, 0.000000000000000000, 4.999999999999998224 ) ) ;
#69933=CARTESIAN_POINT ( 'NONE',  ( 18.13125000122903074, 6.123233995736764310E-16, -4.999999999999998224 ) ) ;
#69935=CARTESIAN_POINT ( 'NONE',  ( 7.706250001229031810, -4.330127018922190985, -2.500000000000001332 ) ) ;
#69937=CARTESIAN_POINT ( 'NONE',  ( 16.05937500061451573, 2.746126346562645981, -4.756430356249997438 ) ) ;
#69949=CARTESIAN_POINT ( 'NONE',  ( 10.77187500061451608, 4.119189519843966529, 2.378215178124999607 ) ) ;
#69958=CARTESIAN_POINT ( 'NONE',  ( 19.89375000122903714, -2.886751345948181946, -4.999999999999904077 ) ) ;
#69960=CARTESIAN_POINT ( 'NONE',  ( 27.38437500061451502, 5.492252693125287522, 3.363034840372157021E-16 ) ) ;
#69963=CARTESIAN_POINT ( 'NONE',  ( 7.987500000000000711, -2.886751345948129988, 4.999999999999997335 ) ) ;
#69966=ORIENTED_EDGE ( 'NONE', *, *, #27421, .T. ) ;
#69972=CARTESIAN_POINT ( 'NONE',  ( 26.74687500061451573, -2.746126346562646425, 4.756430356249996549 ) ) ;
#69974=CARTESIAN_POINT ( 'NONE',  ( 9.459375000614517859, 4.119189519843966529, -2.378215178124998275 ) ) ;
#69990=CARTESIAN_POINT ( 'NONE',  ( 21.46875000122903288, 2.886751345948126879, 4.999999999999999112 ) ) ;
#69993=ORIENTED_EDGE ( 'NONE', *, *, #18715, .T. ) ;
#70005=CARTESIAN_POINT ( 'NONE',  ( 18.80625000122903501, 0.000000000000000000, 4.999999999999998224 ) ) ;
#70011=( BOUNDED_CURVE ( )  B_SPLINE_CURVE ( 2, ( #4204, #14900, #21536, #5285, #27831, #42982, #31901 ),
 .UNSPECIFIED., .F., .F. ) 
 B_SPLINE_CURVE_WITH_KNOTS ( ( 3, 2, 2, 3 ),
 ( 0.5899999999999999689, 0.5933333333333333792, 0.5966666666666666785, 0.5999999999999999778 ),
 .UNSPECIFIED. ) 
 CURVE ( )  GEOMETRIC_REPRESENTATION_ITEM ( )  RATIONAL_B_SPLINE_CURVE ( ( 1.000000000000000000, 0.8660254037844387076, 1.000000000000000000, 0.8660254037844387076, 1.000000000000000000, 0.8660254037844387076, 1.000000000000000000 ) ) 
 REPRESENTATION_ITEM ( '' )  );
#70023=CARTESIAN_POINT ( 'NONE',  ( 16.55625000122903145, 0.000000000000000000, 4.999999999999998224 ) ) ;
#70031=CARTESIAN_POINT ( 'NONE',  ( 7.303125000614516082, 0.000000000000000000, 4.999999999999998224 ) ) ;
#70034=ORIENTED_EDGE ( 'NONE', *, *, #64274, .T. ) ;
#70038=CARTESIAN_POINT ( 'NONE',  ( 25.87500000000000000, 4.330127018922191873, 2.499999999999999556 ) ) ;
#70041=CARTESIAN_POINT ( 'NONE',  ( 16.05937500061451573, 2.746126346562645981, -4.756430356249997438 ) ) ;
#70057=DIRECTION ( 'NONE',  ( -1.000000000000000000, -0.000000000000000000, -0.000000000000000000 ) ) ;
#70060=CARTESIAN_POINT ( 'NONE',  ( 17.55937500061451573, 4.119189519843966529, -2.378215178124998275 ) ) ;
#70077=CARTESIAN_POINT ( 'NONE',  ( 27.28125000122902932, 4.330127018922191873, 2.499999999999999556 ) ) ;
#70079=CARTESIAN_POINT ( 'NONE',  ( 8.550000000000002487, -4.330127018922190985, -2.500000000000001332 ) ) ;
#70081=CARTESIAN_POINT ( 'NONE',  ( 14.81250000000000178, -5.773502691896255534, -1.060575238724906372E-15 ) ) ;
#70103=FACE_OUTER_BOUND ( 'NONE', #73099, .T. ) ;
#70104=CARTESIAN_POINT ( 'NONE',  ( 29.28749999999999787, -2.886751345948125991, -5.000000000000000000 ) ) ;
#70106=CARTESIAN_POINT ( 'NONE',  ( 20.38125000122903430, 6.123233995736764310E-16, -4.999999999999998224 ) ) ;
#70110=CARTESIAN_POINT ( 'NONE',  ( 11.81250000000000000, 2.886751345948129099, -4.999999999999997335 ) ) ;
#70113=CARTESIAN_POINT ( 'NONE',  ( 10.03125000122903288, 6.123233995736764310E-16, -4.999999999999998224 ) ) ;
#70122=CARTESIAN_POINT ( 'NONE',  ( 16.02187500061451431, 5.824947211148865298E-16, -4.756430356249998326 ) ) ;
#70125=CARTESIAN_POINT ( 'NONE',  ( 24.15937500061451360, 2.746126346562645981, -4.756430356249997438 ) ) ;
#70141=CARTESIAN_POINT ( 'NONE',  ( 25.13437500061451502, 5.824947211148865298E-16, -4.756430356249998326 ) ) ;
#70144=CARTESIAN_POINT ( 'NONE',  ( 25.12499999999999645, -4.330127018922194537, 2.499999999999995559 ) ) ;
#70145=CYLINDRICAL_SURFACE ( 'NONE', #37382, 4.999999999999998224 ) ;
#70155=AXIS2_PLACEMENT_3D ( 'NONE', #37679, #55773, #44701 ) ;
#70163=CARTESIAN_POINT ( 'NONE',  ( 13.13437500061451857, 4.119189519843966529, 2.378215178124999607 ) ) ;
#70188=ADVANCED_FACE ( 'NONE', ( #50064 ), #61860, .T. ) ;
#70191=CARTESIAN_POINT ( 'NONE',  ( 14.78437500061451715, 5.824947211148865298E-16, -4.756430356249998326 ) ) ;
#70199=CARTESIAN_POINT ( 'NONE',  ( 15.52500000000000036, 4.330127018922191873, 2.499999999999999556 ) ) ;
#70204=CARTESIAN_POINT ( 'NONE',  ( 22.02187500061451431, 4.119189519843966529, 2.378215178124999607 ) ) ;
#70211=( BOUNDED_CURVE ( )  B_SPLINE_CURVE ( 2, ( #48430, #64307, #41425, #53594, #8528, #42149, #63941 ),
 .UNSPECIFIED., .F., .F. ) 
 B_SPLINE_CURVE_WITH_KNOTS ( ( 3, 2, 2, 3 ),
 ( 0.8699999999999999956, 0.8733333333333332948, 0.8766666666666667052, 0.8800000000000000044 ),
 .UNSPECIFIED. ) 
 CURVE ( )  GEOMETRIC_REPRESENTATION_ITEM ( )  RATIONAL_B_SPLINE_CURVE ( ( 1.000000000000000000, 0.8660254037844387076, 1.000000000000000000, 0.8660254037844387076, 1.000000000000000000, 0.8660254037844387076, 1.000000000000000000 ) ) 
 REPRESENTATION_ITEM ( '' )  );
#70213=CARTESIAN_POINT ( 'NONE',  ( 21.64687500061451431, 0.000000000000000000, 4.756430356249998326 ) ) ;
#70215=CARTESIAN_POINT ( 'NONE',  ( 9.534375000614517148, -2.746126346562646425, 4.756430356249996549 ) ) ;
#70226=CARTESIAN_POINT ( 'NONE',  ( 8.409375000614517148, 2.746126346562645981, -4.756430356249997438 ) ) ;
#70238=ADVANCED_FACE ( 'NONE', ( #10535 ), #4639, .T. ) ;
#70248=CARTESIAN_POINT ( 'NONE',  ( 14.11875000122903323, 2.886751345948073588, -5.000000000000094147 ) ) ;
#70251=CARTESIAN_POINT ( 'NONE',  ( 20.22187500061451715, 2.746126346562645981, -4.756430356249997438 ) ) ;
#70286=CARTESIAN_POINT ( 'NONE',  ( 21.60937500061451644, 4.119189519843966529, -2.378215178124998275 ) ) ;
#70293=CARTESIAN_POINT ( 'NONE',  ( 23.40000000000000213, -4.330127018922190985, -2.500000000000001332 ) ) ;
#70294=AXIS2_PLACEMENT_3D ( 'NONE', #41471, #17824, #34834 ) ;
#70296=CARTESIAN_POINT ( 'NONE',  ( 9.150000000000002132, 4.330127018922192761, -2.499999999999997780 ) ) ;
#70303=CARTESIAN_POINT ( 'NONE',  ( 8.156250001229034652, -4.330127018922190985, -2.500000000000001332 ) ) ;
#70305=CARTESIAN_POINT ( 'NONE',  ( 16.35937500061451644, -5.492252693125287522, -1.008910452111647106E-15 ) ) ;
#70315=CARTESIAN_POINT ( 'NONE',  ( 7.359375000614517326, -5.492252693125287522, -1.008910452111647106E-15 ) ) ;
#70325=CARTESIAN_POINT ( 'NONE',  ( 29.18437500061451217, 5.492252693125287522, 3.363034840372157021E-16 ) ) ;
#70329=CARTESIAN_POINT ( 'NONE',  ( 7.575000000000001954, -4.330127018922194537, 2.499999999999995559 ) ) ;
#70336=CARTESIAN_POINT ( 'NONE',  ( 25.62187500061451928, 2.746126346562645981, -4.756430356249997438 ) ) ;
#70338=CARTESIAN_POINT ( 'NONE',  ( 11.44687500061451857, -2.746126346562646425, 4.756430356249996549 ) ) ;
#70340=EDGE_CURVE ( 'NONE', #55366, #26340, #23126, .T. ) ;
#70347=CYLINDRICAL_SURFACE ( 'NONE', #39574, 4.999999999999998224 ) ;
#70357=CARTESIAN_POINT ( 'NONE',  ( 20.53125000122903288, 4.330127018922191873, 2.499999999999999556 ) ) ;
#70360=ORIENTED_EDGE ( 'NONE', *, *, #29725, .F. ) ;
#70372=CARTESIAN_POINT ( 'NONE',  ( 27.60937500061451644, 0.000000000000000000, 4.756430356249998326 ) ) ;
#70383=EDGE_CURVE ( 'NONE', #42390, #10555, #24510, .T. ) ;
#70392=CARTESIAN_POINT ( 'NONE',  ( 11.04375000122903216, 5.773502691896255534, 3.535250795749688401E-16 ) ) ;
#70399=CARTESIAN_POINT ( 'NONE',  ( 28.12499999999999645, 4.330127018922191873, 2.499999999999999556 ) ) ;
#70409=CARTESIAN_POINT ( 'NONE',  ( 25.76249999999999218, 2.886751345948087355, -5.000000000000071054 ) ) ;
#70412=CARTESIAN_POINT ( 'NONE',  ( 15.94687500061451502, -4.119189519843965641, -2.378215178125001383 ) ) ;
#70420=CARTESIAN_POINT ( 'NONE',  ( 28.87499999999999645, 6.123233995736764310E-16, -4.999999999999998224 ) ) ;
#70427=CARTESIAN_POINT ( 'NONE',  ( 15.20625000122903181, 0.000000000000000000, 4.999999999999998224 ) ) ;
#70432=CARTESIAN_POINT ( 'NONE',  ( 17.85937500061451999, -4.119189519843965641, -2.378215178125001383 ) ) ;
#70443=VERTEX_POINT ( 'NONE', #69588 ) ;
#70450=CARTESIAN_POINT ( 'NONE',  ( 27.46875000122903288, -5.773502691896255534, -1.060575238724906372E-15 ) ) ;
#70454=CARTESIAN_POINT ( 'NONE',  ( 8.212500000000000355, 2.886751345948129099, -4.999999999999997335 ) ) ;
#70463=EDGE_LOOP ( 'NONE', ( #44395, #41423, #53229, #67626 ) ) ;
#70465=DIRECTION ( 'NONE',  ( -1.000000000000000000, -0.000000000000000000, -0.000000000000000000 ) ) ;
#70474=CARTESIAN_POINT ( 'NONE',  ( 17.60625000122903572, -4.330127018922190985, -2.500000000000001332 ) ) ;
#70475=CARTESIAN_POINT ( 'NONE',  ( 7.621875000614519280, 2.746126346562645981, -4.756430356249997438 ) ) ;
#70477=CARTESIAN_POINT ( 'NONE',  ( 26.68125000122903145, 6.123233995736764310E-16, -4.999999999999998224 ) ) ;
#70481=DIRECTION ( 'NONE',  ( -1.000000000000000000, -0.000000000000000000, -0.000000000000000000 ) ) ;
#70493=CARTESIAN_POINT ( 'NONE',  ( 14.67187500061451644, 5.824947211148865298E-16, -4.756430356249998326 ) ) ;
#70496=CARTESIAN_POINT ( 'NONE',  ( 24.08437500061451075, -2.746126346562642428, -4.756430356249999214 ) ) ;
#70506=CARTESIAN_POINT ( 'NONE',  ( 11.96250000000000213, 2.886751345948126879, 4.999999999999999112 ) ) ;
#70514=CARTESIAN_POINT ( 'NONE',  ( 25.84687500061451360, -2.746126346562646425, 4.756430356249996549 ) ) ;
#70535=CARTESIAN_POINT ( 'NONE',  ( 11.93437500061451573, -4.119189519843968306, 2.378215178124996054 ) ) ;
#70551=CARTESIAN_POINT ( 'NONE',  ( 16.16250000000000142, -5.773502691896255534, -1.060575238724906372E-15 ) ) ;
#70563=CARTESIAN_POINT ( 'NONE',  ( 13.62187500061451750, 2.746126346562643317, 4.756430356249998326 ) ) ;
#70570=CARTESIAN_POINT ( 'NONE',  ( 14.73749999999999893, -2.886751345948129988, 4.999999999999997335 ) ) ;
#70572=CARTESIAN_POINT ( 'NONE',  ( 16.91250000000000142, 2.886751345948182834, 4.999999999999902300 ) ) ;
#70573=CARTESIAN_POINT ( 'NONE',  ( 24.78750000000000142, -2.886751345948126435, -5.000000000000000000 ) ) ;
#70575=ORIENTED_EDGE ( 'NONE', *, *, #14684, .T. ) ;
#70578=LINE ( 'NONE', #42139, #61141 ) ;
#70581=CARTESIAN_POINT ( 'NONE',  ( 22.39687500061451431, 4.119189519843966529, -2.378215178124998275 ) ) ;
#70583=CARTESIAN_POINT ( 'NONE',  ( 9.271875000614517859, 5.824947211148865298E-16, -4.756430356249998326 ) ) ;
#70591=CARTESIAN_POINT ( 'NONE',  ( 8.868750001229031454, 2.886751345948182834, 4.999999999999902300 ) ) ;
#70593=CARTESIAN_POINT ( 'NONE',  ( 9.534375000614517148, -2.746126346562646425, 4.756430356249996549 ) ) ;
#70616=CARTESIAN_POINT ( 'NONE',  ( 19.02187500061451786, 2.746126346562643317, 4.756430356249998326 ) ) ;
#70646=CARTESIAN_POINT ( 'NONE',  ( 20.48437500061451289, -4.119189519843968306, 2.378215178124996054 ) ) ;
#70650=( BOUNDED_CURVE ( )  B_SPLINE_CURVE ( 2, ( #20529, #15002, #37539, #55632, #55995, #62260, #56708 ),
 .UNSPECIFIED., .F., .F. ) 
 B_SPLINE_CURVE_WITH_KNOTS ( ( 3, 2, 2, 3 ),
 ( 0.9300000000000001599, 0.9333333333333334592, 0.9366666666666668695, 0.9400000000000001688 ),
 .UNSPECIFIED. ) 
 CURVE ( )  GEOMETRIC_REPRESENTATION_ITEM ( )  RATIONAL_B_SPLINE_CURVE ( ( 0.9999999999999955591, 0.8660254037844431485, 1.000000000000000000, 0.8660254037844387076, 1.000000000000000000, 0.8660254037844298258, 1.000000000000008882 ) ) 
 REPRESENTATION_ITEM ( '' )  );
#70653=CARTESIAN_POINT ( 'NONE',  ( 21.52499999999999858, -4.330127018922194537, 2.499999999999995559 ) ) ;
#70658=DIRECTION ( 'NONE',  ( -1.000000000000000000, -0.000000000000000000, -0.000000000000000000 ) ) ;
#70659=CARTESIAN_POINT ( 'NONE',  ( 19.55625000122903145, 4.330127018922192761, -2.499999999999997780 ) ) ;
#70663=CARTESIAN_POINT ( 'NONE',  ( 7.218750001229033764, -5.773502691896255534, -1.060575238724906372E-15 ) ) ;
#70665=CARTESIAN_POINT ( 'NONE',  ( 17.03437500061451715, 5.492252693125287522, 3.363034840372157021E-16 ) ) ;
#70668=ORIENTED_EDGE ( 'NONE', *, *, #53326, .T. ) ;
#70681=ORIENTED_EDGE ( 'NONE', *, *, #38932, .F. ) ;
#70687=CARTESIAN_POINT ( 'NONE',  ( 28.50937500061451857, -5.492252693125287522, -1.008910452111647106E-15 ) ) ;
#70698=CARTESIAN_POINT ( 'NONE',  ( 26.14687500061451431, 5.492252693125287522, 3.363034840372157021E-16 ) ) ;
#70700=CARTESIAN_POINT ( 'NONE',  ( 9.759375000614516793, -4.119189519843965641, -2.378215178125001383 ) ) ;
#70709=DIRECTION ( 'NONE',  ( 1.000000000000000000, -0.000000000000000000, -0.000000000000000000 ) ) ;
#70717=CARTESIAN_POINT ( 'NONE',  ( 21.69375000122903430, -2.886751345948125991, -5.000000000000000000 ) ) ;
#70725=CARTESIAN_POINT ( 'NONE',  ( 23.19375000122903074, 5.773502691896255534, 3.535250795749688401E-16 ) ) ;
#70732=CARTESIAN_POINT ( 'NONE',  ( 27.38437500061451857, 5.824947211148865298E-16, -4.756430356249998326 ) ) ;
#70747=EDGE_CURVE ( 'NONE', #15624, #10453, #48473, .T. ) ;
#70758=DIRECTION ( 'NONE',  ( -1.000000000000000000, -0.000000000000000000, -0.000000000000000000 ) ) ;
#70761=CARTESIAN_POINT ( 'NONE',  ( 28.16250000000000142, 2.886751345948119774, 5.000000000000010658 ) ) ;
#70772=CARTESIAN_POINT ( 'NONE',  ( 16.35937500061451644, -5.492252693125287522, -1.008910452111647106E-15 ) ) ;
#70777=DIRECTION ( 'NONE',  ( -1.000000000000000000, -0.000000000000000000, -0.000000000000000000 ) ) ;
#70789=CARTESIAN_POINT ( 'NONE',  ( 9.806250001229033231, 0.000000000000000000, 4.999999999999998224 ) ) ;
#70792=CARTESIAN_POINT ( 'NONE',  ( 27.01875000122903359, -5.773502691896255534, -1.060575238724906372E-15 ) ) ;
#70793=CARTESIAN_POINT ( 'NONE',  ( 18.79687500061451644, -2.746126346562642428, -4.756430356249999214 ) ) ;
#70803=FACE_OUTER_BOUND ( 'NONE', #23571, .T. ) ;
#70804=EDGE_LOOP ( 'NONE', ( #28946, #37061 ) ) ;
#70807=CARTESIAN_POINT ( 'NONE',  ( 45.00000000000000000, 0.000000000000000000, 0.000000000000000000 ) ) ;
#70811=CARTESIAN_POINT ( 'NONE',  ( 28.51875000122903359, 2.886751345948129099, -4.999999999999998224 ) ) ;
#70813=CARTESIAN_POINT ( 'NONE',  ( 45.00000000000000000, 0.000000000000000000, 0.000000000000000000 ) ) ;
#70836=CARTESIAN_POINT ( 'NONE',  ( 7.734375000614517326, 4.119189519843966529, 2.378215178124999607 ) ) ;
#70857=CARTESIAN_POINT ( 'NONE',  ( 15.38437500061451679, -2.746126346562646425, 4.756430356249996549 ) ) ;
#70858=ORIENTED_EDGE ( 'NONE', *, *, #22395, .F. ) ;
#70861=CARTESIAN_POINT ( 'NONE',  ( 23.52187500061451431, -4.119189519843968306, 2.378215178124996054 ) ) ;
#70870=CARTESIAN_POINT ( 'NONE',  ( 23.28750000000000142, -2.886751345948130876, 4.999999999999996447 ) ) ;
#70871=CARTESIAN_POINT ( 'NONE',  ( 13.31250000000000178, 2.886751345948126879, 4.999999999999999112 ) ) ;
#70878=CARTESIAN_POINT ( 'NONE',  ( 24.64687500061451431, -2.746126346562642428, -4.756430356249999214 ) ) ;
#70900=CARTESIAN_POINT ( 'NONE',  ( 13.20937500061451786, 0.000000000000000000, 4.756430356249998326 ) ) ;
#70926=ORIENTED_EDGE ( 'NONE', *, *, #8865, .T. ) ;
#70929=CARTESIAN_POINT ( 'NONE',  ( 13.99687500061451928, 5.492252693125287522, 3.363034840372157021E-16 ) ) ;
#70938=CARTESIAN_POINT ( 'NONE',  ( 14.36249999999999893, -5.773502691896255534, -1.060575238724906372E-15 ) ) ;
#70950=CARTESIAN_POINT ( 'NONE',  ( 23.33437500061451786, 5.492252693125287522, 3.363034840372157021E-16 ) ) ;
#70952=CARTESIAN_POINT ( 'NONE',  ( 9.234375000614514661, -2.746126346562641984, -4.756430356249999214 ) ) ;
#70962=CARTESIAN_POINT ( 'NONE',  ( 10.43437500061451395, -2.746126346562646425, 4.756430356249996549 ) ) ;
#70984=CARTESIAN_POINT ( 'NONE',  ( 18.72187500061451360, -5.492252693125287522, -1.008910452111647106E-15 ) ) ;
#70996=ORIENTED_EDGE ( 'NONE', *, *, #26195, .F. ) ;
#70997=CARTESIAN_POINT ( 'NONE',  ( 45.00000000000000000, 6.123233995736764310E-16, -4.999999999999998224 ) ) ;
#71011=ORIENTED_EDGE ( 'NONE', *, *, #35290, .T. ) ;
#71015=CARTESIAN_POINT ( 'NONE',  ( 20.74687500061451573, 5.492252693125287522, 3.363034840372157021E-16 ) ) ;
#71019=EDGE_CURVE ( 'NONE', #31243, #44627, #72252, .T. ) ;
#71022=CARTESIAN_POINT ( 'NONE',  ( 21.26249999999999574, 2.886751345948129099, -4.999999999999998224 ) ) ;
#71035=CARTESIAN_POINT ( 'NONE',  ( 29.59687500061451360, 4.119189519843966529, -2.378215178124998275 ) ) ;
#71037=CARTESIAN_POINT ( 'NONE',  ( 16.80937500061451573, -5.492252693125287522, -1.008910452111647106E-15 ) ) ;
#71047=CARTESIAN_POINT ( 'NONE',  ( 7.396875000614516082, -4.119189519843965641, -2.378215178125001383 ) ) ;
#71062=CARTESIAN_POINT ( 'NONE',  ( 8.925000000000002487, -4.330127018922194537, 2.499999999999995559 ) ) ;
#71063=FACE_OUTER_BOUND ( 'NONE', #27755, .T. ) ;
#71069=CARTESIAN_POINT ( 'NONE',  ( 27.75937500061451502, -4.119189519843965641, -2.378215178125001383 ) ) ;
#71071=CARTESIAN_POINT ( 'NONE',  ( 7.359375000614516438, 0.000000000000000000, 4.756430356249998326 ) ) ;
#71087=CARTESIAN_POINT ( 'NONE',  ( 22.03125000122903288, -4.330127018922194537, 2.499999999999995559 ) ) ;
#71090=ORIENTED_EDGE ( 'NONE', *, *, #19403, .F. ) ;
#71095=CARTESIAN_POINT ( 'NONE',  ( 7.931250001229031454, 4.330127018922191873, 2.499999999999999556 ) ) ;
#71104=CARTESIAN_POINT ( 'NONE',  ( 28.35937500061451289, 4.119189519843966529, -2.378215178124998275 ) ) ;
#71112=CARTESIAN_POINT ( 'NONE',  ( 21.95625000122903003, 0.000000000000000000, 4.999999999999998224 ) ) ;
#71121=CARTESIAN_POINT ( 'NONE',  ( 16.51875000122903003, 2.886751345948182834, 4.999999999999902300 ) ) ;
#71135=VERTEX_POINT ( 'NONE', #60054 ) ;
#71139=CARTESIAN_POINT ( 'NONE',  ( 15.19687500061451502, 4.119189519843966529, -2.378215178124998275 ) ) ;
#71143=CARTESIAN_POINT ( 'NONE',  ( 45.00000000000000000, 6.123233995736764310E-16, -4.999999999999998224 ) ) ;
#71150=DIRECTION ( 'NONE',  ( -1.000000000000000000, -0.000000000000000000, -0.000000000000000000 ) ) ;
#71158=CARTESIAN_POINT ( 'NONE',  ( 16.80937500061451573, 0.000000000000000000, 4.756430356249998326 ) ) ;
#71172=CARTESIAN_POINT ( 'NONE',  ( 21.50625000122903074, 0.000000000000000000, 4.999999999999998224 ) ) ;
#71176=CARTESIAN_POINT ( 'NONE',  ( 28.78125000122903288, -4.330127018922194537, 2.499999999999995559 ) ) ;
#71178=CYLINDRICAL_SURFACE ( 'NONE', #45521, 4.999999999999998224 ) ;
#71187=ORIENTED_EDGE ( 'NONE', *, *, #32834, .T. ) ;
#71191=EDGE_CURVE ( 'NONE', #38944, #1656, #50961, .T. ) ;
#71201=CARTESIAN_POINT ( 'NONE',  ( 27.18750000000000000, 5.773502691896255534, 3.535250795749688894E-16 ) ) ;
#71203=CARTESIAN_POINT ( 'NONE',  ( 26.49375000122903145, -2.886751345948130876, 4.999999999999996447 ) ) ;
#71219=CARTESIAN_POINT ( 'NONE',  ( 12.72187500061451537, -4.119189519843968306, 2.378215178124996054 ) ) ;
#71223=CARTESIAN_POINT ( 'NONE',  ( 24.30937500061451573, 2.746126346562643317, 4.756430356249998326 ) ) ;
#71232=CARTESIAN_POINT ( 'NONE',  ( 45.00000000000000000, 0.000000000000000000, 0.000000000000000000 ) ) ;
#71233=CARTESIAN_POINT ( 'NONE',  ( 12.18750000000000000, -2.886751345948125991, -5.000000000000000000 ) ) ;
#71240=CARTESIAN_POINT ( 'NONE',  ( 24.87187500061451573, 2.746126346562643317, 4.756430356249998326 ) ) ;
#71243=( LENGTH_UNIT ( ) NAMED_UNIT ( * ) SI_UNIT ( .MILLI., .METRE. ) );
#71261=CARTESIAN_POINT ( 'NONE',  ( 11.03437500061451715, -4.119189519843968306, 2.378215178124996054 ) ) ;
#71276=ORIENTED_EDGE ( 'NONE', *, *, #60032, .F. ) ;
#71290=CARTESIAN_POINT ( 'NONE',  ( 14.52187500061451608, 2.746126346562643317, 4.756430356249998326 ) ) ;
#71299=CARTESIAN_POINT ( 'NONE',  ( 14.62500000000000000, 4.330127018922191873, 2.499999999999999556 ) ) ;
#71313=CARTESIAN_POINT ( 'NONE',  ( 22.84687500061451360, 4.119189519843966529, -2.378215178124998275 ) ) ;
#71329=CARTESIAN_POINT ( 'NONE',  ( 10.35937500061451644, 2.746126346562643317, 4.756430356249998326 ) ) ;
#71335=CARTESIAN_POINT ( 'NONE',  ( 23.02499999999999858, 6.123233995736764310E-16, -4.999999999999998224 ) ) ;
#71338=( BOUNDED_CURVE ( )  B_SPLINE_CURVE ( 2, ( #3959, #14292, #54557, #26855, #49387, #48653, #37193 ),
 .UNSPECIFIED., .F., .F. ) 
 B_SPLINE_CURVE_WITH_KNOTS ( ( 3, 2, 2, 3 ),
 ( 0.1200000000000000788, 0.1233333333333334059, 0.1266666666666667329, 0.1300000000000000322 ),
 .UNSPECIFIED. ) 
 CURVE ( )  GEOMETRIC_REPRESENTATION_ITEM ( )  RATIONAL_B_SPLINE_CURVE ( ( 0.9999999999999966693, 0.8660254037844420383, 1.000000000000000000, 0.8660254037844387076, 1.000000000000000000, 0.8660254037844375974, 1.000000000000001110 ) ) 
 REPRESENTATION_ITEM ( '' )  );
#71351=EDGE_CURVE ( 'NONE', #23511, #16810, #3290, .T. ) ;
#71353=CARTESIAN_POINT ( 'NONE',  ( 17.67187500061451999, 2.746126346562643317, 4.756430356249998326 ) ) ;
#71385=VECTOR ( 'NONE', #69266, 1000.000000000000000 ) ;
#71387=CARTESIAN_POINT ( 'NONE',  ( 22.28437500061451715, -4.119189519843968306, 2.378215178124996054 ) ) ;
#71394=CARTESIAN_POINT ( 'NONE',  ( 22.64999999999999858, 4.330127018922192761, -2.499999999999997780 ) ) ;
#71396=CARTESIAN_POINT ( 'NONE',  ( 22.80000000000000071, 0.000000000000000000, 4.999999999999998224 ) ) ;
#71404=CARTESIAN_POINT ( 'NONE',  ( 29.44687500061451146, -4.119189519843965641, -2.378215178125001383 ) ) ;
#71406=CARTESIAN_POINT ( 'NONE',  ( 14.33437500061451608, 5.492252693125287522, 3.363034840372157021E-16 ) ) ;
#71416=CARTESIAN_POINT ( 'NONE',  ( 8.259375000614515017, -5.492252693125287522, -1.008910452111647106E-15 ) ) ;
#71421=ORIENTED_EDGE ( 'NONE', *, *, #40580, .F. ) ;
#71436=EDGE_CURVE ( 'NONE', #69475, #18169, #17933, .T. ) ;
#71440=CARTESIAN_POINT ( 'NONE',  ( 27.15937500061451360, 0.000000000000000000, 4.756430356249998326 ) ) ;
#71442=CARTESIAN_POINT ( 'NONE',  ( 8.559375000614515727, 4.119189519843966529, -2.378215178124998275 ) ) ;
#71451=ADVANCED_FACE ( 'NONE', ( #29276 ), #64332, .T. ) ;
#71460=CARTESIAN_POINT ( 'NONE',  ( 18.76875000122903359, 2.886751345948126879, 4.999999999999999112 ) ) ;
#71468=DIRECTION ( 'NONE',  ( -1.000000000000000000, -0.000000000000000000, -0.000000000000000000 ) ) ;
#71476=CARTESIAN_POINT ( 'NONE',  ( 28.05937500061451573, 0.000000000000000000, 4.756430356249998326 ) ) ;
#71498=ORIENTED_EDGE ( 'NONE', *, *, #15666, .T. ) ;
#71509=VERTEX_POINT ( 'NONE', #24080 ) ;
#71510=CARTESIAN_POINT ( 'NONE',  ( 19.01249999999999929, 2.886751345948073588, -5.000000000000094147 ) ) ;
#71513=CARTESIAN_POINT ( 'NONE',  ( 14.18437500061451573, -2.746126346562642428, -4.756430356249999214 ) ) ;
#71528=CARTESIAN_POINT ( 'NONE',  ( 9.543750001229033941, -2.886751345948126435, -5.000000000000000000 ) ) ;
#71529=CARTESIAN_POINT ( 'NONE',  ( 14.02499999999999858, 6.123233995736764310E-16, -4.999999999999998224 ) ) ;
#71533=CARTESIAN_POINT ( 'NONE',  ( 15.94687500061451502, -2.746126346562646425, 4.756430356249996549 ) ) ;
#71543=EDGE_CURVE ( 'NONE', #32563, #58840, #63250, .T. ) ;
#71551=CARTESIAN_POINT ( 'NONE',  ( 27.54375000122903216, -2.886751345948125991, -5.000000000000000000 ) ) ;
#71555=CARTESIAN_POINT ( 'NONE',  ( 8.250000000000000000, 4.330127018922192761, -2.499999999999997780 ) ) ;
#71562=ORIENTED_EDGE ( 'NONE', *, *, #27156, .F. ) ;
#71584=CARTESIAN_POINT ( 'NONE',  ( 9.356250001229033941, 0.000000000000000000, 4.999999999999998224 ) ) ;
#71595=ORIENTED_EDGE ( 'NONE', *, *, #14306, .F. ) ;
#71598=CARTESIAN_POINT ( 'NONE',  ( 20.29687500061451289, 0.000000000000000000, 4.756430356249998326 ) ) ;
#71606=EDGE_CURVE ( 'NONE', #61419, #8461, #27886, .T. ) ;
#71609=CARTESIAN_POINT ( 'NONE',  ( 13.64999999999999858, 4.330127018922192761, -2.499999999999997780 ) ) ;
#71610=AXIS2_PLACEMENT_3D ( 'NONE', #52762, #25040, #63115 ) ;
#71617=CARTESIAN_POINT ( 'NONE',  ( 23.37187500061451573, 2.746126346562645981, -4.756430356249997438 ) ) ;
#71621=DIRECTION ( 'NONE',  ( 0.000000000000000000, 0.000000000000000000, 1.000000000000000000 ) ) ;
#71628=EDGE_LOOP ( 'NONE', ( #50061, #65338, #64240, #69600 ) ) ;
#71639=CARTESIAN_POINT ( 'NONE',  ( 10.24687500061451573, -2.746126346562641984, -4.756430356249999214 ) ) ;
#71650=ORIENTED_EDGE ( 'NONE', *, *, #13859, .F. ) ;
#71661=ORIENTED_EDGE ( 'NONE', *, *, #70747, .T. ) ;
#71664=CARTESIAN_POINT ( 'NONE',  ( 12.12187500061451573, 2.746126346562645981, -4.756430356249997438 ) ) ;
#71665=CYLINDRICAL_SURFACE ( 'NONE', #21731, 4.999999999999998224 ) ;
#71667=CARTESIAN_POINT ( 'NONE',  ( 13.55625000122903323, -4.330127018922190985, -2.500000000000001332 ) ) ;
#71681=CARTESIAN_POINT ( 'NONE',  ( 20.08125000122903359, 4.330127018922191873, 2.499999999999999556 ) ) ;
#71683=( BOUNDED_CURVE ( )  B_SPLINE_CURVE ( 2, ( #36381, #53007, #71095, #52644, #2767, #13842, #13110 ),
 .UNSPECIFIED., .F., .F. ) 
 B_SPLINE_CURVE_WITH_KNOTS ( ( 3, 2, 2, 3 ),
 ( 0.9599999999999999645, 0.9633333333333333748, 0.9666666666666666741, 0.9699999999999999734 ),
 .UNSPECIFIED. ) 
 CURVE ( )  GEOMETRIC_REPRESENTATION_ITEM ( )  RATIONAL_B_SPLINE_CURVE ( ( 1.000000000000000000, 0.8660254037844387076, 1.000000000000000000, 0.8660254037844387076, 1.000000000000000000, 0.8660254037844387076, 1.000000000000000000 ) ) 
 REPRESENTATION_ITEM ( '' )  );
#71687=CARTESIAN_POINT ( 'NONE',  ( 19.20937500061451786, 2.746126346562645981, -4.756430356249997438 ) ) ;
#71690=CARTESIAN_POINT ( 'NONE',  ( 14.79375000122903216, -2.886751345948129988, 4.999999999999997335 ) ) ;
#71704=CARTESIAN_POINT ( 'NONE',  ( 8.709375000614516082, -5.492252693125287522, -1.008910452111647106E-15 ) ) ;
#71709=LINE ( 'NONE', #43269, #30121 ) ;
#71727=CARTESIAN_POINT ( 'NONE',  ( 17.70937500061451431, 0.000000000000000000, 4.756430356249998326 ) ) ;
#71746=CARTESIAN_POINT ( 'NONE',  ( 20.45625000122903359, 4.330127018922192761, -2.499999999999997780 ) ) ;
#71756=EDGE_LOOP ( 'NONE', ( #10119, #39435, #12184, #15842 ) ) ;
#71759=CARTESIAN_POINT ( 'NONE',  ( 19.73437500061451644, 5.824947211148865298E-16, -4.756430356249998326 ) ) ;
#71765=CARTESIAN_POINT ( 'NONE',  ( 22.50000000000000000, -4.330127018922190985, -2.500000000000001332 ) ) ;
#71768=CARTESIAN_POINT ( 'NONE',  ( 14.45625000122903359, -4.330127018922190985, -2.500000000000001332 ) ) ;
#71776=CARTESIAN_POINT ( 'NONE',  ( 27.94687500061451502, 0.000000000000000000, 4.756430356249998326 ) ) ;
#71779=CARTESIAN_POINT ( 'NONE',  ( 13.84687500061451715, 4.119189519843966529, -2.378215178124998275 ) ) ;
#71789=CARTESIAN_POINT ( 'NONE',  ( 8.559375000614515727, 2.746126346562643317, 4.756430356249998326 ) ) ;
#71803=CARTESIAN_POINT ( 'NONE',  ( 10.20000000000000107, 0.000000000000000000, 4.999999999999998224 ) ) ;
#71810=CARTESIAN_POINT ( 'NONE',  ( 24.15937500061451715, -4.119189519843965641, -2.378215178125001383 ) ) ;
#71812=CARTESIAN_POINT ( 'NONE',  ( 7.471875000614519813, -5.492252693125287522, -1.008910452111647106E-15 ) ) ;
#71829=CARTESIAN_POINT ( 'NONE',  ( 17.90625000122903288, 0.000000000000000000, 4.999999999999998224 ) ) ;
#71832=ORIENTED_EDGE ( 'NONE', *, *, #49066, .F. ) ;
#71833=EDGE_CURVE ( 'NONE', #4995, #61022, #40602, .T. ) ;
#71838=CARTESIAN_POINT ( 'NONE',  ( 20.88749999999999929, 5.773502691896255534, 3.535250795749688401E-16 ) ) ;
#71845=CARTESIAN_POINT ( 'NONE',  ( 29.22187500061451715, 2.746126346562645981, -4.756430356249997438 ) ) ;
#71852=CARTESIAN_POINT ( 'NONE',  ( 7.368750001229031454, 2.886751345948018077, -5.000000000000190070 ) ) ;
#71863=CARTESIAN_POINT ( 'NONE',  ( 20.18437500061451217, 5.492252693125287522, 3.363034840372157021E-16 ) ) ;
#71867=CARTESIAN_POINT ( 'NONE',  ( 10.66875000122903216, 2.886751345948126879, 4.999999999999998224 ) ) ;
#71877=ORIENTED_EDGE ( 'NONE', *, *, #62721, .T. ) ;
#71881=CARTESIAN_POINT ( 'NONE',  ( 13.50937500061451679, 2.746126346562643317, 4.756430356249998326 ) ) ;
#71899=CARTESIAN_POINT ( 'NONE',  ( 14.48437500061451821, 4.119189519843966529, 2.378215178124999607 ) ) ;
#71916=CARTESIAN_POINT ( 'NONE',  ( 24.73125000122903216, -4.330127018922194537, 2.499999999999995559 ) ) ;
#71928=CARTESIAN_POINT ( 'NONE',  ( 23.83125000122903359, -4.330127018922194537, 2.499999999999995559 ) ) ;
#71960=( BOUNDED_CURVE ( )  B_SPLINE_CURVE ( 2, ( #22164, #44716, #33608, #56152, #12164, #46154, #45796 ),
 .UNSPECIFIED., .F., .F. ) 
 B_SPLINE_CURVE_WITH_KNOTS ( ( 3, 2, 2, 3 ),
 ( 0.1300000000000000322, 0.1333333333333333592, 0.1366666666666666585, 0.1400000000000000133 ),
 .UNSPECIFIED. ) 
 CURVE ( )  GEOMETRIC_REPRESENTATION_ITEM ( )  RATIONAL_B_SPLINE_CURVE ( ( 0.9999999999999988898, 0.8660254037844398178, 1.000000000000000000, 0.8660254037844387076, 1.000000000000000000, 0.8660254037844387076, 1.000000000000000000 ) ) 
 REPRESENTATION_ITEM ( '' )  );
#71965=CARTESIAN_POINT ( 'NONE',  ( 21.90937500061451715, 2.746126346562645981, -4.756430356249997438 ) ) ;
#71974=CARTESIAN_POINT ( 'NONE',  ( 13.08750000000000036, -2.886751345948125991, -5.000000000000000000 ) ) ;
#71981=CARTESIAN_POINT ( 'NONE',  ( 23.18437500061451573, -4.119189519843968306, 2.378215178124996054 ) ) ;
#71984=CARTESIAN_POINT ( 'NONE',  ( 13.25625000122903074, 4.330127018922192761, -2.499999999999997780 ) ) ;
#71996=CARTESIAN_POINT ( 'NONE',  ( 27.13125000122903430, 6.123233995736764310E-16, -4.999999999999998224 ) ) ;
#72002=CARTESIAN_POINT ( 'NONE',  ( 10.28437500061451715, 5.824947211148865298E-16, -4.756430356249998326 ) ) ;
#72010=VERTEX_POINT ( 'NONE', #21823 ) ;
#72024=CARTESIAN_POINT ( 'NONE',  ( 11.37187500061451750, 2.746126346562643317, 4.756430356249998326 ) ) ;
#72027=EDGE_CURVE ( 'NONE', #1784, #40656, #27022, .T. ) ;
#72034=FACE_OUTER_BOUND ( 'NONE', #24114, .T. ) ;
#72042=CARTESIAN_POINT ( 'NONE',  ( 19.80937500061451217, 2.746126346562643317, 4.756430356249998326 ) ) ;
#72045=CARTESIAN_POINT ( 'NONE',  ( 14.98125000122903216, 6.123233995736764310E-16, -4.999999999999998224 ) ) ;
#72051=CARTESIAN_POINT ( 'NONE',  ( 21.89999999999999858, 0.000000000000000000, 4.999999999999998224 ) ) ;
#72058=CARTESIAN_POINT ( 'NONE',  ( 28.95937500061451431, 0.000000000000000000, 4.756430356249998326 ) ) ;
#72078=CARTESIAN_POINT ( 'NONE',  ( 16.65937500061452070, 4.119189519843966529, -2.378215178124998275 ) ) ;
#72105=VECTOR ( 'NONE', #1101, 1000.000000000000000 ) ;
#72108=EDGE_LOOP ( 'NONE', ( #32117, #40892, #38544, #10134 ) ) ;
#72111=CARTESIAN_POINT ( 'NONE',  ( 18.23437500061451999, -4.119189519843968306, 2.378215178124996054 ) ) ;
#72116=( BOUNDED_CURVE ( )  B_SPLINE_CURVE ( 2, ( #24562, #59631, #43023, #70725, #30110, #25666, #37105 ),
 .UNSPECIFIED., .F., .F. ) 
 B_SPLINE_CURVE_WITH_KNOTS ( ( 3, 2, 2, 3 ),
 ( 0.2800000000000000266, 0.2833333333333333259, 0.2866666666666667362, 0.2900000000000000355 ),
 .UNSPECIFIED. ) 
 CURVE ( )  GEOMETRIC_REPRESENTATION_ITEM ( )  RATIONAL_B_SPLINE_CURVE ( ( 1.000000000000000000, 0.8660254037844387076, 1.000000000000000000, 0.8660254037844387076, 1.000000000000000000, 0.8660254037844364872, 1.000000000000002220 ) ) 
 REPRESENTATION_ITEM ( '' )  );
#72119=CARTESIAN_POINT ( 'NONE',  ( 20.77500000000000213, 6.123233995736764310E-16, -4.999999999999998224 ) ) ;
#72121=CARTESIAN_POINT ( 'NONE',  ( 20.54999999999999716, 0.000000000000000000, 4.999999999999998224 ) ) ;
#72123=CARTESIAN_POINT ( 'NONE',  ( 18.91875000122903216, -5.773502691896255534, -1.060575238724906372E-15 ) ) ;
#72126=CARTESIAN_POINT ( 'NONE',  ( 28.27499999999999858, -4.330127018922194537, 2.499999999999995559 ) ) ;
#72131=CARTESIAN_POINT ( 'NONE',  ( 27.00937500061451502, 2.746126346562643317, 4.756430356249998326 ) ) ;
#72133=CARTESIAN_POINT ( 'NONE',  ( 12.75937500061451502, -5.492252693125287522, -1.008910452111647106E-15 ) ) ;
#72150=VERTEX_POINT ( 'NONE', #10748 ) ;
#72166=( BOUNDED_CURVE ( )  B_SPLINE_CURVE ( 2, ( #31693, #54228, #15415, #37958, #37594, #60478, #32421 ),
 .UNSPECIFIED., .F., .F. ) 
 B_SPLINE_CURVE_WITH_KNOTS ( ( 3, 2, 2, 3 ),
 ( 0.08999999999999996891, 0.09333333333333329596, 0.09666666666666662300, 0.09999999999999995004 ),
 .UNSPECIFIED. ) 
 CURVE ( )  GEOMETRIC_REPRESENTATION_ITEM ( )  RATIONAL_B_SPLINE_CURVE ( ( 1.000000000000001110, 0.8660254037844374864, 1.000000000000000000, 0.8660254037844387076, 1.000000000000000000, 0.8660254037844409281, 0.9999999999999977796 ) ) 
 REPRESENTATION_ITEM ( '' )  );
#72168=CARTESIAN_POINT ( 'NONE',  ( 25.17187500061451644, 2.746126346562645981, -4.756430356249997438 ) ) ;
#72170=CARTESIAN_POINT ( 'NONE',  ( 9.196875000614518569, -2.746126346562646425, 4.756430356249996549 ) ) ;
#72175=ORIENTED_EDGE ( 'NONE', *, *, #64115, .T. ) ;
#72177=CARTESIAN_POINT ( 'NONE',  ( 27.22499999999999787, 4.330127018922191873, 2.499999999999999556 ) ) ;
#72189=CARTESIAN_POINT ( 'NONE',  ( 19.48125000122903216, 6.123233995736764310E-16, -4.999999999999998224 ) ) ;
#72191=CARTESIAN_POINT ( 'NONE',  ( 29.38125000122903074, 6.123233995736764310E-16, -4.999999999999998224 ) ) ;
#72207=CARTESIAN_POINT ( 'NONE',  ( 27.12187500061451573, 2.746126346562643317, 4.756430356249998326 ) ) ;
#72215=CARTESIAN_POINT ( 'NONE',  ( 9.825000000000001066, -4.330127018922194537, 2.499999999999995559 ) ) ;
#72219=CARTESIAN_POINT ( 'NONE',  ( 27.56249999999999645, 2.886751345948164182, -4.999999999999937828 ) ) ;
#72221=CARTESIAN_POINT ( 'NONE',  ( 11.64375000122903003, -2.886751345948129988, 4.999999999999997335 ) ) ;
#72222=CARTESIAN_POINT ( 'NONE',  ( 13.27500000000000213, 4.330127018922191873, 2.499999999999999556 ) ) ;
#72224=CARTESIAN_POINT ( 'NONE',  ( 19.99687500061451217, -4.119189519843965641, -2.378215178125001383 ) ) ;
#72242=CARTESIAN_POINT ( 'NONE',  ( 10.91249999999999964, 2.886751345948018077, -5.000000000000190070 ) ) ;
#72243=CARTESIAN_POINT ( 'NONE',  ( 13.05937500061451573, 2.746126346562643317, 4.756430356249998326 ) ) ;
#72246=CYLINDRICAL_SURFACE ( 'NONE', #5036, 4.999999999999998224 ) ;
#72249=ORIENTED_EDGE ( 'NONE', *, *, #46464, .T. ) ;
#72252=LINE ( 'NONE', #9097, #36859 ) ;
#72259=CARTESIAN_POINT ( 'NONE',  ( 28.99687500061451217, -4.119189519843965641, -2.378215178125001383 ) ) ;
#72260=CARTESIAN_POINT ( 'NONE',  ( 15.38437500061451679, 4.119189519843966529, 2.378215178124999607 ) ) ;
#72268=CARTESIAN_POINT ( 'NONE',  ( 26.39999999999999858, 0.000000000000000000, 4.999999999999998224 ) ) ;
#72278=CARTESIAN_POINT ( 'NONE',  ( 25.74375000122903501, -2.886751345948125991, -5.000000000000000000 ) ) ;
#72290=CARTESIAN_POINT ( 'NONE',  ( 10.29375000122902861, -2.886751345948019409, 5.000000000000189182 ) ) ;
#72319=ADVANCED_FACE ( 'NONE', ( #69363 ), #25746, .T. ) ;
#72321=ORIENTED_EDGE ( 'NONE', *, *, #47314, .F. ) ;
#72324=CARTESIAN_POINT ( 'NONE',  ( 20.97187500061451715, 5.824947211148865298E-16, -4.756430356249998326 ) ) ;
#72331=CARTESIAN_POINT ( 'NONE',  ( 34.99999999999999289, 2.500000000000000444, 3.499999999999999112 ) ) ;
#72333=CARTESIAN_POINT ( 'NONE',  ( 10.12500000000000178, 4.330127018922191873, 2.499999999999999556 ) ) ;
#72339=CARTESIAN_POINT ( 'NONE',  ( 22.17187500061451644, 2.746126346562643317, 4.756430356249998326 ) ) ;
#72361=CARTESIAN_POINT ( 'NONE',  ( 9.609375000614518214, 0.000000000000000000, 4.756430356249998326 ) ) ;
#72365=EDGE_CURVE ( 'NONE', #16786, #50451, #66067, .T. ) ;
#72371=ORIENTED_EDGE ( 'NONE', *, *, #8883, .T. ) ;
#72384=CARTESIAN_POINT ( 'NONE',  ( 12.00937500061451857, -4.119189519843965641, -2.378215178125001383 ) ) ;
#72403=CARTESIAN_POINT ( 'NONE',  ( 20.85937500061451644, -5.492252693125287522, -1.008910452111647106E-15 ) ) ;
#72406=CARTESIAN_POINT ( 'NONE',  ( 14.86875000122903323, -5.773502691896255534, -1.060575238724906372E-15 ) ) ;
#72413=CARTESIAN_POINT ( 'NONE',  ( 21.78750000000000142, 5.773502691896255534, 3.535250795749688401E-16 ) ) ;
#72421=CARTESIAN_POINT ( 'NONE',  ( 7.321875000614517681, -4.119189519843968306, 2.378215178124996054 ) ) ;
#72426=CYLINDRICAL_SURFACE ( 'NONE', #69108, 4.999999999999998224 ) ;
#72442=CARTESIAN_POINT ( 'NONE',  ( 16.92187500061451999, -5.492252693125287522, -1.008910452111647106E-15 ) ) ;
#72475=CARTESIAN_POINT ( 'NONE',  ( 18.34687500061451715, -2.746126346562642428, -4.756430356249999214 ) ) ;
#72481=CARTESIAN_POINT ( 'NONE',  ( 19.76250000000000639, -5.773502691896255534, -1.060575238724906372E-15 ) ) ;
#72484=CARTESIAN_POINT ( 'NONE',  ( 25.84687500061451360, -4.119189519843965641, -2.378215178125001383 ) ) ;
#72485=CARTESIAN_POINT ( 'NONE',  ( 14.38125000122903252, -4.330127018922194537, 2.499999999999995559 ) ) ;
#72490=ADVANCED_FACE ( 'NONE', ( #30912 ), #58247, .T. ) ;
#72492=CARTESIAN_POINT ( 'NONE',  ( 28.35937500061451644, 2.746126346562643317, 4.756430356249998326 ) ) ;
#72494=CARTESIAN_POINT ( 'NONE',  ( 14.29687500061451644, 4.119189519843966529, -2.378215178124998275 ) ) ;
#72508=EDGE_CURVE ( 'NONE', #8461, #16786, #14286, .T. ) ;
#72518=DIRECTION ( 'NONE',  ( 0.000000000000000000, 0.000000000000000000, 1.000000000000000000 ) ) ;
#72520=VERTEX_POINT ( 'NONE', #24638 ) ;
#72523=CARTESIAN_POINT ( 'NONE',  ( 45.00000000000000000, 0.000000000000000000, 4.999999999999998224 ) ) ;
#72530=CARTESIAN_POINT ( 'NONE',  ( 24.34687500061451715, 5.492252693125287522, 3.363034840372157021E-16 ) ) ;
#72532=CARTESIAN_POINT ( 'NONE',  ( 7.696875000614516793, 5.492252693125287522, 3.363034840372157021E-16 ) ) ;
#72542=CARTESIAN_POINT ( 'NONE',  ( 17.34375000122903288, 5.773502691896255534, 3.535250795749688401E-16 ) ) ;
#72550=CARTESIAN_POINT ( 'NONE',  ( 19.29375000122903216, -2.886751345948129988, 4.999999999999997335 ) ) ;
#72566=CARTESIAN_POINT ( 'NONE',  ( 25.50937500061451502, -4.119189519843965641, -2.378215178125001383 ) ) ;
#72572=CARTESIAN_POINT ( 'NONE',  ( 27.29999999999999716, 0.000000000000000000, 4.999999999999998224 ) ) ;
#72573=AXIS2_PLACEMENT_3D ( 'NONE', #30909, #36819, #37183 ) ;
#72575=CARTESIAN_POINT ( 'NONE',  ( 9.750000000000001776, 0.000000000000000000, 4.999999999999998224 ) ) ;
#72580=LINE ( 'NONE', #67415, #26857 ) ;
#72583=CARTESIAN_POINT ( 'NONE',  ( 12.35625000122903394, 4.330127018922192761, -2.499999999999997780 ) ) ;
#72587=CARTESIAN_POINT ( 'NONE',  ( 21.87187500061451573, 5.824947211148865298E-16, -4.756430356249998326 ) ) ;
#72599=CARTESIAN_POINT ( 'NONE',  ( 13.95937500061451608, 2.746126346562643317, 4.756430356249998326 ) ) ;
#72603=( BOUNDED_CURVE ( )  B_SPLINE_CURVE ( 2, ( #59719, #8757, #25381, #26858, #71555, #70454, #20930 ),
 .UNSPECIFIED., .F., .F. ) 
 B_SPLINE_CURVE_WITH_KNOTS ( ( 3, 2, 2, 3 ),
 ( 0.9599999999999999645, 0.9633333333333333748, 0.9666666666666666741, 0.9699999999999999734 ),
 .UNSPECIFIED. ) 
 CURVE ( )  GEOMETRIC_REPRESENTATION_ITEM ( )  RATIONAL_B_SPLINE_CURVE ( ( 1.000000000000000000, 0.8660254037844387076, 1.000000000000000000, 0.8660254037844387076, 1.000000000000000000, 0.8660254037844387076, 1.000000000000000000 ) ) 
 REPRESENTATION_ITEM ( '' )  );
#72612=FACE_OUTER_BOUND ( 'NONE', #55977, .T. ) ;
#72626=CARTESIAN_POINT ( 'NONE',  ( 16.17187500061451644, 2.746126346562645981, -4.756430356249997438 ) ) ;
#72632=CARTESIAN_POINT ( 'NONE',  ( 10.65000000000000036, 0.000000000000000000, 4.999999999999998224 ) ) ;
#72643=CARTESIAN_POINT ( 'NONE',  ( 25.10625000122903216, 0.000000000000000000, 4.999999999999998224 ) ) ;
#72658=CARTESIAN_POINT ( 'NONE',  ( 10.48125000122903216, 6.123233995736764310E-16, -4.999999999999998224 ) ) ;
#72692=CARTESIAN_POINT ( 'NONE',  ( 21.23437500061451644, -2.746126346562646425, 4.756430356249996549 ) ) ;
#72701=CARTESIAN_POINT ( 'NONE',  ( 11.36250000000000071, 2.886751345948129099, -4.999999999999998224 ) ) ;
#72708=CARTESIAN_POINT ( 'NONE',  ( 21.23437500061451644, 4.119189519843966529, 2.378215178124999607 ) ) ;
#72730=CARTESIAN_POINT ( 'NONE',  ( 8.971875000614515372, 2.746126346562645981, -4.756430356249997438 ) ) ;
#72737=ORIENTED_EDGE ( 'NONE', *, *, #66497, .T. ) ;
#72740=DIRECTION ( 'NONE',  ( 0.000000000000000000, 0.000000000000000000, 1.000000000000000000 ) ) ;
#72743=EDGE_CURVE ( 'NONE', #27832, #55926, #12765, .T. ) ;
#72751=CARTESIAN_POINT ( 'NONE',  ( 17.25000000000000000, 4.330127018922192761, -2.499999999999997780 ) ) ;
#72752=CARTESIAN_POINT ( 'NONE',  ( 12.34687500061452070, -2.746126346562646425, 4.756430356249996549 ) ) ;
#72773=CARTESIAN_POINT ( 'NONE',  ( 21.12187500061451217, 4.119189519843966529, 2.378215178124999607 ) ) ;
#72776=CARTESIAN_POINT ( 'NONE',  ( 13.10625000122903394, -4.330127018922190985, -2.500000000000001332 ) ) ;
#72778=CARTESIAN_POINT ( 'NONE',  ( 7.434375000614515727, -2.746126346562641984, -4.756430356249999214 ) ) ;
#72792=CARTESIAN_POINT ( 'NONE',  ( 29.07187500061451502, -5.492252693125287522, -1.008910452111647106E-15 ) ) ;
#72798=CARTESIAN_POINT ( 'NONE',  ( 14.55000000000000071, 4.330127018922192761, -2.499999999999997780 ) ) ;
#72800=DIRECTION ( 'NONE',  ( -1.000000000000000000, -0.000000000000000000, -0.000000000000000000 ) ) ;
#72814=CARTESIAN_POINT ( 'NONE',  ( 16.24687500061451573, 5.492252693125287522, 3.363034840372157021E-16 ) ) ;
#72818=ORIENTED_EDGE ( 'NONE', *, *, #10883, .T. ) ;
#72847=CARTESIAN_POINT ( 'NONE',  ( 18.72187500061451360, -5.492252693125287522, -1.008910452111647106E-15 ) ) ;
#72852=CARTESIAN_POINT ( 'NONE',  ( 19.23749999999999716, -2.886751345948129988, 4.999999999999997335 ) ) ;
#72855=CARTESIAN_POINT ( 'NONE',  ( 21.44999999999999929, 0.000000000000000000, 4.999999999999998224 ) ) ;
#72856=CARTESIAN_POINT ( 'NONE',  ( 25.02187500061451431, 5.824947211148865298E-16, -4.756430356249998326 ) ) ;
#72863=CARTESIAN_POINT ( 'NONE',  ( 28.47187500061451715, -4.119189519843968306, 2.378215178124996054 ) ) ;
#72865=CARTESIAN_POINT ( 'NONE',  ( 13.73437500061451289, -2.746126346562641984, -4.756430356249999214 ) ) ;
#72873=AXIS2_PLACEMENT_3D ( 'NONE', #41292, #1411, #47551 ) ;
#72875=CARTESIAN_POINT ( 'NONE',  ( 18.13125000122903074, 6.123233995736764310E-16, -4.999999999999998224 ) ) ;
#72899=CARTESIAN_POINT ( 'NONE',  ( 23.70937500061451786, -4.119189519843965641, -2.378215178125001383 ) ) ;
#72906=VERTEX_POINT ( 'NONE', #38280 ) ;
#72910=CARTESIAN_POINT ( 'NONE',  ( 7.631250001229033408, -4.330127018922194537, 2.499999999999995559 ) ) ;
#72917=CARTESIAN_POINT ( 'NONE',  ( 18.46875000122902932, -5.773502691896255534, -1.060575238724906372E-15 ) ) ;
#72927=CARTESIAN_POINT ( 'NONE',  ( 20.85000000000000142, 4.330127018922192761, -2.499999999999997780 ) ) ;
#72933=CARTESIAN_POINT ( 'NONE',  ( 24.90937500061451715, 0.000000000000000000, 4.756430356249998326 ) ) ;
#72939=CARTESIAN_POINT ( 'NONE',  ( 25.94999999999999929, 0.000000000000000000, 4.999999999999998224 ) ) ;
#72948=CARTESIAN_POINT ( 'NONE',  ( 12.76875000122903181, 2.886751345948129099, -4.999999999999998224 ) ) ;
#72952=CARTESIAN_POINT ( 'NONE',  ( 19.65937500061451360, 2.746126346562645981, -4.756430356249997438 ) ) ;
#72963=CARTESIAN_POINT ( 'NONE',  ( 14.03437500061451892, -2.746126346562646425, 4.756430356249996549 ) ) ;
#72964=ORIENTED_EDGE ( 'NONE', *, *, #54007, .T. ) ;
#72970=CARTESIAN_POINT ( 'NONE',  ( 21.24375000122903145, -2.886751345948126435, -5.000000000000000000 ) ) ;
#72984=CARTESIAN_POINT ( 'NONE',  ( 13.50000000000000178, -4.330127018922190985, -2.500000000000001332 ) ) ;
#72987=CARTESIAN_POINT ( 'NONE',  ( 14.22187500061451537, -5.492252693125287522, -1.008910452111647106E-15 ) ) ;
#72994=CARTESIAN_POINT ( 'NONE',  ( 10.42500000000000071, 6.123233995736764310E-16, -4.999999999999998224 ) ) ;
#73003=CARTESIAN_POINT ( 'NONE',  ( 45.00000000000000000, 0.000000000000000000, 0.000000000000000000 ) ) ;
#73004=CARTESIAN_POINT ( 'NONE',  ( 26.79375000122903216, 5.773502691896255534, 3.535250795749688894E-16 ) ) ;
#73012=EDGE_CURVE ( 'NONE', #24228, #24506, #489, .T. ) ;
#73029=CYLINDRICAL_SURFACE ( 'NONE', #26425, 4.999999999999998224 ) ;
#73043=EDGE_CURVE ( 'NONE', #53411, #32794, #18370, .T. ) ;
#73049=ORIENTED_EDGE ( 'NONE', *, *, #24709, .T. ) ;
#73052=CARTESIAN_POINT ( 'NONE',  ( 20.48437500061451644, -2.746126346562642428, -4.756430356249999214 ) ) ;
#73056=CARTESIAN_POINT ( 'NONE',  ( 11.32500000000000107, 6.123233995736764310E-16, -4.999999999999998224 ) ) ;
#73063=CARTESIAN_POINT ( 'NONE',  ( 11.47499999999999964, 4.330127018922191873, 2.499999999999999556 ) ) ;
#73069=CARTESIAN_POINT ( 'NONE',  ( 21.60937500061451644, 4.119189519843966529, -2.378215178124998275 ) ) ;
#73086=CARTESIAN_POINT ( 'NONE',  ( 18.52499999999999858, 6.123233995736764310E-16, -4.999999999999998224 ) ) ;
#73091=CARTESIAN_POINT ( 'NONE',  ( 7.884375000614517681, -4.119189519843968306, 2.378215178124996054 ) ) ;
#73099=EDGE_LOOP ( 'NONE', ( #11929, #59178, #27988, #24516 ) ) ;
#73113=CARTESIAN_POINT ( 'NONE',  ( 11.33437500061451608, 4.119189519843966529, 2.378215178124999607 ) ) ;
#73114=CYLINDRICAL_SURFACE ( 'NONE', #50058, 4.999999999999998224 ) ;
#73138=COLOUR_RGB('Sky Blue',0.24,0.69,0.87);
#73139=FILL_AREA_STYLE_COLOUR('',#73138);
#73140=FILL_AREA_STYLE('',(#73139));
#73141=SURFACE_STYLE_FILL_AREA(#73140);
#73142=SURFACE_SIDE_STYLE('',(#73141));
#73143=SURFACE_STYLE_USAGE(.BOTH.,#73142);
#73144=PRESENTATION_STYLE_ASSIGNMENT((#73143));
ENDSEC;
END-ISO-10303-21;
